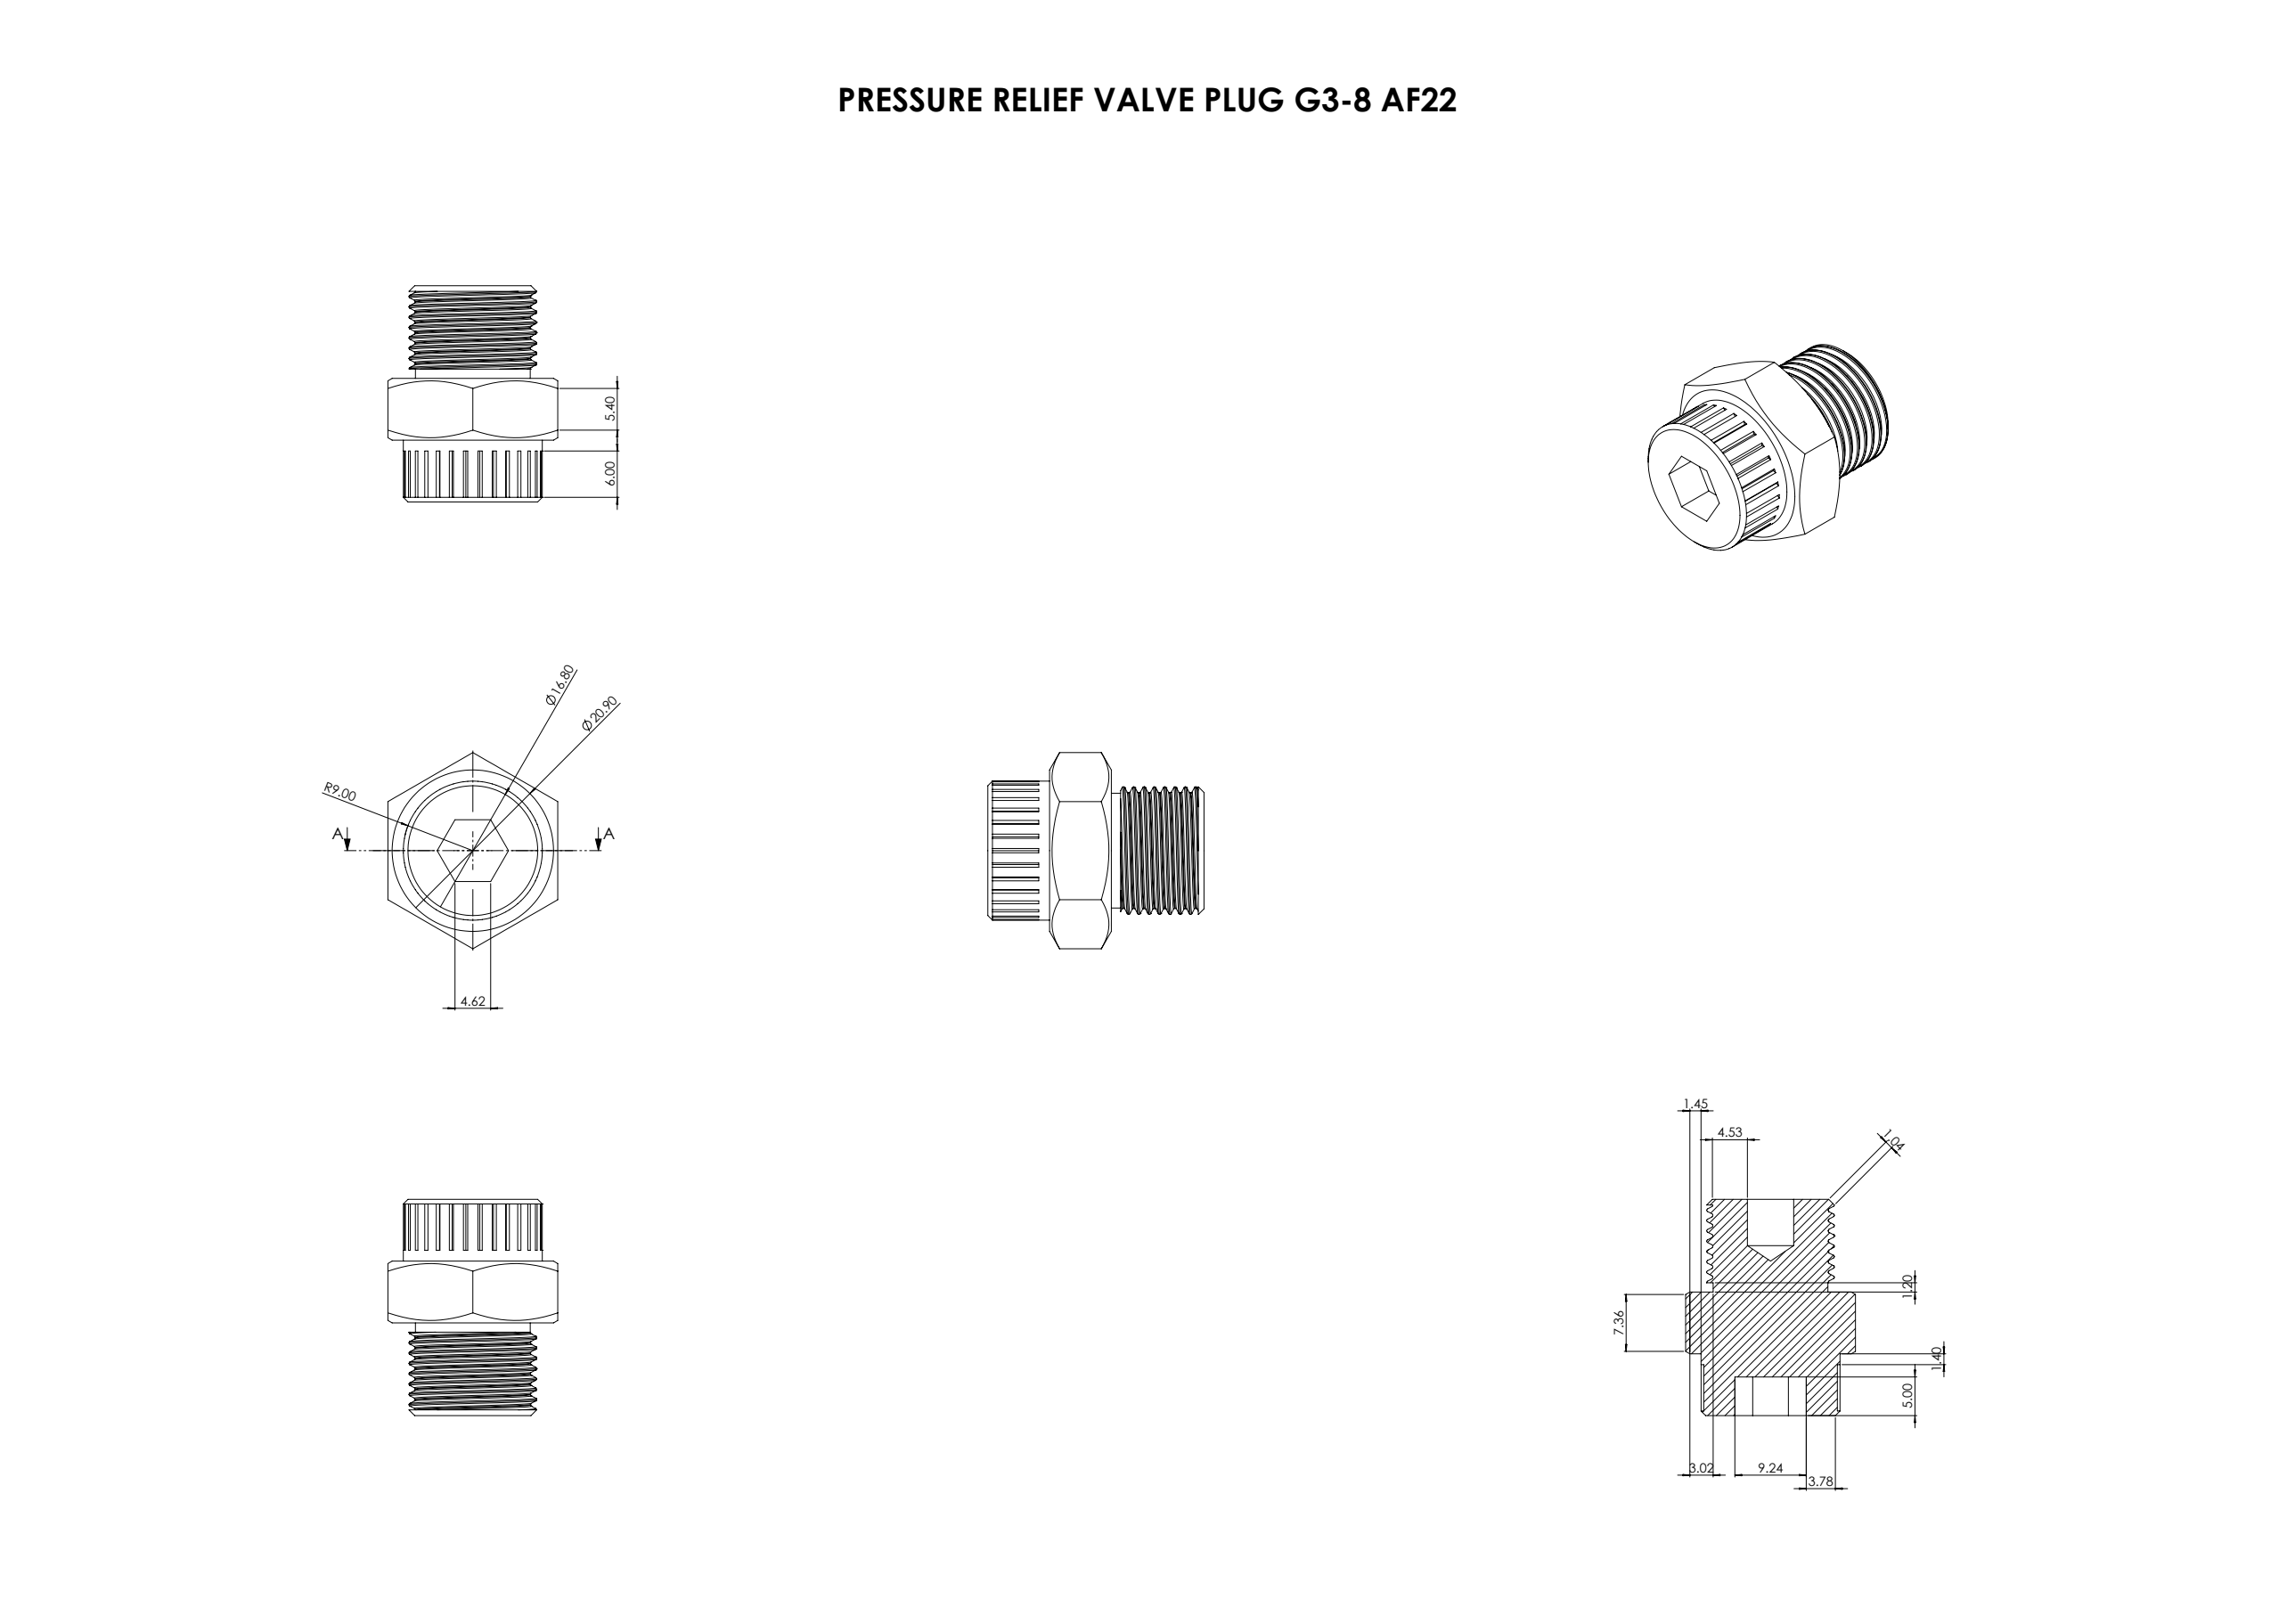
ISO-10303-21;
HEADER;
/* Generated by software containing ST-Developer
 * from STEP Tools, Inc. (www.steptools.com) 
 */

FILE_DESCRIPTION(
/* description */ (''),
/* implementation_level */ '2;1');

FILE_NAME(
/* name */ '18_Pressure_Relief_Valve_Plug_G3-8_AF22.step',
/* time_stamp */ '2026-10-23T00:52:27+05:00',
/* author */ (''),
/* organization */ (''),
/* preprocessor_version */ 'ST-DEVELOPER v20.2',
/* originating_system */ 'Autodesk Translation Framework v15.15.0.0',
/* authorisation */ '');

FILE_SCHEMA (('AUTOMOTIVE_DESIGN { 1 0 10303 214 3 1 1 }'));
ENDSEC;

DATA;
#10=MECHANICAL_DESIGN_GEOMETRIC_PRESENTATION_REPRESENTATION('',(#1554),#59204);
#318=B_SPLINE_SURFACE_WITH_KNOTS('',3,3,((#32590,#32591,#32592,#32593,#32594,
#32595,#32596,#32597,#32598,#32599,#32600,#32601,#32602,#32603,#32604,#32605,
#32606,#32607,#32608,#32609,#32610,#32611,#32612,#32613,#32614,#32615,#32616,
#32617,#32618,#32619,#32620,#32621,#32622,#32623,#32624,#32625,#32626,#32627,
#32628,#32629,#32630,#32631,#32632,#32633,#32634,#32635,#32636,#32637,#32638,
#32639,#32640,#32641,#32642,#32643,#32644,#32645,#32646,#32647,#32648,#32649,
#32650,#32651,#32652,#32653,#32654,#32655,#32656,#32657,#32658,#32659,#32660,
#32661,#32662,#32663,#32664,#32665,#32666,#32667,#32668,#32669,#32670,#32671,
#32672,#32673,#32674,#32675,#32676,#32677,#32678,#32679,#32680,#32681,#32682,
#32683,#32684,#32685,#32686,#32687,#32688,#32689,#32690),(#32691,#32692,
#32693,#32694,#32695,#32696,#32697,#32698,#32699,#32700,#32701,#32702,#32703,
#32704,#32705,#32706,#32707,#32708,#32709,#32710,#32711,#32712,#32713,#32714,
#32715,#32716,#32717,#32718,#32719,#32720,#32721,#32722,#32723,#32724,#32725,
#32726,#32727,#32728,#32729,#32730,#32731,#32732,#32733,#32734,#32735,#32736,
#32737,#32738,#32739,#32740,#32741,#32742,#32743,#32744,#32745,#32746,#32747,
#32748,#32749,#32750,#32751,#32752,#32753,#32754,#32755,#32756,#32757,#32758,
#32759,#32760,#32761,#32762,#32763,#32764,#32765,#32766,#32767,#32768,#32769,
#32770,#32771,#32772,#32773,#32774,#32775,#32776,#32777,#32778,#32779,#32780,
#32781,#32782,#32783,#32784,#32785,#32786,#32787,#32788,#32789,#32790,#32791),
(#32792,#32793,#32794,#32795,#32796,#32797,#32798,#32799,#32800,#32801,
#32802,#32803,#32804,#32805,#32806,#32807,#32808,#32809,#32810,#32811,#32812,
#32813,#32814,#32815,#32816,#32817,#32818,#32819,#32820,#32821,#32822,#32823,
#32824,#32825,#32826,#32827,#32828,#32829,#32830,#32831,#32832,#32833,#32834,
#32835,#32836,#32837,#32838,#32839,#32840,#32841,#32842,#32843,#32844,#32845,
#32846,#32847,#32848,#32849,#32850,#32851,#32852,#32853,#32854,#32855,#32856,
#32857,#32858,#32859,#32860,#32861,#32862,#32863,#32864,#32865,#32866,#32867,
#32868,#32869,#32870,#32871,#32872,#32873,#32874,#32875,#32876,#32877,#32878,
#32879,#32880,#32881,#32882,#32883,#32884,#32885,#32886,#32887,#32888,#32889,
#32890,#32891,#32892),(#32893,#32894,#32895,#32896,#32897,#32898,#32899,
#32900,#32901,#32902,#32903,#32904,#32905,#32906,#32907,#32908,#32909,#32910,
#32911,#32912,#32913,#32914,#32915,#32916,#32917,#32918,#32919,#32920,#32921,
#32922,#32923,#32924,#32925,#32926,#32927,#32928,#32929,#32930,#32931,#32932,
#32933,#32934,#32935,#32936,#32937,#32938,#32939,#32940,#32941,#32942,#32943,
#32944,#32945,#32946,#32947,#32948,#32949,#32950,#32951,#32952,#32953,#32954,
#32955,#32956,#32957,#32958,#32959,#32960,#32961,#32962,#32963,#32964,#32965,
#32966,#32967,#32968,#32969,#32970,#32971,#32972,#32973,#32974,#32975,#32976,
#32977,#32978,#32979,#32980,#32981,#32982,#32983,#32984,#32985,#32986,#32987,
#32988,#32989,#32990,#32991,#32992,#32993),(#32994,#32995,#32996,#32997,
#32998,#32999,#33000,#33001,#33002,#33003,#33004,#33005,#33006,#33007,#33008,
#33009,#33010,#33011,#33012,#33013,#33014,#33015,#33016,#33017,#33018,#33019,
#33020,#33021,#33022,#33023,#33024,#33025,#33026,#33027,#33028,#33029,#33030,
#33031,#33032,#33033,#33034,#33035,#33036,#33037,#33038,#33039,#33040,#33041,
#33042,#33043,#33044,#33045,#33046,#33047,#33048,#33049,#33050,#33051,#33052,
#33053,#33054,#33055,#33056,#33057,#33058,#33059,#33060,#33061,#33062,#33063,
#33064,#33065,#33066,#33067,#33068,#33069,#33070,#33071,#33072,#33073,#33074,
#33075,#33076,#33077,#33078,#33079,#33080,#33081,#33082,#33083,#33084,#33085,
#33086,#33087,#33088,#33089,#33090,#33091,#33092,#33093,#33094)),
 .UNSPECIFIED.,.F.,.F.,.F.,(4,1,4),(4,1,1,1,1,1,1,1,1,1,1,1,1,1,1,1,1,1,
1,1,1,1,1,1,1,1,1,1,1,1,1,1,1,1,1,1,1,1,1,1,1,1,1,1,1,1,1,1,1,1,1,1,1,1,
1,1,1,1,1,1,1,1,1,1,1,1,1,1,1,1,1,1,1,1,1,1,1,1,1,1,1,1,1,1,1,1,1,1,1,1,
1,1,1,1,1,1,1,1,4),(0.,0.467498906784196,1.09083078249646),(6.28318530717956,
6.77358368901884,7.26398207085813,7.75438045269741,8.24477883453669,8.73517721637598,
9.22557559821526,9.71597398005454,10.2063723618938,10.6967707437331,11.1871691255724,
11.6775675074117,12.167965889251,12.6583642710902,13.1487626529295,13.6391610347688,
14.1295594166081,14.6199577984474,15.1103561802867,15.6007545621259,16.0911529439652,
16.5815513258045,17.0719497076438,17.5623480894831,18.0527464713224,18.5431448531616,
19.0335432350009,19.5239416168402,20.0143399986795,20.5047383805188,20.9951367623581,
21.4855351441973,21.9759335260366,22.4663319078759,22.9567302897152,23.4471286715545,
23.9375270533938,24.427925435233,24.9183238170723,25.4087221989116,25.8991205807509,
26.3895189625902,26.8799173444295,27.3703157262687,27.860714108108,28.3511124899473,
28.8415108717866,29.3319092536259,29.8223076354652,30.3127060173044,30.8031043991437,
31.293502780983,31.7839011628223,32.2742995446616,32.7646979265009,33.2550963083402,
33.7454946901794,34.2358930720187,34.726291453858,35.2166898356973,35.7070882175366,
36.1974865993759,36.6878849812151,37.1782833630544,37.6686817448937,38.159080126733,
38.6494785085723,39.1398768904116,39.6302752722508,40.1206736540901,40.6110720359294,
41.1014704177687,41.591868799608,42.0822671814473,42.5726655632865,43.0630639451258,
43.5534623269651,44.0438607088044,44.5342590906437,45.024657472483,45.5150558543222,
46.0054542361615,46.4958526180008,46.9862509998401,47.4766493816794,47.9670477635187,
48.4574461453579,48.9478445271972,49.4382429090365,49.9286412908758,50.4190396727151,
50.9094380545544,51.3998364363936,51.8902348182329,52.3806332000722,52.8710315819115,
53.3614299637508,53.8518283455901,54.3422267274293),.UNSPECIFIED.);
#319=B_SPLINE_SURFACE_WITH_KNOTS('',3,3,((#33507,#33508,#33509,#33510,#33511,
#33512,#33513,#33514,#33515,#33516,#33517,#33518,#33519,#33520,#33521,#33522,
#33523,#33524,#33525,#33526,#33527,#33528,#33529,#33530,#33531,#33532,#33533,
#33534,#33535,#33536,#33537,#33538,#33539,#33540,#33541,#33542,#33543,#33544,
#33545,#33546,#33547,#33548,#33549,#33550,#33551,#33552,#33553,#33554,#33555,
#33556,#33557,#33558,#33559,#33560,#33561,#33562,#33563,#33564,#33565,#33566,
#33567,#33568,#33569,#33570,#33571,#33572,#33573,#33574,#33575,#33576,#33577,
#33578,#33579,#33580,#33581,#33582,#33583,#33584,#33585,#33586,#33587,#33588,
#33589,#33590,#33591,#33592,#33593,#33594,#33595,#33596,#33597,#33598,#33599,
#33600,#33601,#33602,#33603,#33604,#33605,#33606,#33607),(#33608,#33609,
#33610,#33611,#33612,#33613,#33614,#33615,#33616,#33617,#33618,#33619,#33620,
#33621,#33622,#33623,#33624,#33625,#33626,#33627,#33628,#33629,#33630,#33631,
#33632,#33633,#33634,#33635,#33636,#33637,#33638,#33639,#33640,#33641,#33642,
#33643,#33644,#33645,#33646,#33647,#33648,#33649,#33650,#33651,#33652,#33653,
#33654,#33655,#33656,#33657,#33658,#33659,#33660,#33661,#33662,#33663,#33664,
#33665,#33666,#33667,#33668,#33669,#33670,#33671,#33672,#33673,#33674,#33675,
#33676,#33677,#33678,#33679,#33680,#33681,#33682,#33683,#33684,#33685,#33686,
#33687,#33688,#33689,#33690,#33691,#33692,#33693,#33694,#33695,#33696,#33697,
#33698,#33699,#33700,#33701,#33702,#33703,#33704,#33705,#33706,#33707,#33708),
(#33709,#33710,#33711,#33712,#33713,#33714,#33715,#33716,#33717,#33718,
#33719,#33720,#33721,#33722,#33723,#33724,#33725,#33726,#33727,#33728,#33729,
#33730,#33731,#33732,#33733,#33734,#33735,#33736,#33737,#33738,#33739,#33740,
#33741,#33742,#33743,#33744,#33745,#33746,#33747,#33748,#33749,#33750,#33751,
#33752,#33753,#33754,#33755,#33756,#33757,#33758,#33759,#33760,#33761,#33762,
#33763,#33764,#33765,#33766,#33767,#33768,#33769,#33770,#33771,#33772,#33773,
#33774,#33775,#33776,#33777,#33778,#33779,#33780,#33781,#33782,#33783,#33784,
#33785,#33786,#33787,#33788,#33789,#33790,#33791,#33792,#33793,#33794,#33795,
#33796,#33797,#33798,#33799,#33800,#33801,#33802,#33803,#33804,#33805,#33806,
#33807,#33808,#33809),(#33810,#33811,#33812,#33813,#33814,#33815,#33816,
#33817,#33818,#33819,#33820,#33821,#33822,#33823,#33824,#33825,#33826,#33827,
#33828,#33829,#33830,#33831,#33832,#33833,#33834,#33835,#33836,#33837,#33838,
#33839,#33840,#33841,#33842,#33843,#33844,#33845,#33846,#33847,#33848,#33849,
#33850,#33851,#33852,#33853,#33854,#33855,#33856,#33857,#33858,#33859,#33860,
#33861,#33862,#33863,#33864,#33865,#33866,#33867,#33868,#33869,#33870,#33871,
#33872,#33873,#33874,#33875,#33876,#33877,#33878,#33879,#33880,#33881,#33882,
#33883,#33884,#33885,#33886,#33887,#33888,#33889,#33890,#33891,#33892,#33893,
#33894,#33895,#33896,#33897,#33898,#33899,#33900,#33901,#33902,#33903,#33904,
#33905,#33906,#33907,#33908,#33909,#33910)),.UNSPECIFIED.,.F.,.F.,.F.,(4,
4),(4,1,1,1,1,1,1,1,1,1,1,1,1,1,1,1,1,1,1,1,1,1,1,1,1,1,1,1,1,1,1,1,1,1,
1,1,1,1,1,1,1,1,1,1,1,1,1,1,1,1,1,1,1,1,1,1,1,1,1,1,1,1,1,1,1,1,1,1,1,1,
1,1,1,1,1,1,1,1,1,1,1,1,1,1,1,1,1,1,1,1,1,1,1,1,1,1,1,1,4),(0.,0.0671853436149873),
(7.04827039213813,7.54574010072062,8.04320980930311,8.5406795178856,9.03814922646809,
9.53561893505058,10.0330886436331,10.5305583522156,11.0280280607981,11.5254977693805,
12.022967477963,12.5204371865455,13.017906895128,13.5153766037105,14.012846312293,
14.5103160208755,15.007785729458,15.5052554380405,16.002725146623,16.5001948552054,
16.9976645637879,17.4951342723704,17.9926039809529,18.4900736895354,18.9875433981179,
19.4850131067004,19.9824828152829,20.4799525238654,20.9774222324479,21.4748919410303,
21.9723616496128,22.4698313581953,22.9673010667778,23.4647707753603,23.9622404839428,
24.4597101925253,24.9571799011078,25.4546496096903,25.9521193182728,26.4495890268552,
26.9470587354377,27.4445284440202,27.9419981526027,28.4394678611852,28.9369375697677,
29.4344072783502,29.9318769869327,30.4293466955152,30.9268164040977,31.4242861126801,
31.9217558212626,32.4192255298451,32.9166952384276,33.4141649470101,33.9116346555926,
34.4091043641751,34.9065740727576,35.4040437813401,35.9015134899225,36.398983198505,
36.8964529070875,37.39392261567,37.8913923242525,38.388862032835,38.8863317414175,
39.38380145,39.8812711585825,40.378740867165,40.8762105757474,41.3736802843299,
41.8711499929124,42.3686197014949,42.8660894100774,43.3635591186599,43.8610288272424,
44.3584985358249,44.8559682444074,45.3534379529899,45.8509076615723,46.3483773701548,
46.8458470787373,47.3433167873198,47.8407864959023,48.3382562044848,48.8357259130673,
49.3331956216498,49.8306653302323,50.3281350388148,50.8256047473972,51.3230744559797,
51.8205441645622,52.3180138731447,52.8154835817272,53.3129532903097,53.8104229988922,
54.3078927074747,54.8053624160572,55.3028321246397,55.8003018332221),
 .UNSPECIFIED.);
#320=B_SPLINE_SURFACE_WITH_KNOTS('',3,3,((#34113,#34114,#34115,#34116,#34117,
#34118,#34119,#34120,#34121,#34122,#34123,#34124,#34125,#34126,#34127,#34128,
#34129,#34130,#34131,#34132,#34133,#34134,#34135,#34136,#34137,#34138,#34139,
#34140,#34141,#34142,#34143,#34144,#34145,#34146,#34147,#34148,#34149,#34150,
#34151,#34152,#34153,#34154,#34155,#34156,#34157,#34158,#34159,#34160,#34161,
#34162,#34163,#34164,#34165,#34166,#34167,#34168,#34169,#34170,#34171,#34172,
#34173,#34174,#34175,#34176,#34177,#34178,#34179,#34180,#34181,#34182,#34183,
#34184,#34185,#34186,#34187,#34188,#34189,#34190,#34191,#34192,#34193,#34194,
#34195,#34196,#34197,#34198,#34199,#34200,#34201,#34202,#34203,#34204,#34205,
#34206,#34207,#34208,#34209,#34210,#34211,#34212,#34213),(#34214,#34215,
#34216,#34217,#34218,#34219,#34220,#34221,#34222,#34223,#34224,#34225,#34226,
#34227,#34228,#34229,#34230,#34231,#34232,#34233,#34234,#34235,#34236,#34237,
#34238,#34239,#34240,#34241,#34242,#34243,#34244,#34245,#34246,#34247,#34248,
#34249,#34250,#34251,#34252,#34253,#34254,#34255,#34256,#34257,#34258,#34259,
#34260,#34261,#34262,#34263,#34264,#34265,#34266,#34267,#34268,#34269,#34270,
#34271,#34272,#34273,#34274,#34275,#34276,#34277,#34278,#34279,#34280,#34281,
#34282,#34283,#34284,#34285,#34286,#34287,#34288,#34289,#34290,#34291,#34292,
#34293,#34294,#34295,#34296,#34297,#34298,#34299,#34300,#34301,#34302,#34303,
#34304,#34305,#34306,#34307,#34308,#34309,#34310,#34311,#34312,#34313,#34314),
(#34315,#34316,#34317,#34318,#34319,#34320,#34321,#34322,#34323,#34324,
#34325,#34326,#34327,#34328,#34329,#34330,#34331,#34332,#34333,#34334,#34335,
#34336,#34337,#34338,#34339,#34340,#34341,#34342,#34343,#34344,#34345,#34346,
#34347,#34348,#34349,#34350,#34351,#34352,#34353,#34354,#34355,#34356,#34357,
#34358,#34359,#34360,#34361,#34362,#34363,#34364,#34365,#34366,#34367,#34368,
#34369,#34370,#34371,#34372,#34373,#34374,#34375,#34376,#34377,#34378,#34379,
#34380,#34381,#34382,#34383,#34384,#34385,#34386,#34387,#34388,#34389,#34390,
#34391,#34392,#34393,#34394,#34395,#34396,#34397,#34398,#34399,#34400,#34401,
#34402,#34403,#34404,#34405,#34406,#34407,#34408,#34409,#34410,#34411,#34412,
#34413,#34414,#34415),(#34416,#34417,#34418,#34419,#34420,#34421,#34422,
#34423,#34424,#34425,#34426,#34427,#34428,#34429,#34430,#34431,#34432,#34433,
#34434,#34435,#34436,#34437,#34438,#34439,#34440,#34441,#34442,#34443,#34444,
#34445,#34446,#34447,#34448,#34449,#34450,#34451,#34452,#34453,#34454,#34455,
#34456,#34457,#34458,#34459,#34460,#34461,#34462,#34463,#34464,#34465,#34466,
#34467,#34468,#34469,#34470,#34471,#34472,#34473,#34474,#34475,#34476,#34477,
#34478,#34479,#34480,#34481,#34482,#34483,#34484,#34485,#34486,#34487,#34488,
#34489,#34490,#34491,#34492,#34493,#34494,#34495,#34496,#34497,#34498,#34499,
#34500,#34501,#34502,#34503,#34504,#34505,#34506,#34507,#34508,#34509,#34510,
#34511,#34512,#34513,#34514,#34515,#34516),(#34517,#34518,#34519,#34520,
#34521,#34522,#34523,#34524,#34525,#34526,#34527,#34528,#34529,#34530,#34531,
#34532,#34533,#34534,#34535,#34536,#34537,#34538,#34539,#34540,#34541,#34542,
#34543,#34544,#34545,#34546,#34547,#34548,#34549,#34550,#34551,#34552,#34553,
#34554,#34555,#34556,#34557,#34558,#34559,#34560,#34561,#34562,#34563,#34564,
#34565,#34566,#34567,#34568,#34569,#34570,#34571,#34572,#34573,#34574,#34575,
#34576,#34577,#34578,#34579,#34580,#34581,#34582,#34583,#34584,#34585,#34586,
#34587,#34588,#34589,#34590,#34591,#34592,#34593,#34594,#34595,#34596,#34597,
#34598,#34599,#34600,#34601,#34602,#34603,#34604,#34605,#34606,#34607,#34608,
#34609,#34610,#34611,#34612,#34613,#34614,#34615,#34616,#34617)),
 .UNSPECIFIED.,.F.,.F.,.F.,(4,1,4),(4,1,1,1,1,1,1,1,1,1,1,1,1,1,1,1,1,1,
1,1,1,1,1,1,1,1,1,1,1,1,1,1,1,1,1,1,1,1,1,1,1,1,1,1,1,1,1,1,1,1,1,1,1,1,
1,1,1,1,1,1,1,1,1,1,1,1,1,1,1,1,1,1,1,1,1,1,1,1,1,1,1,1,1,1,1,1,1,1,1,1,
1,1,1,1,1,1,1,1,4),(0.,0.467498906784196,1.09083078249646),(8.50634549793094,
8.99674387977022,9.48714226160951,9.97754064344879,10.4679390252881,10.9583374071274,
11.4487357889666,11.9391341708059,12.4295325526452,12.9199309344845,13.4103293163238,
13.9007276981631,14.3911260800023,14.8815244618416,15.3719228436809,15.8623212255202,
16.3527196073595,16.8431179891988,17.333516371038,17.8239147528773,18.3143131347166,
18.8047115165559,19.2951098983952,19.7855082802345,20.2759066620737,20.766305043913,
21.2567034257523,21.7471018075916,22.2375001894309,22.7278985712702,23.2182969531094,
23.7086953349487,24.199093716788,24.6894920986273,25.1798904804666,25.6702888623059,
26.1606872441451,26.6510856259844,27.1414840078237,27.631882389663,28.1222807715023,
28.6126791533416,29.1030775351808,29.5934759170201,30.0838742988594,30.5742726806987,
31.064671062538,31.5550694443773,32.0454678262165,32.5358662080558,33.0262645898951,
33.5166629717344,34.0070613535737,34.497459735413,34.9878581172523,35.4782564990915,
35.9686548809308,36.4590532627701,36.9494516446094,37.4398500264487,37.930248408288,
38.4206467901272,38.9110451719665,39.4014435538058,39.8918419356451,40.3822403174844,
40.8726386993237,41.3630370811629,41.8534354630022,42.3438338448415,42.8342322266808,
43.3246306085201,43.8150289903594,44.3054273721986,44.7958257540379,45.2862241358772,
45.7766225177165,46.2670208995558,46.7574192813951,47.2478176632343,47.7382160450736,
48.2286144269129,48.7190128087522,49.2094111905915,49.6998095724308,50.19020795427,
50.6806063361093,51.1710047179486,51.6614030997879,52.1518014816272,52.6421998634665,
53.1325982453057,53.622996627145,54.1133950089843,54.6037933908236,55.0941917726629,
55.5845901545022,56.0749885363414,56.5653869181807),.UNSPECIFIED.);
#321=B_SPLINE_SURFACE_WITH_KNOTS('',3,3,((#34710,#34711,#34712,#34713,#34714,
#34715,#34716,#34717,#34718,#34719,#34720,#34721,#34722,#34723,#34724,#34725,
#34726,#34727,#34728,#34729,#34730,#34731,#34732,#34733,#34734,#34735,#34736,
#34737,#34738,#34739,#34740,#34741,#34742,#34743,#34744,#34745,#34746,#34747,
#34748,#34749,#34750,#34751,#34752,#34753,#34754,#34755,#34756,#34757,#34758,
#34759,#34760,#34761,#34762,#34763,#34764,#34765,#34766,#34767,#34768,#34769,
#34770,#34771,#34772,#34773,#34774,#34775,#34776,#34777,#34778,#34779,#34780,
#34781,#34782,#34783,#34784,#34785,#34786,#34787,#34788,#34789,#34790,#34791,
#34792,#34793,#34794,#34795,#34796,#34797,#34798,#34799,#34800,#34801,#34802,
#34803,#34804,#34805,#34806,#34807,#34808,#34809,#34810),(#34811,#34812,
#34813,#34814,#34815,#34816,#34817,#34818,#34819,#34820,#34821,#34822,#34823,
#34824,#34825,#34826,#34827,#34828,#34829,#34830,#34831,#34832,#34833,#34834,
#34835,#34836,#34837,#34838,#34839,#34840,#34841,#34842,#34843,#34844,#34845,
#34846,#34847,#34848,#34849,#34850,#34851,#34852,#34853,#34854,#34855,#34856,
#34857,#34858,#34859,#34860,#34861,#34862,#34863,#34864,#34865,#34866,#34867,
#34868,#34869,#34870,#34871,#34872,#34873,#34874,#34875,#34876,#34877,#34878,
#34879,#34880,#34881,#34882,#34883,#34884,#34885,#34886,#34887,#34888,#34889,
#34890,#34891,#34892,#34893,#34894,#34895,#34896,#34897,#34898,#34899,#34900,
#34901,#34902,#34903,#34904,#34905,#34906,#34907,#34908,#34909,#34910,#34911),
(#34912,#34913,#34914,#34915,#34916,#34917,#34918,#34919,#34920,#34921,
#34922,#34923,#34924,#34925,#34926,#34927,#34928,#34929,#34930,#34931,#34932,
#34933,#34934,#34935,#34936,#34937,#34938,#34939,#34940,#34941,#34942,#34943,
#34944,#34945,#34946,#34947,#34948,#34949,#34950,#34951,#34952,#34953,#34954,
#34955,#34956,#34957,#34958,#34959,#34960,#34961,#34962,#34963,#34964,#34965,
#34966,#34967,#34968,#34969,#34970,#34971,#34972,#34973,#34974,#34975,#34976,
#34977,#34978,#34979,#34980,#34981,#34982,#34983,#34984,#34985,#34986,#34987,
#34988,#34989,#34990,#34991,#34992,#34993,#34994,#34995,#34996,#34997,#34998,
#34999,#35000,#35001,#35002,#35003,#35004,#35005,#35006,#35007,#35008,#35009,
#35010,#35011,#35012),(#35013,#35014,#35015,#35016,#35017,#35018,#35019,
#35020,#35021,#35022,#35023,#35024,#35025,#35026,#35027,#35028,#35029,#35030,
#35031,#35032,#35033,#35034,#35035,#35036,#35037,#35038,#35039,#35040,#35041,
#35042,#35043,#35044,#35045,#35046,#35047,#35048,#35049,#35050,#35051,#35052,
#35053,#35054,#35055,#35056,#35057,#35058,#35059,#35060,#35061,#35062,#35063,
#35064,#35065,#35066,#35067,#35068,#35069,#35070,#35071,#35072,#35073,#35074,
#35075,#35076,#35077,#35078,#35079,#35080,#35081,#35082,#35083,#35084,#35085,
#35086,#35087,#35088,#35089,#35090,#35091,#35092,#35093,#35094,#35095,#35096,
#35097,#35098,#35099,#35100,#35101,#35102,#35103,#35104,#35105,#35106,#35107,
#35108,#35109,#35110,#35111,#35112,#35113),(#35114,#35115,#35116,#35117,
#35118,#35119,#35120,#35121,#35122,#35123,#35124,#35125,#35126,#35127,#35128,
#35129,#35130,#35131,#35132,#35133,#35134,#35135,#35136,#35137,#35138,#35139,
#35140,#35141,#35142,#35143,#35144,#35145,#35146,#35147,#35148,#35149,#35150,
#35151,#35152,#35153,#35154,#35155,#35156,#35157,#35158,#35159,#35160,#35161,
#35162,#35163,#35164,#35165,#35166,#35167,#35168,#35169,#35170,#35171,#35172,
#35173,#35174,#35175,#35176,#35177,#35178,#35179,#35180,#35181,#35182,#35183,
#35184,#35185,#35186,#35187,#35188,#35189,#35190,#35191,#35192,#35193,#35194,
#35195,#35196,#35197,#35198,#35199,#35200,#35201,#35202,#35203,#35204,#35205,
#35206,#35207,#35208,#35209,#35210,#35211,#35212,#35213,#35214)),
 .UNSPECIFIED.,.F.,.F.,.F.,(4,1,4),(4,1,1,1,1,1,1,1,1,1,1,1,1,1,1,1,1,1,
1,1,1,1,1,1,1,1,1,1,1,1,1,1,1,1,1,1,1,1,1,1,1,1,1,1,1,1,1,1,1,1,1,1,1,1,
1,1,1,1,1,1,1,1,1,1,1,1,1,1,1,1,1,1,1,1,1,1,1,1,1,1,1,1,1,1,1,1,1,1,1,1,
1,1,1,1,1,1,1,1,4),(-1.09083078249646,-0.623331875712262,0.),(9.57812533864918,
10.0685237204885,10.5589221023278,11.049320484167,11.5397188660063,12.0301172478456,
12.5205156296849,13.0109140115242,13.5013123933635,13.9917107752027,14.482109157042,
14.9725075388813,15.4629059207206,15.9533043025599,16.4437026843992,16.9341010662384,
17.4244994480777,17.914897829917,18.4052962117563,18.8956945935956,19.3860929754349,
19.8764913572741,20.3668897391134,20.8572881209527,21.347686502792,21.8380848846313,
22.3284832664706,22.8188816483098,23.3092800301491,23.7996784119884,24.2900767938277,
24.780475175667,25.2708735575063,25.7612719393455,26.2516703211848,26.7420687030241,
27.2324670848634,27.7228654667027,28.213263848542,28.7036622303812,29.1940606122205,
29.6844589940598,30.1748573758991,30.6652557577384,31.1556541395777,31.6460525214169,
32.1364509032562,32.6268492850955,33.1172476669348,33.6076460487741,34.0980444306134,
34.5884428124526,35.0788411942919,35.5692395761312,36.0596379579705,36.5500363398098,
37.0404347216491,37.5308331034883,38.0212314853276,38.5116298671669,39.0020282490062,
39.4924266308455,39.9828250126848,40.473223394524,40.9636217763633,41.4540201582026,
41.9444185400419,42.4348169218812,42.9252153037205,43.4156136855597,43.906012067399,
44.3964104492383,44.8868088310776,45.3772072129169,45.8676055947562,46.3580039765954,
46.8484023584347,47.338800740274,47.8291991221133,48.3195975039526,48.8099958857919,
49.3003942676311,49.7907926494704,50.2811910313097,50.771589413149,51.2619877949883,
51.7523861768276,52.2427845586669,52.7331829405061,53.2235813223454,53.7139797041847,
54.204378086024,54.6947764678633,55.1851748497025,55.6755732315418,56.1659716133811,
56.6563699952204,57.1467683770597,57.637166758899),.UNSPECIFIED.);
#322=B_SPLINE_SURFACE_WITH_KNOTS('',3,3,((#35322,#35323,#35324,#35325,#35326,
#35327,#35328,#35329,#35330,#35331,#35332,#35333,#35334,#35335,#35336,#35337,
#35338,#35339,#35340,#35341,#35342,#35343,#35344,#35345,#35346,#35347,#35348,
#35349,#35350,#35351,#35352,#35353,#35354,#35355,#35356,#35357,#35358,#35359,
#35360,#35361,#35362,#35363,#35364,#35365,#35366,#35367,#35368,#35369,#35370,
#35371,#35372,#35373,#35374,#35375,#35376,#35377,#35378,#35379,#35380,#35381,
#35382,#35383,#35384,#35385,#35386,#35387,#35388,#35389,#35390,#35391,#35392,
#35393,#35394,#35395,#35396,#35397,#35398,#35399,#35400,#35401,#35402,#35403,
#35404,#35405,#35406,#35407,#35408,#35409,#35410,#35411,#35412,#35413,#35414,
#35415,#35416,#35417,#35418,#35419,#35420,#35421,#35422),(#35423,#35424,
#35425,#35426,#35427,#35428,#35429,#35430,#35431,#35432,#35433,#35434,#35435,
#35436,#35437,#35438,#35439,#35440,#35441,#35442,#35443,#35444,#35445,#35446,
#35447,#35448,#35449,#35450,#35451,#35452,#35453,#35454,#35455,#35456,#35457,
#35458,#35459,#35460,#35461,#35462,#35463,#35464,#35465,#35466,#35467,#35468,
#35469,#35470,#35471,#35472,#35473,#35474,#35475,#35476,#35477,#35478,#35479,
#35480,#35481,#35482,#35483,#35484,#35485,#35486,#35487,#35488,#35489,#35490,
#35491,#35492,#35493,#35494,#35495,#35496,#35497,#35498,#35499,#35500,#35501,
#35502,#35503,#35504,#35505,#35506,#35507,#35508,#35509,#35510,#35511,#35512,
#35513,#35514,#35515,#35516,#35517,#35518,#35519,#35520,#35521,#35522,#35523),
(#35524,#35525,#35526,#35527,#35528,#35529,#35530,#35531,#35532,#35533,
#35534,#35535,#35536,#35537,#35538,#35539,#35540,#35541,#35542,#35543,#35544,
#35545,#35546,#35547,#35548,#35549,#35550,#35551,#35552,#35553,#35554,#35555,
#35556,#35557,#35558,#35559,#35560,#35561,#35562,#35563,#35564,#35565,#35566,
#35567,#35568,#35569,#35570,#35571,#35572,#35573,#35574,#35575,#35576,#35577,
#35578,#35579,#35580,#35581,#35582,#35583,#35584,#35585,#35586,#35587,#35588,
#35589,#35590,#35591,#35592,#35593,#35594,#35595,#35596,#35597,#35598,#35599,
#35600,#35601,#35602,#35603,#35604,#35605,#35606,#35607,#35608,#35609,#35610,
#35611,#35612,#35613,#35614,#35615,#35616,#35617,#35618,#35619,#35620,#35621,
#35622,#35623,#35624),(#35625,#35626,#35627,#35628,#35629,#35630,#35631,
#35632,#35633,#35634,#35635,#35636,#35637,#35638,#35639,#35640,#35641,#35642,
#35643,#35644,#35645,#35646,#35647,#35648,#35649,#35650,#35651,#35652,#35653,
#35654,#35655,#35656,#35657,#35658,#35659,#35660,#35661,#35662,#35663,#35664,
#35665,#35666,#35667,#35668,#35669,#35670,#35671,#35672,#35673,#35674,#35675,
#35676,#35677,#35678,#35679,#35680,#35681,#35682,#35683,#35684,#35685,#35686,
#35687,#35688,#35689,#35690,#35691,#35692,#35693,#35694,#35695,#35696,#35697,
#35698,#35699,#35700,#35701,#35702,#35703,#35704,#35705,#35706,#35707,#35708,
#35709,#35710,#35711,#35712,#35713,#35714,#35715,#35716,#35717,#35718,#35719,
#35720,#35721,#35722,#35723,#35724,#35725)),.UNSPECIFIED.,.F.,.F.,.F.,(4,
4),(4,1,1,1,1,1,1,1,1,1,1,1,1,1,1,1,1,1,1,1,1,1,1,1,1,1,1,1,1,1,1,1,1,1,
1,1,1,1,1,1,1,1,1,1,1,1,1,1,1,1,1,1,1,1,1,1,1,1,1,1,1,1,1,1,1,1,1,1,1,1,
1,1,1,1,1,1,1,1,1,1,1,1,1,1,1,1,1,1,1,1,1,1,1,1,1,1,1,1,4),(0.,0.0671853436149873),
(10.3432104236078,10.8406801321902,11.3381498407727,11.8356195493552,12.3330892579377,
12.8305589665202,13.3280286751027,13.8254983836852,14.3229680922677,14.8204378008502,
15.3179075094327,15.8153772180151,16.3128469265976,16.8103166351801,17.3077863437626,
17.8052560523451,18.3027257609276,18.8001954695101,19.2976651780926,19.7951348866751,
20.2926045952576,20.79007430384,21.2875440124225,21.785013721005,22.2824834295875,
22.77995313817,23.2774228467525,23.774892555335,24.2723622639175,24.7698319725,
25.2673016810825,25.7647713896649,26.2622410982474,26.7597108068299,27.2571805154124,
27.7546502239949,28.2521199325774,28.7495896411599,29.2470593497424,29.7445290583249,
30.2419987669074,30.7394684754899,31.2369381840723,31.7344078926548,32.2318776012373,
32.7293473098198,33.2268170184023,33.7242867269848,34.2217564355673,34.7192261441498,
35.2166958527323,35.7141655613148,36.2116352698972,36.7091049784797,37.2065746870622,
37.7040443956447,38.2015141042272,38.6989838128097,39.1964535213922,39.6939232299747,
40.1913929385572,40.6888626471397,41.1863323557221,41.6838020643046,42.1812717728871,
42.6787414814696,43.1762111900521,43.6736808986346,44.1711506072171,44.6686203157996,
45.1660900243821,45.6635597329645,46.161029441547,46.6584991501295,47.155968858712,
47.6534385672945,48.150908275877,48.6483779844595,49.145847693042,49.6433174016245,
50.140787110207,50.6382568187894,51.1357265273719,51.6331962359544,52.1306659445369,
52.6281356531194,53.1256053617019,53.6230750702844,54.1205447788669,54.6180144874494,
55.1154841960319,55.6129539046143,56.1104236131968,56.6078933217793,57.1053630303618,
57.6028327389443,58.1003024475268,58.5977721561093,59.0952418646918),
 .UNSPECIFIED.);
#323=B_SPLINE_SURFACE_WITH_KNOTS('',3,3,((#35878,#35879,#35880,#35881,#35882,
#35883,#35884,#35885,#35886,#35887,#35888,#35889,#35890,#35891,#35892,#35893,
#35894,#35895,#35896,#35897,#35898,#35899,#35900,#35901,#35902,#35903,#35904,
#35905,#35906,#35907,#35908,#35909,#35910,#35911,#35912,#35913,#35914,#35915,
#35916,#35917,#35918,#35919,#35920,#35921,#35922,#35923,#35924,#35925,#35926,
#35927,#35928,#35929,#35930,#35931,#35932,#35933,#35934,#35935,#35936,#35937,
#35938,#35939,#35940,#35941,#35942,#35943,#35944,#35945,#35946,#35947,#35948,
#35949,#35950,#35951,#35952,#35953,#35954,#35955,#35956,#35957,#35958,#35959,
#35960,#35961,#35962,#35963,#35964,#35965,#35966,#35967,#35968,#35969,#35970,
#35971,#35972,#35973,#35974,#35975,#35976,#35977,#35978),(#35979,#35980,
#35981,#35982,#35983,#35984,#35985,#35986,#35987,#35988,#35989,#35990,#35991,
#35992,#35993,#35994,#35995,#35996,#35997,#35998,#35999,#36000,#36001,#36002,
#36003,#36004,#36005,#36006,#36007,#36008,#36009,#36010,#36011,#36012,#36013,
#36014,#36015,#36016,#36017,#36018,#36019,#36020,#36021,#36022,#36023,#36024,
#36025,#36026,#36027,#36028,#36029,#36030,#36031,#36032,#36033,#36034,#36035,
#36036,#36037,#36038,#36039,#36040,#36041,#36042,#36043,#36044,#36045,#36046,
#36047,#36048,#36049,#36050,#36051,#36052,#36053,#36054,#36055,#36056,#36057,
#36058,#36059,#36060,#36061,#36062,#36063,#36064,#36065,#36066,#36067,#36068,
#36069,#36070,#36071,#36072,#36073,#36074,#36075,#36076,#36077,#36078,#36079),
(#36080,#36081,#36082,#36083,#36084,#36085,#36086,#36087,#36088,#36089,
#36090,#36091,#36092,#36093,#36094,#36095,#36096,#36097,#36098,#36099,#36100,
#36101,#36102,#36103,#36104,#36105,#36106,#36107,#36108,#36109,#36110,#36111,
#36112,#36113,#36114,#36115,#36116,#36117,#36118,#36119,#36120,#36121,#36122,
#36123,#36124,#36125,#36126,#36127,#36128,#36129,#36130,#36131,#36132,#36133,
#36134,#36135,#36136,#36137,#36138,#36139,#36140,#36141,#36142,#36143,#36144,
#36145,#36146,#36147,#36148,#36149,#36150,#36151,#36152,#36153,#36154,#36155,
#36156,#36157,#36158,#36159,#36160,#36161,#36162,#36163,#36164,#36165,#36166,
#36167,#36168,#36169,#36170,#36171,#36172,#36173,#36174,#36175,#36176,#36177,
#36178,#36179,#36180),(#36181,#36182,#36183,#36184,#36185,#36186,#36187,
#36188,#36189,#36190,#36191,#36192,#36193,#36194,#36195,#36196,#36197,#36198,
#36199,#36200,#36201,#36202,#36203,#36204,#36205,#36206,#36207,#36208,#36209,
#36210,#36211,#36212,#36213,#36214,#36215,#36216,#36217,#36218,#36219,#36220,
#36221,#36222,#36223,#36224,#36225,#36226,#36227,#36228,#36229,#36230,#36231,
#36232,#36233,#36234,#36235,#36236,#36237,#36238,#36239,#36240,#36241,#36242,
#36243,#36244,#36245,#36246,#36247,#36248,#36249,#36250,#36251,#36252,#36253,
#36254,#36255,#36256,#36257,#36258,#36259,#36260,#36261,#36262,#36263,#36264,
#36265,#36266,#36267,#36268,#36269,#36270,#36271,#36272,#36273,#36274,#36275,
#36276,#36277,#36278,#36279,#36280,#36281),(#36282,#36283,#36284,#36285,
#36286,#36287,#36288,#36289,#36290,#36291,#36292,#36293,#36294,#36295,#36296,
#36297,#36298,#36299,#36300,#36301,#36302,#36303,#36304,#36305,#36306,#36307,
#36308,#36309,#36310,#36311,#36312,#36313,#36314,#36315,#36316,#36317,#36318,
#36319,#36320,#36321,#36322,#36323,#36324,#36325,#36326,#36327,#36328,#36329,
#36330,#36331,#36332,#36333,#36334,#36335,#36336,#36337,#36338,#36339,#36340,
#36341,#36342,#36343,#36344,#36345,#36346,#36347,#36348,#36349,#36350,#36351,
#36352,#36353,#36354,#36355,#36356,#36357,#36358,#36359,#36360,#36361,#36362,
#36363,#36364,#36365,#36366,#36367,#36368,#36369,#36370,#36371,#36372,#36373,
#36374,#36375,#36376,#36377,#36378,#36379,#36380,#36381,#36382)),
 .UNSPECIFIED.,.F.,.F.,.F.,(4,1,4),(4,1,1,1,1,1,1,1,1,1,1,1,1,1,1,1,1,1,
1,1,1,1,1,1,1,1,1,1,1,1,1,1,1,1,1,1,1,1,1,1,1,1,1,1,1,1,1,1,1,1,1,1,1,1,
1,1,1,1,1,1,1,1,1,1,1,1,1,1,1,1,1,1,1,1,1,1,1,1,1,1,1,1,1,1,1,1,1,1,1,1,
1,1,1,1,1,1,1,1,4),(-1.09083078249646,-0.623331875712262,0.),(11.8012855294006,
12.2916839112399,12.7820822930791,13.2724806749184,13.7628790567577,14.253277438597,
14.7436758204363,15.2340742022756,15.7244725841148,16.2148709659541,16.7052693477934,
17.1956677296327,17.686066111472,18.1764644933113,18.6668628751505,19.1572612569898,
19.6476596388291,20.1380580206684,20.6284564025077,21.118854784347,21.6092531661862,
22.0996515480255,22.5900499298648,23.0804483117041,23.5708466935434,24.0612450753827,
24.5516434572219,25.0420418390612,25.5324402209005,26.0228386027398,26.5132369845791,
27.0036353664184,27.4940337482576,27.9844321300969,28.4748305119362,28.9652288937755,
29.4556272756148,29.9460256574541,30.4364240392933,30.9268224211326,31.4172208029719,
31.9076191848112,32.3980175666505,32.8884159484898,33.378814330329,33.8692127121683,
34.3596110940076,34.8500094758469,35.3404078576862,35.8308062395255,36.3212046213647,
36.811603003204,37.3020013850433,37.7923997668826,38.2827981487219,38.7731965305612,
39.2635949124004,39.7539932942397,40.244391676079,40.7347900579183,41.2251884397576,
41.7155868215969,42.2059852034361,42.6963835852754,43.1867819671147,43.677180348954,
44.1675787307933,44.6579771126326,45.1483754944718,45.6387738763111,46.1291722581504,
46.6195706399897,47.109969021829,47.6003674036683,48.0907657855076,48.5811641673468,
49.0715625491861,49.5619609310254,50.0523593128647,50.542757694704,51.0331560765432,
51.5235544583825,52.0139528402218,52.5043512220611,52.9947496039004,53.4851479857397,
53.975546367579,54.4659447494182,54.9563431312575,55.4467415130968,55.9371398949361,
56.4275382767754,56.9179366586147,57.4083350404539,57.8987334222932,58.3891318041325,
58.8795301859718,59.3699285678111,59.8603269496504),.UNSPECIFIED.);
#581=B_SPLINE_CURVE_WITH_KNOTS('',3,(#32302,#32303,#32304,#32305,#32306,
#32307,#32308,#32309,#32310,#32311,#32312),.UNSPECIFIED.,.F.,.F.,(4,1,1,
1,1,1,1,1,4),(53.4070751110265,53.7139797041847,54.204378086024,54.6947764678633,
55.1851748497025,55.6755732315418,56.1659716133811,56.6563699952204,56.8720816739404),
 .UNSPECIFIED.);
#582=B_SPLINE_CURVE_WITH_KNOTS('',3,(#32315,#32316,#32317,#32318,#32319,
#32320,#32321,#32322,#32323,#32324),.UNSPECIFIED.,.F.,.F.,(4,1,1,1,1,1,
1,4),(53.4070751110265,53.622996627145,54.1133950089843,54.6037933908236,
55.0941917726629,55.5845901545022,56.0749885363414,56.5653869181807),
 .UNSPECIFIED.);
#583=B_SPLINE_CURVE_WITH_KNOTS('',3,(#32329,#32330,#32331,#32332,#32333,
#32334,#32335,#32336,#32337,#32338,#32339,#32340,#32341,#32342,#32343,#32344,
#32345),.UNSPECIFIED.,.F.,.F.,(4,1,1,1,1,1,1,1,1,1,1,1,1,1,4),(47.1238898038469,
47.338800740274,47.8291991221133,48.3195975039526,48.8099958857919,49.3003942676311,
49.7907926494704,50.2811910313097,50.771589413149,51.2619877949883,51.7523861768276,
52.2427845586669,52.7331829405061,53.2235813223454,53.4070751110265),
 .UNSPECIFIED.);
#584=B_SPLINE_CURVE_WITH_KNOTS('',3,(#32346,#32347,#32348,#32349,#32350,
#32351,#32352,#32353,#32354,#32355,#32356,#32357,#32358,#32359,#32360,#32361,
#32362),.UNSPECIFIED.,.F.,.F.,(4,1,1,1,1,1,1,1,1,1,1,1,1,1,4),(47.1238898038469,
47.2478176632343,47.7382160450736,48.2286144269129,48.7190128087522,49.2094111905915,
49.6998095724308,50.19020795427,50.6806063361093,51.1710047179486,51.6614030997879,
52.1518014816272,52.6421998634665,53.1325982453057,53.4070751110265),
 .UNSPECIFIED.);
#585=B_SPLINE_CURVE_WITH_KNOTS('',3,(#32367,#32368,#32369,#32370,#32371,
#32372,#32373,#32374,#32375,#32376,#32377,#32378,#32379,#32380,#32381,#32382,
#32383),.UNSPECIFIED.,.F.,.F.,(4,1,1,1,1,1,1,1,1,1,1,1,1,1,4),(40.8407044966673,
40.9636217763633,41.4540201582026,41.9444185400419,42.4348169218812,42.9252153037205,
43.4156136855597,43.906012067399,44.3964104492383,44.8868088310776,45.3772072129169,
45.8676055947562,46.3580039765954,46.8484023584347,47.1238898038469),
 .UNSPECIFIED.);
#586=B_SPLINE_CURVE_WITH_KNOTS('',3,(#32384,#32385,#32386,#32387,#32388,
#32389,#32390,#32391,#32392,#32393,#32394,#32395,#32396,#32397,#32398,#32399,
#32400),.UNSPECIFIED.,.F.,.F.,(4,1,1,1,1,1,1,1,1,1,1,1,1,1,4),(40.8407044966673,
40.8726386993237,41.3630370811629,41.8534354630022,42.3438338448415,42.8342322266808,
43.3246306085201,43.8150289903594,44.3054273721986,44.7958257540379,45.2862241358772,
45.7766225177165,46.2670208995558,46.7574192813951,47.1238898038469),
 .UNSPECIFIED.);
#587=B_SPLINE_CURVE_WITH_KNOTS('',3,(#32405,#32406,#32407,#32408,#32409,
#32410,#32411,#32412,#32413,#32414,#32415,#32416,#32417,#32418,#32419,#32420,
#32421),.UNSPECIFIED.,.F.,.F.,(4,1,1,1,1,1,1,1,1,1,1,1,1,1,4),(34.5575191894877,
34.5884428124526,35.0788411942919,35.5692395761312,36.0596379579705,36.5500363398098,
37.0404347216491,37.5308331034883,38.0212314853276,38.5116298671669,39.0020282490062,
39.4924266308455,39.9828250126848,40.473223394524,40.8407044966673),
 .UNSPECIFIED.);
#588=B_SPLINE_CURVE_WITH_KNOTS('',3,(#32422,#32423,#32424,#32425,#32426,
#32427,#32428,#32429,#32430,#32431,#32432,#32433,#32434,#32435,#32436,#32437),
 .UNSPECIFIED.,.F.,.F.,(4,1,1,1,1,1,1,1,1,1,1,1,1,4),(34.5575191894877,
34.9878581172523,35.4782564990915,35.9686548809308,36.4590532627701,36.9494516446094,
37.4398500264487,37.930248408288,38.4206467901272,38.9110451719665,39.4014435538058,
39.8918419356451,40.3822403174844,40.8407044966673),.UNSPECIFIED.);
#589=B_SPLINE_CURVE_WITH_KNOTS('',3,(#32442,#32443,#32444,#32445,#32446,
#32447,#32448,#32449,#32450,#32451,#32452,#32453,#32454,#32455,#32456,#32457),
 .UNSPECIFIED.,.F.,.F.,(4,1,1,1,1,1,1,1,1,1,1,1,1,4),(28.2743338823081,
28.7036622303812,29.1940606122205,29.6844589940598,30.1748573758991,30.6652557577384,
31.1556541395777,31.6460525214169,32.1364509032562,32.6268492850955,33.1172476669348,
33.6076460487741,34.0980444306134,34.5575191894877),.UNSPECIFIED.);
#590=B_SPLINE_CURVE_WITH_KNOTS('',3,(#32458,#32459,#32460,#32461,#32462,
#32463,#32464,#32465,#32466,#32467,#32468,#32469,#32470,#32471,#32472,#32473,
#32474),.UNSPECIFIED.,.F.,.F.,(4,1,1,1,1,1,1,1,1,1,1,1,1,1,4),(28.2743338823081,
28.6126791533416,29.1030775351808,29.5934759170201,30.0838742988594,30.5742726806987,
31.064671062538,31.5550694443773,32.0454678262165,32.5358662080558,33.0262645898951,
33.5166629717344,34.0070613535737,34.497459735413,34.5575191894877),
 .UNSPECIFIED.);
#591=B_SPLINE_CURVE_WITH_KNOTS('',3,(#32479,#32480,#32481,#32482,#32483,
#32484,#32485,#32486,#32487,#32488,#32489,#32490,#32491,#32492,#32493,#32494,
#32495),.UNSPECIFIED.,.F.,.F.,(4,1,1,1,1,1,1,1,1,1,1,1,1,1,4),(21.9911485751285,
22.3284832664706,22.8188816483098,23.3092800301491,23.7996784119884,24.2900767938277,
24.780475175667,25.2708735575063,25.7612719393455,26.2516703211848,26.7420687030241,
27.2324670848634,27.7228654667027,28.213263848542,28.2743338823081),
 .UNSPECIFIED.);
#592=B_SPLINE_CURVE_WITH_KNOTS('',3,(#32496,#32497,#32498,#32499,#32500,
#32501,#32502,#32503,#32504,#32505,#32506,#32507,#32508,#32509,#32510,#32511,
#32512),.UNSPECIFIED.,.F.,.F.,(4,1,1,1,1,1,1,1,1,1,1,1,1,1,4),(21.9911485751285,
22.2375001894309,22.7278985712702,23.2182969531094,23.7086953349487,24.199093716788,
24.6894920986273,25.1798904804666,25.6702888623059,26.1606872441451,26.6510856259844,
27.1414840078237,27.631882389663,28.1222807715023,28.2743338823081),
 .UNSPECIFIED.);
#593=B_SPLINE_CURVE_WITH_KNOTS('',3,(#32517,#32518,#32519,#32520,#32521,
#32522,#32523,#32524,#32525,#32526,#32527,#32528,#32529,#32530,#32531,#32532,
#32533),.UNSPECIFIED.,.F.,.F.,(4,1,1,1,1,1,1,1,1,1,1,1,1,1,4),(15.7079632679489,
15.9533043025599,16.4437026843992,16.9341010662384,17.4244994480777,17.914897829917,
18.4052962117563,18.8956945935956,19.3860929754349,19.8764913572741,20.3668897391134,
20.8572881209527,21.347686502792,21.8380848846313,21.9911485751285),
 .UNSPECIFIED.);
#594=B_SPLINE_CURVE_WITH_KNOTS('',3,(#32534,#32535,#32536,#32537,#32538,
#32539,#32540,#32541,#32542,#32543,#32544,#32545,#32546,#32547,#32548,#32549,
#32550),.UNSPECIFIED.,.F.,.F.,(4,1,1,1,1,1,1,1,1,1,1,1,1,1,4),(15.7079632679489,
15.8623212255202,16.3527196073595,16.8431179891988,17.333516371038,17.8239147528773,
18.3143131347166,18.8047115165559,19.2951098983952,19.7855082802345,20.2759066620737,
20.766305043913,21.2567034257523,21.7471018075916,21.9911485751285),
 .UNSPECIFIED.);
#595=B_SPLINE_CURVE_WITH_KNOTS('',3,(#32557,#32558,#32559,#32560,#32561,
#32562,#32563,#32564,#32565,#32566,#32567,#32568,#32569,#32570,#32571,#32572),
 .UNSPECIFIED.,.F.,.F.,(4,1,1,1,1,1,1,1,1,1,1,1,1,4),(9.57812533864918,
10.0685237204885,10.5589221023278,11.049320484167,11.5397188660063,12.0301172478456,
12.5205156296849,13.0109140115242,13.5013123933635,13.9917107752027,14.482109157042,
14.9725075388813,15.4629059207206,15.7079632679489),.UNSPECIFIED.);
#596=B_SPLINE_CURVE_WITH_KNOTS('',3,(#32573,#32574,#32575,#32576,#32577,
#32578,#32579,#32580,#32581,#32582,#32583,#32584,#32585,#32586,#32587,#32588,
#32589),.UNSPECIFIED.,.F.,.F.,(4,1,1,1,1,1,1,1,1,1,1,1,1,1,4),(9.42477796076936,
9.48714226160951,9.97754064344879,10.4679390252881,10.9583374071274,11.4487357889666,
11.9391341708059,12.4295325526452,12.9199309344845,13.4103293163238,13.9007276981631,
14.3911260800023,14.8815244618416,15.3719228436809,15.7079632679489),
 .UNSPECIFIED.);
#597=B_SPLINE_CURVE_WITH_KNOTS('',3,(#33097,#33098,#33099,#33100,#33101,
#33102,#33103,#33104),.UNSPECIFIED.,.F.,.F.,(4,2,2,4),(0.,0.303392014531492,
0.493985861454512,0.655896371978029),.UNSPECIFIED.);
#598=B_SPLINE_CURVE_WITH_KNOTS('',3,(#33106,#33107,#33108,#33109,#33110,
#33111,#33112,#33113,#33114,#33115,#33116,#33117,#33118,#33119,#33120,#33121,
#33122,#33123,#33124,#33125,#33126,#33127,#33128,#33129,#33130,#33131,#33132,
#33133,#33134,#33135,#33136,#33137,#33138,#33139,#33140,#33141,#33142,#33143,
#33144,#33145,#33146,#33147,#33148,#33149,#33150,#33151,#33152,#33153,#33154,
#33155,#33156,#33157,#33158,#33159,#33160,#33161,#33162,#33163,#33164,#33165,
#33166,#33167,#33168,#33169,#33170,#33171,#33172,#33173,#33174,#33175,#33176,
#33177,#33178,#33179,#33180,#33181,#33182,#33183,#33184,#33185,#33186,#33187,
#33188,#33189,#33190,#33191,#33192,#33193,#33194,#33195,#33196,#33197,#33198,
#33199,#33200,#33201,#33202,#33203,#33204,#33205,#33206,#33207,#33208,#33209,
#33210,#33211,#33212,#33213,#33214,#33215,#33216,#33217,#33218,#33219,#33220,
#33221,#33222,#33223,#33224,#33225,#33226,#33227,#33228,#33229,#33230,#33231,
#33232,#33233,#33234,#33235,#33236,#33237,#33238,#33239,#33240,#33241,#33242,
#33243,#33244,#33245,#33246,#33247,#33248,#33249,#33250,#33251,#33252,#33253,
#33254,#33255,#33256,#33257,#33258,#33259,#33260,#33261,#33262,#33263,#33264,
#33265,#33266,#33267,#33268,#33269,#33270,#33271,#33272,#33273,#33274,#33275,
#33276,#33277,#33278,#33279,#33280,#33281,#33282,#33283,#33284,#33285,#33286,
#33287,#33288,#33289,#33290,#33291,#33292,#33293,#33294,#33295,#33296,#33297,
#33298,#33299,#33300,#33301,#33302,#33303,#33304,#33305,#33306,#33307,#33308,
#33309,#33310,#33311,#33312,#33313,#33314,#33315,#33316,#33317,#33318,#33319,
#33320,#33321,#33322,#33323,#33324,#33325,#33326,#33327,#33328,#33329,#33330,
#33331,#33332,#33333,#33334,#33335,#33336,#33337,#33338,#33339,#33340,#33341,
#33342,#33343,#33344,#33345,#33346,#33347,#33348,#33349,#33350,#33351,#33352,
#33353,#33354,#33355,#33356,#33357,#33358,#33359,#33360,#33361,#33362,#33363,
#33364,#33365,#33366,#33367,#33368,#33369,#33370,#33371,#33372,#33373,#33374,
#33375,#33376,#33377,#33378,#33379,#33380,#33381,#33382,#33383,#33384,#33385,
#33386,#33387,#33388,#33389,#33390,#33391,#33392,#33393,#33394,#33395,#33396,
#33397),.UNSPECIFIED.,.F.,.F.,(4,3,3,3,3,3,3,3,3,3,3,3,3,3,3,3,3,3,3,3,
3,3,3,3,3,3,3,3,3,3,3,3,3,3,3,3,3,3,3,3,3,3,3,3,3,3,3,3,3,3,3,3,3,3,3,3,
3,3,3,3,3,3,3,3,3,3,3,3,3,3,3,3,3,3,3,3,3,3,3,3,3,3,3,3,3,3,3,3,3,3,3,3,
3,3,3,3,3,4),(0.,0.490398381839284,0.980796763678568,1.47119514551785,1.96159352735713,
2.45199190919642,2.9423902910357,3.43278867287498,3.92318705471427,4.41358543655355,
4.90398381839284,5.39438220023212,5.8847805820714,6.37517896391069,6.86557734574997,
7.35597572758925,7.84637410942854,8.33677249126782,8.8271708731071,9.31756925494639,
9.80796763678567,10.298366018625,10.7887644004642,11.2791627823035,11.7695611641428,
12.2599595459821,12.7503579278214,13.2407563096607,13.7311546914999,14.2215530733392,
14.7119514551785,15.2023498370178,15.6927482188571,16.1831466006964,16.6735449825356,
17.1639433643749,17.6543417462142,18.1447401280535,18.6351385098928,19.1255368917321,
19.6159352735713,20.1063336554106,20.5967320372499,21.0871304190892,21.5775288009285,
22.0679271827678,22.558325564607,23.0487239464463,23.5391223282856,24.0295207101249,
24.5199190919642,25.0103174738035,25.5007158556427,25.991114237482,26.4815126193213,
26.9719110011606,27.4623093829999,27.9527077648392,28.4431061466784,28.9335045285177,
29.423902910357,29.9143012921963,30.4046996740356,30.8950980558749,31.3854964377141,
31.8758948195534,32.3662932013927,32.856691583232,33.3470899650713,33.8374883469106,
34.3278867287498,34.8182851105891,35.3086834924284,35.7990818742677,36.289480256107,
36.7798786379463,37.2702770197855,37.7606754016248,38.2510737834641,38.7414721653034,
39.2318705471427,39.722268928982,40.2126673108212,40.7030656926605,41.1934640744998,
41.6838624563391,42.1742608381784,42.6646592200177,43.1550576018569,43.6454559836962,
44.1358543655355,44.6262527473748,45.1166511292141,45.6070495110534,46.0974478928927,
46.5878462747319,47.0782446565712,47.2939563352912),.UNSPECIFIED.);
#599=B_SPLINE_CURVE_WITH_KNOTS('',3,(#33399,#33400,#33401,#33402,#33403,
#33404,#33405,#33406),.UNSPECIFIED.,.F.,.F.,(4,2,2,4),(-0.65589582858317,
-0.493988108841952,-0.303390394118172,0.),.UNSPECIFIED.);
#600=B_SPLINE_CURVE_WITH_KNOTS('',3,(#33407,#33408,#33409,#33410,#33411,
#33412,#33413,#33414,#33415,#33416,#33417,#33418,#33419,#33420,#33421,#33422,
#33423,#33424,#33425,#33426,#33427,#33428,#33429,#33430,#33431,#33432,#33433,
#33434,#33435,#33436,#33437,#33438,#33439,#33440,#33441,#33442,#33443,#33444,
#33445,#33446,#33447,#33448,#33449,#33450,#33451,#33452,#33453,#33454,#33455,
#33456,#33457,#33458,#33459,#33460,#33461,#33462,#33463,#33464,#33465,#33466,
#33467,#33468,#33469,#33470,#33471,#33472,#33473,#33474,#33475,#33476,#33477,
#33478,#33479,#33480,#33481,#33482,#33483,#33484,#33485,#33486,#33487,#33488,
#33489,#33490,#33491,#33492,#33493,#33494,#33495,#33496,#33497,#33498,#33499,
#33500,#33501,#33502,#33503,#33504,#33505,#33506),.UNSPECIFIED.,.F.,.F.,
(4,1,1,1,1,1,1,1,1,1,1,1,1,1,1,1,1,1,1,1,1,1,1,1,1,1,1,1,1,1,1,1,1,1,1,
1,1,1,1,1,1,1,1,1,1,1,1,1,1,1,1,1,1,1,1,1,1,1,1,1,1,1,1,1,1,1,1,1,1,1,1,
1,1,1,1,1,1,1,1,1,1,1,1,1,1,1,1,1,1,1,1,1,1,1,1,1,1,4),(7.04827039213814,
7.26398207085813,7.75438045269741,8.24477883453669,8.73517721637598,9.22557559821526,
9.71597398005454,10.2063723618938,10.6967707437331,11.1871691255724,11.6775675074117,
12.167965889251,12.6583642710902,13.1487626529295,13.6391610347688,14.1295594166081,
14.6199577984474,15.1103561802867,15.6007545621259,16.0911529439652,16.5815513258045,
17.0719497076438,17.5623480894831,18.0527464713224,18.5431448531616,19.0335432350009,
19.5239416168402,20.0143399986795,20.5047383805188,20.9951367623581,21.4855351441973,
21.9759335260366,22.4663319078759,22.9567302897152,23.4471286715545,23.9375270533938,
24.427925435233,24.9183238170723,25.4087221989116,25.8991205807509,26.3895189625902,
26.8799173444295,27.3703157262687,27.860714108108,28.3511124899473,28.8415108717866,
29.3319092536259,29.8223076354652,30.3127060173044,30.8031043991437,31.293502780983,
31.7839011628223,32.2742995446616,32.7646979265009,33.2550963083402,33.7454946901794,
34.2358930720187,34.726291453858,35.2166898356973,35.7070882175366,36.1974865993759,
36.6878849812151,37.1782833630544,37.6686817448937,38.159080126733,38.6494785085723,
39.1398768904116,39.6302752722508,40.1206736540901,40.6110720359294,41.1014704177687,
41.591868799608,42.0822671814473,42.5726655632865,43.0630639451258,43.5534623269651,
44.0438607088044,44.5342590906437,45.024657472483,45.5150558543222,46.0054542361615,
46.4958526180008,46.9862509998401,47.4766493816794,47.9670477635187,48.4574461453579,
48.9478445271972,49.4382429090365,49.9286412908758,50.4190396727151,50.9094380545544,
51.3998364363936,51.8902348182329,52.3806332000722,52.8710315819115,53.3614299637508,
53.8518283455901,54.3422267274293),.UNSPECIFIED.);
#601=B_SPLINE_CURVE_WITH_KNOTS('',3,(#33912,#33913,#33914,#33915,#33916,
#33917,#33918,#33919,#33920,#33921,#33922,#33923,#33924,#33925,#33926,#33927,
#33928,#33929,#33930,#33931,#33932,#33933,#33934,#33935,#33936,#33937,#33938,
#33939,#33940,#33941,#33942,#33943,#33944,#33945,#33946,#33947,#33948,#33949,
#33950,#33951,#33952,#33953,#33954,#33955,#33956,#33957,#33958,#33959,#33960,
#33961,#33962,#33963),.UNSPECIFIED.,.F.,.F.,(4,3,3,3,3,3,3,3,3,3,3,3,3,
3,3,3,3,4),(0.,0.113340575159357,0.226679014314907,0.308971226978626,0.33157413936908,
0.375660801919025,0.487626538864722,0.577647057858466,0.619647639286856,
0.64272677861779,0.752674952041405,0.769690750751205,0.865631662359576,
0.890410497383802,0.914699066264647,1.0235933763044,1.1305555281797,1.15345439718469),
 .UNSPECIFIED.);
#602=B_SPLINE_CURVE_WITH_KNOTS('',3,(#33965,#33966,#33967,#33968,#33969,
#33970,#33971,#33972,#33973,#33974,#33975,#33976,#33977,#33978,#33979,#33980,
#33981,#33982,#33983,#33984,#33985,#33986,#33987,#33988,#33989,#33990,#33991,
#33992,#33993,#33994,#33995,#33996,#33997,#33998,#33999,#34000,#34001,#34002,
#34003,#34004,#34005,#34006,#34007,#34008,#34009,#34010,#34011,#34012,#34013),
 .UNSPECIFIED.,.F.,.F.,(4,3,3,3,3,3,3,3,3,3,3,3,3,3,3,3,4),(-1.15345439718468,
-1.04561219422333,-0.936713145930038,-0.898860433224647,-0.874966557602631,
-0.796527420497185,-0.698191229719559,-0.637686241518532,-0.608878950476881,
-0.496956393340814,-0.403182657386682,-0.351450861947777,-0.316015134691263,
-0.293361871620024,-0.18057397642641,-0.0674064753207201,0.),
 .UNSPECIFIED.);
#603=B_SPLINE_CURVE_WITH_KNOTS('',3,(#34014,#34015,#34016,#34017,#34018,
#34019,#34020,#34021,#34022,#34023,#34024,#34025,#34026,#34027,#34028,#34029,
#34030,#34031,#34032,#34033,#34034,#34035,#34036,#34037,#34038,#34039,#34040,
#34041,#34042,#34043,#34044,#34045,#34046,#34047,#34048,#34049,#34050,#34051,
#34052,#34053,#34054,#34055,#34056,#34057,#34058,#34059,#34060,#34061,#34062,
#34063,#34064,#34065,#34066,#34067,#34068,#34069,#34070,#34071,#34072,#34073,
#34074,#34075,#34076,#34077,#34078,#34079,#34080,#34081,#34082,#34083,#34084,
#34085,#34086,#34087,#34088,#34089,#34090,#34091,#34092,#34093,#34094,#34095,
#34096,#34097,#34098,#34099,#34100,#34101,#34102,#34103,#34104,#34105,#34106,
#34107,#34108,#34109,#34110,#34111,#34112),.UNSPECIFIED.,.F.,.F.,(4,1,1,
1,1,1,1,1,1,1,1,1,1,1,1,1,1,1,1,1,1,1,1,1,1,1,1,1,1,1,1,1,1,1,1,1,1,1,1,
1,1,1,1,1,1,1,1,1,1,1,1,1,1,1,1,1,1,1,1,1,1,1,1,1,1,1,1,1,1,1,1,1,1,1,1,
1,1,1,1,1,1,1,1,1,1,1,1,1,1,1,1,1,1,1,1,1,4),(8.50634549793094,8.5406795178856,
9.03814922646809,9.53561893505058,10.0330886436331,10.5305583522156,11.0280280607981,
11.5254977693805,12.022967477963,12.5204371865455,13.017906895128,13.5153766037105,
14.012846312293,14.5103160208755,15.007785729458,15.5052554380405,16.002725146623,
16.5001948552054,16.9976645637879,17.4951342723704,17.9926039809529,18.4900736895354,
18.9875433981179,19.4850131067004,19.9824828152829,20.4799525238654,20.9774222324479,
21.4748919410303,21.9723616496128,22.4698313581953,22.9673010667778,23.4647707753603,
23.9622404839428,24.4597101925253,24.9571799011078,25.4546496096903,25.9521193182728,
26.4495890268552,26.9470587354377,27.4445284440202,27.9419981526027,28.4394678611852,
28.9369375697677,29.4344072783502,29.9318769869327,30.4293466955152,30.9268164040977,
31.4242861126801,31.9217558212626,32.4192255298451,32.9166952384276,33.4141649470101,
33.9116346555926,34.4091043641751,34.9065740727576,35.4040437813401,35.9015134899225,
36.398983198505,36.8964529070875,37.39392261567,37.8913923242525,38.388862032835,
38.8863317414175,39.38380145,39.8812711585825,40.378740867165,40.8762105757474,
41.3736802843299,41.8711499929124,42.3686197014949,42.8660894100774,43.3635591186599,
43.8610288272424,44.3584985358249,44.8559682444074,45.3534379529899,45.8509076615723,
46.3483773701548,46.8458470787373,47.3433167873198,47.8407864959023,48.3382562044848,
48.8357259130673,49.3331956216498,49.8306653302323,50.3281350388148,50.8256047473972,
51.3230744559797,51.8205441645622,52.3180138731447,52.8154835817272,53.3129532903097,
53.8104229988922,54.3078927074747,54.8053624160572,55.3028321246397,55.8003018332221),
 .UNSPECIFIED.);
#604=B_SPLINE_CURVE_WITH_KNOTS('',3,(#34618,#34619,#34620,#34621,#34622,
#34623,#34624,#34625),.UNSPECIFIED.,.F.,.F.,(4,2,2,4),(0.,0.169060128143195,
0.259665069689286,0.357335207358759),.UNSPECIFIED.);
#605=B_SPLINE_CURVE_WITH_KNOTS('',3,(#34627,#34628,#34629,#34630,#34631,
#34632,#34633,#34634),.UNSPECIFIED.,.F.,.F.,(4,2,2,4),(-0.357325312875839,
-0.2596648130129,-0.169069150031592,0.),.UNSPECIFIED.);
#606=B_SPLINE_CURVE_WITH_KNOTS('',3,(#34635,#34636,#34637,#34638),
 .UNSPECIFIED.,.F.,.F.,(4,4),(9.27143058288951,9.42477796076936),
 .UNSPECIFIED.);
#607=B_SPLINE_CURVE_WITH_KNOTS('',3,(#34644,#34645,#34646,#34647,#34648,
#34649,#34650,#34651),.UNSPECIFIED.,.F.,.F.,(4,2,2,4),(-0.415677006509016,
-0.300108570891024,-0.193253093542031,0.),.UNSPECIFIED.);
#608=B_SPLINE_CURVE_WITH_KNOTS('',3,(#34653,#34654,#34655,#34656,#34657,
#34658,#34659,#34660,#34661,#34662,#34663,#34664,#34665,#34666,#34667,#34668,
#34669,#34670,#34671,#34672,#34673,#34674,#34675,#34676,#34677,#34678,#34679,
#34680,#34681,#34682,#34683,#34684,#34685,#34686,#34687,#34688,#34689,#34690,
#34691,#34692,#34693,#34694,#34695,#34696,#34697,#34698,#34699,#34700,#34701),
 .UNSPECIFIED.,.F.,.F.,(4,3,3,3,3,3,3,3,3,3,3,3,3,3,3,3,4),(-1.15166532125566,
-1.03829677946555,-0.925260930580166,-0.889798588874509,-0.857950257399306,
-0.776795567921363,-0.678445564828452,-0.620287810074686,-0.586753712344115,
-0.476556476809781,-0.383395555549721,-0.332702788626051,-0.305063279660781,
-0.282851348861602,-0.174044273864526,-0.0667784584747076,0.),
 .UNSPECIFIED.);
#609=B_SPLINE_CURVE_WITH_KNOTS('',3,(#34702,#34703,#34704,#34705,#34706,
#34707),.UNSPECIFIED.,.F.,.F.,(4,2,4),(-0.659276662925395,-0.291453031942622,
0.),.UNSPECIFIED.);
#610=B_SPLINE_CURVE_WITH_KNOTS('',3,(#35216,#35217,#35218,#35219,#35220,
#35221),.UNSPECIFIED.,.F.,.F.,(4,2,4),(0.,0.291454760594741,0.659275699695529),
 .UNSPECIFIED.);
#611=B_SPLINE_CURVE_WITH_KNOTS('',3,(#35222,#35223,#35224,#35225,#35226,
#35227,#35228,#35229,#35230,#35231,#35232,#35233,#35234,#35235,#35236,#35237,
#35238,#35239,#35240,#35241,#35242,#35243,#35244,#35245,#35246,#35247,#35248,
#35249,#35250,#35251,#35252,#35253,#35254,#35255,#35256,#35257,#35258,#35259,
#35260,#35261,#35262,#35263,#35264,#35265,#35266,#35267,#35268,#35269,#35270,
#35271,#35272,#35273,#35274,#35275,#35276,#35277,#35278,#35279,#35280,#35281,
#35282,#35283,#35284,#35285,#35286,#35287,#35288,#35289,#35290,#35291,#35292,
#35293,#35294,#35295,#35296,#35297,#35298,#35299,#35300,#35301,#35302,#35303,
#35304,#35305,#35306,#35307,#35308,#35309,#35310,#35311,#35312,#35313,#35314,
#35315,#35316,#35317,#35318,#35319,#35320,#35321),.UNSPECIFIED.,.F.,.F.,
(4,1,1,1,1,1,1,1,1,1,1,1,1,1,1,1,1,1,1,1,1,1,1,1,1,1,1,1,1,1,1,1,1,1,1,
1,1,1,1,1,1,1,1,1,1,1,1,1,1,1,1,1,1,1,1,1,1,1,1,1,1,1,1,1,1,1,1,1,1,1,1,
1,1,1,1,1,1,1,1,1,1,1,1,1,1,1,1,1,1,1,1,1,1,1,1,1,1,4),(10.3432104236078,
10.5589221023278,11.049320484167,11.5397188660063,12.0301172478456,12.5205156296849,
13.0109140115242,13.5013123933635,13.9917107752027,14.482109157042,14.9725075388813,
15.4629059207206,15.9533043025599,16.4437026843992,16.9341010662384,17.4244994480777,
17.914897829917,18.4052962117563,18.8956945935956,19.3860929754349,19.8764913572741,
20.3668897391134,20.8572881209527,21.347686502792,21.8380848846313,22.3284832664706,
22.8188816483098,23.3092800301491,23.7996784119884,24.2900767938277,24.780475175667,
25.2708735575063,25.7612719393455,26.2516703211848,26.7420687030241,27.2324670848634,
27.7228654667027,28.213263848542,28.7036622303812,29.1940606122205,29.6844589940598,
30.1748573758991,30.6652557577384,31.1556541395777,31.6460525214169,32.1364509032562,
32.6268492850955,33.1172476669348,33.6076460487741,34.0980444306134,34.5884428124526,
35.0788411942919,35.5692395761312,36.0596379579705,36.5500363398098,37.0404347216491,
37.5308331034883,38.0212314853276,38.5116298671669,39.0020282490062,39.4924266308455,
39.9828250126848,40.473223394524,40.9636217763633,41.4540201582026,41.9444185400419,
42.4348169218812,42.9252153037205,43.4156136855597,43.906012067399,44.3964104492383,
44.8868088310776,45.3772072129169,45.8676055947562,46.3580039765954,46.8484023584347,
47.338800740274,47.8291991221133,48.3195975039526,48.8099958857919,49.3003942676311,
49.7907926494704,50.2811910313097,50.771589413149,51.2619877949883,51.7523861768276,
52.2427845586669,52.7331829405061,53.2235813223454,53.7139797041847,54.204378086024,
54.6947764678633,55.1851748497025,55.6755732315418,56.1659716133811,56.6563699952204,
57.1467683770597,57.637166758899),.UNSPECIFIED.);
#612=B_SPLINE_CURVE_WITH_KNOTS('',3,(#35727,#35728,#35729,#35730,#35731,
#35732,#35733,#35734,#35735,#35736,#35737,#35738,#35739,#35740,#35741,#35742,
#35743,#35744,#35745,#35746,#35747,#35748,#35749,#35750,#35751,#35752,#35753,
#35754,#35755,#35756,#35757,#35758,#35759,#35760,#35761,#35762,#35763,#35764,
#35765,#35766,#35767,#35768,#35769,#35770,#35771,#35772,#35773,#35774,#35775,
#35776,#35777,#35778),.UNSPECIFIED.,.F.,.F.,(4,3,3,3,3,3,3,3,3,3,3,3,3,
3,3,3,3,4),(0.,0.107536136059931,0.216397453782157,0.296736912822655,0.319843387978689,
0.356604402276694,0.46652467054214,0.547074483570674,0.595815754020393,
0.619047604484214,0.731049962231847,0.749314772119407,0.849902409403466,
0.873496419878896,0.898389588300942,1.01139267280479,1.12432918309124,1.15166532125564),
 .UNSPECIFIED.);
#613=B_SPLINE_CURVE_WITH_KNOTS('',3,(#35779,#35780,#35781,#35782,#35783,
#35784,#35785,#35786,#35787,#35788,#35789,#35790,#35791,#35792,#35793,#35794,
#35795,#35796,#35797,#35798,#35799,#35800,#35801,#35802,#35803,#35804,#35805,
#35806,#35807,#35808,#35809,#35810,#35811,#35812,#35813,#35814,#35815,#35816,
#35817,#35818,#35819,#35820,#35821,#35822,#35823,#35824,#35825,#35826,#35827,
#35828,#35829,#35830,#35831,#35832,#35833,#35834,#35835,#35836,#35837,#35838,
#35839,#35840,#35841,#35842,#35843,#35844,#35845,#35846,#35847,#35848,#35849,
#35850,#35851,#35852,#35853,#35854,#35855,#35856,#35857,#35858,#35859,#35860,
#35861,#35862,#35863,#35864,#35865,#35866,#35867,#35868,#35869,#35870,#35871,
#35872,#35873,#35874,#35875,#35876,#35877),.UNSPECIFIED.,.F.,.F.,(4,1,1,
1,1,1,1,1,1,1,1,1,1,1,1,1,1,1,1,1,1,1,1,1,1,1,1,1,1,1,1,1,1,1,1,1,1,1,1,
1,1,1,1,1,1,1,1,1,1,1,1,1,1,1,1,1,1,1,1,1,1,1,1,1,1,1,1,1,1,1,1,1,1,1,1,
1,1,1,1,1,1,1,1,1,1,1,1,1,1,1,1,1,1,1,1,1,4),(11.8012855294006,11.8356195493552,
12.3330892579377,12.8305589665202,13.3280286751027,13.8254983836852,14.3229680922677,
14.8204378008502,15.3179075094327,15.8153772180151,16.3128469265976,16.8103166351801,
17.3077863437626,17.8052560523451,18.3027257609276,18.8001954695101,19.2976651780926,
19.7951348866751,20.2926045952576,20.79007430384,21.2875440124225,21.785013721005,
22.2824834295875,22.77995313817,23.2774228467525,23.774892555335,24.2723622639175,
24.7698319725,25.2673016810825,25.7647713896649,26.2622410982474,26.7597108068299,
27.2571805154124,27.7546502239949,28.2521199325774,28.7495896411599,29.2470593497424,
29.7445290583249,30.2419987669074,30.7394684754899,31.2369381840723,31.7344078926548,
32.2318776012373,32.7293473098198,33.2268170184023,33.7242867269848,34.2217564355673,
34.7192261441498,35.2166958527323,35.7141655613148,36.2116352698972,36.7091049784797,
37.2065746870622,37.7040443956447,38.2015141042272,38.6989838128097,39.1964535213922,
39.6939232299747,40.1913929385572,40.6888626471397,41.1863323557221,41.6838020643046,
42.1812717728871,42.6787414814696,43.1762111900521,43.6736808986346,44.1711506072171,
44.6686203157996,45.1660900243821,45.6635597329645,46.161029441547,46.6584991501295,
47.155968858712,47.6534385672945,48.150908275877,48.6483779844595,49.145847693042,
49.6433174016245,50.140787110207,50.6382568187894,51.1357265273719,51.6331962359544,
52.1306659445369,52.6281356531194,53.1256053617019,53.6230750702844,54.1205447788669,
54.6180144874494,55.1154841960319,55.6129539046143,56.1104236131968,56.6078933217793,
57.1053630303618,57.6028327389443,58.1003024475268,58.5977721561093,59.0952418646918),
 .UNSPECIFIED.);
#614=B_SPLINE_CURVE_WITH_KNOTS('',3,(#36383,#36384,#36385,#36386,#36387,
#36388,#36389,#36390),.UNSPECIFIED.,.F.,.F.,(4,2,2,4),(0.,0.193236966585146,
0.300098749787204,0.415673620384002),.UNSPECIFIED.);
#1454=(
BOUNDED_CURVE()
B_SPLINE_CURVE(2,(#37008,#37009,#37010),.UNSPECIFIED.,.F.,.F.)
B_SPLINE_CURVE_WITH_KNOTS((3,3),(0.0827095041446621,0.74095125061019),
 .UNSPECIFIED.)
CURVE()
GEOMETRIC_REPRESENTATION_ITEM()
RATIONAL_B_SPLINE_CURVE((1.02109552796081,1.1000775419169,1.1000775419169))
REPRESENTATION_ITEM('')
);
#1455=(
BOUNDED_CURVE()
B_SPLINE_CURVE(2,(#37012,#37013,#37014),.UNSPECIFIED.,.F.,.F.)
B_SPLINE_CURVE_WITH_KNOTS((3,3),(0.0827095041446618,1.39919299707572),
 .UNSPECIFIED.)
CURVE()
GEOMETRIC_REPRESENTATION_ITEM()
RATIONAL_B_SPLINE_CURVE((1.02109552796081,1.17905955587299,1.02109552796081))
REPRESENTATION_ITEM('')
);
#1456=(
BOUNDED_CURVE()
B_SPLINE_CURVE(2,(#37016,#37017,#37018),.UNSPECIFIED.,.F.,.F.)
B_SPLINE_CURVE_WITH_KNOTS((3,3),(0.082709504144662,1.39919299707572),
 .UNSPECIFIED.)
CURVE()
GEOMETRIC_REPRESENTATION_ITEM()
RATIONAL_B_SPLINE_CURVE((1.02109552796081,1.17905955587299,1.02109552796081))
REPRESENTATION_ITEM('')
);
#1457=(
BOUNDED_CURVE()
B_SPLINE_CURVE(2,(#37020,#37021,#37022),.UNSPECIFIED.,.F.,.F.)
B_SPLINE_CURVE_WITH_KNOTS((3,3),(0.0827095041446621,1.39919299707572),
 .UNSPECIFIED.)
CURVE()
GEOMETRIC_REPRESENTATION_ITEM()
RATIONAL_B_SPLINE_CURVE((1.02109552796081,1.17905955587299,1.02109552796081))
REPRESENTATION_ITEM('')
);
#1458=(
BOUNDED_CURVE()
B_SPLINE_CURVE(2,(#37024,#37025,#37026),.UNSPECIFIED.,.F.,.F.)
B_SPLINE_CURVE_WITH_KNOTS((3,3),(0.0827095041446625,1.39919299707572),
 .UNSPECIFIED.)
CURVE()
GEOMETRIC_REPRESENTATION_ITEM()
RATIONAL_B_SPLINE_CURVE((1.02109552796081,1.17905955587299,1.02109552796081))
REPRESENTATION_ITEM('')
);
#1459=(
BOUNDED_CURVE()
B_SPLINE_CURVE(2,(#37028,#37029,#37030),.UNSPECIFIED.,.F.,.F.)
B_SPLINE_CURVE_WITH_KNOTS((3,3),(0.0827095041446619,1.39919299707572),
 .UNSPECIFIED.)
CURVE()
GEOMETRIC_REPRESENTATION_ITEM()
RATIONAL_B_SPLINE_CURVE((1.02109552796081,1.17905955587299,1.02109552796081))
REPRESENTATION_ITEM('')
);
#1460=(
BOUNDED_CURVE()
B_SPLINE_CURVE(2,(#37031,#37032,#37033),.UNSPECIFIED.,.F.,.F.)
B_SPLINE_CURVE_WITH_KNOTS((3,3),(0.74095125061019,1.39919299707572),
 .UNSPECIFIED.)
CURVE()
GEOMETRIC_REPRESENTATION_ITEM()
RATIONAL_B_SPLINE_CURVE((1.1000775419169,1.1000775419169,1.02109552796081))
REPRESENTATION_ITEM('')
);
#1461=(
BOUNDED_CURVE()
B_SPLINE_CURVE(2,(#37038,#37039,#37040),.UNSPECIFIED.,.F.,.F.)
B_SPLINE_CURVE_WITH_KNOTS((3,3),(0.0827095041446625,1.39919299707572),
 .UNSPECIFIED.)
CURVE()
GEOMETRIC_REPRESENTATION_ITEM()
RATIONAL_B_SPLINE_CURVE((1.02109552796081,1.17905955587299,1.02109552796081))
REPRESENTATION_ITEM('')
);
#1462=(
BOUNDED_CURVE()
B_SPLINE_CURVE(2,(#37045,#37046,#37047),.UNSPECIFIED.,.F.,.F.)
B_SPLINE_CURVE_WITH_KNOTS((3,3),(0.0827095041446616,1.39919299707572),
 .UNSPECIFIED.)
CURVE()
GEOMETRIC_REPRESENTATION_ITEM()
RATIONAL_B_SPLINE_CURVE((1.02109552796081,1.17905955587299,1.02109552796081))
REPRESENTATION_ITEM('')
);
#1463=(
BOUNDED_CURVE()
B_SPLINE_CURVE(2,(#37051,#37052,#37053),.UNSPECIFIED.,.F.,.F.)
B_SPLINE_CURVE_WITH_KNOTS((3,3),(0.082709504144662,1.39919299707572),
 .UNSPECIFIED.)
CURVE()
GEOMETRIC_REPRESENTATION_ITEM()
RATIONAL_B_SPLINE_CURVE((1.02109552796081,1.17905955587299,1.02109552796081))
REPRESENTATION_ITEM('')
);
#1464=(
BOUNDED_CURVE()
B_SPLINE_CURVE(2,(#37056,#37057,#37058),.UNSPECIFIED.,.F.,.F.)
B_SPLINE_CURVE_WITH_KNOTS((3,3),(0.0827095041446617,1.39919299707572),
 .UNSPECIFIED.)
CURVE()
GEOMETRIC_REPRESENTATION_ITEM()
RATIONAL_B_SPLINE_CURVE((1.02109552796081,1.17905955587299,1.02109552796081))
REPRESENTATION_ITEM('')
);
#1465=(
BOUNDED_CURVE()
B_SPLINE_CURVE(2,(#37060,#37061,#37062),.UNSPECIFIED.,.F.,.F.)
B_SPLINE_CURVE_WITH_KNOTS((3,3),(0.74095125061019,1.39919299707572),
 .UNSPECIFIED.)
CURVE()
GEOMETRIC_REPRESENTATION_ITEM()
RATIONAL_B_SPLINE_CURVE((1.1000775419169,1.1000775419169,1.02109552796081))
REPRESENTATION_ITEM('')
);
#1466=(
BOUNDED_CURVE()
B_SPLINE_CURVE(2,(#37067,#37068,#37069),.UNSPECIFIED.,.F.,.F.)
B_SPLINE_CURVE_WITH_KNOTS((3,3),(0.0827095041446617,0.74095125061019),
 .UNSPECIFIED.)
CURVE()
GEOMETRIC_REPRESENTATION_ITEM()
RATIONAL_B_SPLINE_CURVE((1.02109552796081,1.1000775419169,1.1000775419169))
REPRESENTATION_ITEM('')
);
#1467=(
BOUNDED_CURVE()
B_SPLINE_CURVE(2,(#37070,#37071,#37072),.UNSPECIFIED.,.F.,.F.)
B_SPLINE_CURVE_WITH_KNOTS((3,3),(0.0827095041446618,1.39919299707572),
 .UNSPECIFIED.)
CURVE()
GEOMETRIC_REPRESENTATION_ITEM()
RATIONAL_B_SPLINE_CURVE((1.02109552796081,1.17905955587299,1.02109552796081))
REPRESENTATION_ITEM('')
);
#1514=SHAPE_REPRESENTATION_RELATIONSHIP('SRR','None',#59303,#1534);
#1534=ADVANCED_BREP_SHAPE_REPRESENTATION('',(#1581),#59190);
#1554=STYLED_ITEM('',(#59572),#1581);
#1581=MANIFOLD_SOLID_BREP('Relief valve plug',#22810);
#1629=FACE_BOUND('',#4244,.T.);
#1630=FACE_BOUND('',#4246,.T.);
#1631=FACE_BOUND('',#4252,.T.);
#1632=FACE_BOUND('',#4255,.T.);
#1633=FACE_BOUND('',#4260,.T.);
#1836=PLANE('',#23239);
#1837=PLANE('',#23244);
#1838=PLANE('',#23245);
#1839=PLANE('',#23246);
#1840=PLANE('',#23247);
#1841=PLANE('',#23248);
#1842=PLANE('',#23249);
#1843=PLANE('',#23250);
#1844=PLANE('',#23251);
#1845=PLANE('',#23252);
#1846=PLANE('',#23254);
#1847=PLANE('',#23255);
#1848=PLANE('',#23257);
#1849=PLANE('',#23258);
#1850=PLANE('',#23260);
#1851=PLANE('',#23261);
#1852=PLANE('',#23263);
#1853=PLANE('',#23264);
#1854=PLANE('',#23266);
#1855=PLANE('',#23267);
#1856=PLANE('',#23269);
#1857=PLANE('',#23270);
#1858=PLANE('',#23272);
#1859=PLANE('',#23273);
#1860=PLANE('',#23275);
#1861=PLANE('',#23276);
#1862=PLANE('',#23278);
#1863=PLANE('',#23279);
#1864=PLANE('',#23281);
#1865=PLANE('',#23282);
#1866=PLANE('',#23284);
#1867=PLANE('',#23285);
#1868=PLANE('',#23287);
#1869=PLANE('',#23288);
#1870=PLANE('',#23290);
#1871=PLANE('',#23291);
#1872=PLANE('',#23293);
#1873=PLANE('',#23295);
#1874=PLANE('',#23296);
#1875=PLANE('',#23297);
#1876=PLANE('',#23299);
#1877=PLANE('',#23300);
#1878=PLANE('',#23302);
#1879=PLANE('',#23303);
#1880=PLANE('',#23305);
#1881=PLANE('',#23306);
#1882=PLANE('',#23308);
#1883=PLANE('',#23309);
#1884=PLANE('',#23311);
#1885=PLANE('',#23312);
#1886=PLANE('',#23314);
#1887=PLANE('',#23315);
#1888=PLANE('',#23317);
#1889=PLANE('',#23318);
#1890=PLANE('',#23320);
#1891=PLANE('',#23321);
#1892=PLANE('',#23323);
#1893=PLANE('',#23324);
#1894=PLANE('',#23326);
#1895=PLANE('',#23327);
#1896=PLANE('',#23329);
#1897=PLANE('',#23330);
#1898=PLANE('',#23332);
#1899=PLANE('',#23333);
#1900=PLANE('',#23335);
#1901=PLANE('',#23336);
#1902=PLANE('',#23338);
#1903=PLANE('',#23339);
#1904=PLANE('',#23341);
#1905=PLANE('',#23342);
#1906=PLANE('',#23344);
#1907=PLANE('',#23345);
#1908=PLANE('',#23347);
#1909=PLANE('',#23348);
#1910=PLANE('',#23350);
#1911=PLANE('',#23351);
#1912=PLANE('',#23353);
#1913=PLANE('',#23354);
#1914=PLANE('',#23356);
#1915=PLANE('',#23357);
#1916=PLANE('',#23359);
#1917=PLANE('',#23360);
#1918=PLANE('',#23362);
#1919=PLANE('',#23363);
#1920=PLANE('',#23365);
#1921=PLANE('',#23366);
#1922=PLANE('',#23368);
#1923=PLANE('',#23369);
#1924=PLANE('',#23371);
#1925=PLANE('',#23372);
#1926=PLANE('',#23374);
#1927=PLANE('',#23375);
#1928=PLANE('',#23377);
#1929=PLANE('',#23378);
#1930=PLANE('',#23380);
#1931=PLANE('',#23381);
#1932=PLANE('',#23383);
#1933=PLANE('',#23384);
#1934=PLANE('',#23387);
#1935=PLANE('',#23388);
#1936=PLANE('',#23391);
#1937=PLANE('',#23392);
#1938=PLANE('',#23394);
#1939=PLANE('',#23395);
#1940=PLANE('',#23397);
#1941=PLANE('',#23398);
#1942=PLANE('',#23400);
#1943=PLANE('',#23401);
#1944=PLANE('',#23403);
#1945=PLANE('',#23404);
#1946=PLANE('',#23406);
#1947=PLANE('',#23407);
#1948=PLANE('',#23409);
#1949=PLANE('',#23410);
#1950=PLANE('',#23412);
#1951=PLANE('',#23413);
#1952=PLANE('',#23415);
#1953=PLANE('',#23416);
#1954=PLANE('',#23418);
#1955=PLANE('',#23419);
#1956=PLANE('',#23421);
#1957=PLANE('',#23422);
#1958=PLANE('',#23424);
#1959=PLANE('',#23425);
#1960=PLANE('',#23427);
#1961=PLANE('',#23428);
#1962=PLANE('',#23430);
#1963=PLANE('',#23431);
#1964=PLANE('',#23435);
#1965=PLANE('',#23436);
#1966=PLANE('',#23437);
#1967=PLANE('',#23440);
#1968=PLANE('',#23441);
#1969=PLANE('',#23443);
#1970=PLANE('',#23445);
#1971=PLANE('',#23446);
#1972=PLANE('',#23451);
#1973=PLANE('',#23454);
#1974=PLANE('',#23490);
#2434=CYLINDRICAL_SURFACE('',#23229,0.7475);
#2435=CYLINDRICAL_SURFACE('',#23231,0.7475);
#2436=CYLINDRICAL_SURFACE('',#23232,0.7475);
#2437=CYLINDRICAL_SURFACE('',#23233,0.7475);
#2438=CYLINDRICAL_SURFACE('',#23234,0.7475);
#2439=CYLINDRICAL_SURFACE('',#23235,0.7475);
#2440=CYLINDRICAL_SURFACE('',#23236,0.7475);
#2441=CYLINDRICAL_SURFACE('',#23237,0.7475);
#2442=CYLINDRICAL_SURFACE('',#23243,0.7475);
#2443=CYLINDRICAL_SURFACE('',#23447,0.3);
#2444=CYLINDRICAL_SURFACE('',#23456,0.7431);
#2445=CYLINDRICAL_SURFACE('',#23457,0.9);
#2759=FACE_OUTER_BOUND('',#4094,.T.);
#2760=FACE_OUTER_BOUND('',#4095,.T.);
#2761=FACE_OUTER_BOUND('',#4096,.T.);
#2762=FACE_OUTER_BOUND('',#4097,.T.);
#2763=FACE_OUTER_BOUND('',#4098,.T.);
#2764=FACE_OUTER_BOUND('',#4099,.T.);
#2765=FACE_OUTER_BOUND('',#4100,.T.);
#2766=FACE_OUTER_BOUND('',#4101,.T.);
#2767=FACE_OUTER_BOUND('',#4102,.T.);
#2768=FACE_OUTER_BOUND('',#4103,.T.);
#2769=FACE_OUTER_BOUND('',#4104,.T.);
#2770=FACE_OUTER_BOUND('',#4105,.T.);
#2771=FACE_OUTER_BOUND('',#4106,.T.);
#2772=FACE_OUTER_BOUND('',#4107,.T.);
#2773=FACE_OUTER_BOUND('',#4108,.T.);
#2774=FACE_OUTER_BOUND('',#4109,.T.);
#2775=FACE_OUTER_BOUND('',#4110,.T.);
#2776=FACE_OUTER_BOUND('',#4111,.T.);
#2777=FACE_OUTER_BOUND('',#4112,.T.);
#2778=FACE_OUTER_BOUND('',#4113,.T.);
#2779=FACE_OUTER_BOUND('',#4114,.T.);
#2780=FACE_OUTER_BOUND('',#4115,.T.);
#2781=FACE_OUTER_BOUND('',#4116,.T.);
#2782=FACE_OUTER_BOUND('',#4117,.T.);
#2783=FACE_OUTER_BOUND('',#4118,.T.);
#2784=FACE_OUTER_BOUND('',#4119,.T.);
#2785=FACE_OUTER_BOUND('',#4120,.T.);
#2786=FACE_OUTER_BOUND('',#4121,.T.);
#2787=FACE_OUTER_BOUND('',#4122,.T.);
#2788=FACE_OUTER_BOUND('',#4123,.T.);
#2789=FACE_OUTER_BOUND('',#4124,.T.);
#2790=FACE_OUTER_BOUND('',#4125,.T.);
#2791=FACE_OUTER_BOUND('',#4126,.T.);
#2792=FACE_OUTER_BOUND('',#4127,.T.);
#2793=FACE_OUTER_BOUND('',#4128,.T.);
#2794=FACE_OUTER_BOUND('',#4129,.T.);
#2795=FACE_OUTER_BOUND('',#4130,.T.);
#2796=FACE_OUTER_BOUND('',#4131,.T.);
#2797=FACE_OUTER_BOUND('',#4132,.T.);
#2798=FACE_OUTER_BOUND('',#4133,.T.);
#2799=FACE_OUTER_BOUND('',#4134,.T.);
#2800=FACE_OUTER_BOUND('',#4135,.T.);
#2801=FACE_OUTER_BOUND('',#4136,.T.);
#2802=FACE_OUTER_BOUND('',#4137,.T.);
#2803=FACE_OUTER_BOUND('',#4138,.T.);
#2804=FACE_OUTER_BOUND('',#4139,.T.);
#2805=FACE_OUTER_BOUND('',#4140,.T.);
#2806=FACE_OUTER_BOUND('',#4141,.T.);
#2807=FACE_OUTER_BOUND('',#4142,.T.);
#2808=FACE_OUTER_BOUND('',#4143,.T.);
#2809=FACE_OUTER_BOUND('',#4144,.T.);
#2810=FACE_OUTER_BOUND('',#4145,.T.);
#2811=FACE_OUTER_BOUND('',#4146,.T.);
#2812=FACE_OUTER_BOUND('',#4147,.T.);
#2813=FACE_OUTER_BOUND('',#4148,.T.);
#2814=FACE_OUTER_BOUND('',#4149,.T.);
#2815=FACE_OUTER_BOUND('',#4150,.T.);
#2816=FACE_OUTER_BOUND('',#4151,.T.);
#2817=FACE_OUTER_BOUND('',#4152,.T.);
#2818=FACE_OUTER_BOUND('',#4153,.T.);
#2819=FACE_OUTER_BOUND('',#4154,.T.);
#2820=FACE_OUTER_BOUND('',#4155,.T.);
#2821=FACE_OUTER_BOUND('',#4156,.T.);
#2822=FACE_OUTER_BOUND('',#4157,.T.);
#2823=FACE_OUTER_BOUND('',#4158,.T.);
#2824=FACE_OUTER_BOUND('',#4159,.T.);
#2825=FACE_OUTER_BOUND('',#4160,.T.);
#2826=FACE_OUTER_BOUND('',#4161,.T.);
#2827=FACE_OUTER_BOUND('',#4162,.T.);
#2828=FACE_OUTER_BOUND('',#4163,.T.);
#2829=FACE_OUTER_BOUND('',#4164,.T.);
#2830=FACE_OUTER_BOUND('',#4165,.T.);
#2831=FACE_OUTER_BOUND('',#4166,.T.);
#2832=FACE_OUTER_BOUND('',#4167,.T.);
#2833=FACE_OUTER_BOUND('',#4168,.T.);
#2834=FACE_OUTER_BOUND('',#4169,.T.);
#2835=FACE_OUTER_BOUND('',#4170,.T.);
#2836=FACE_OUTER_BOUND('',#4171,.T.);
#2837=FACE_OUTER_BOUND('',#4172,.T.);
#2838=FACE_OUTER_BOUND('',#4173,.T.);
#2839=FACE_OUTER_BOUND('',#4174,.T.);
#2840=FACE_OUTER_BOUND('',#4175,.T.);
#2841=FACE_OUTER_BOUND('',#4176,.T.);
#2842=FACE_OUTER_BOUND('',#4177,.T.);
#2843=FACE_OUTER_BOUND('',#4178,.T.);
#2844=FACE_OUTER_BOUND('',#4179,.T.);
#2845=FACE_OUTER_BOUND('',#4180,.T.);
#2846=FACE_OUTER_BOUND('',#4181,.T.);
#2847=FACE_OUTER_BOUND('',#4182,.T.);
#2848=FACE_OUTER_BOUND('',#4183,.T.);
#2849=FACE_OUTER_BOUND('',#4184,.T.);
#2850=FACE_OUTER_BOUND('',#4185,.T.);
#2851=FACE_OUTER_BOUND('',#4186,.T.);
#2852=FACE_OUTER_BOUND('',#4187,.T.);
#2853=FACE_OUTER_BOUND('',#4188,.T.);
#2854=FACE_OUTER_BOUND('',#4189,.T.);
#2855=FACE_OUTER_BOUND('',#4190,.T.);
#2856=FACE_OUTER_BOUND('',#4191,.T.);
#2857=FACE_OUTER_BOUND('',#4192,.T.);
#2858=FACE_OUTER_BOUND('',#4193,.T.);
#2859=FACE_OUTER_BOUND('',#4194,.T.);
#2860=FACE_OUTER_BOUND('',#4195,.T.);
#2861=FACE_OUTER_BOUND('',#4196,.T.);
#2862=FACE_OUTER_BOUND('',#4197,.T.);
#2863=FACE_OUTER_BOUND('',#4198,.T.);
#2864=FACE_OUTER_BOUND('',#4199,.T.);
#2865=FACE_OUTER_BOUND('',#4200,.T.);
#2866=FACE_OUTER_BOUND('',#4201,.T.);
#2867=FACE_OUTER_BOUND('',#4202,.T.);
#2868=FACE_OUTER_BOUND('',#4203,.T.);
#2869=FACE_OUTER_BOUND('',#4204,.T.);
#2870=FACE_OUTER_BOUND('',#4205,.T.);
#2871=FACE_OUTER_BOUND('',#4206,.T.);
#2872=FACE_OUTER_BOUND('',#4207,.T.);
#2873=FACE_OUTER_BOUND('',#4208,.T.);
#2874=FACE_OUTER_BOUND('',#4209,.T.);
#2875=FACE_OUTER_BOUND('',#4210,.T.);
#2876=FACE_OUTER_BOUND('',#4211,.T.);
#2877=FACE_OUTER_BOUND('',#4212,.T.);
#2878=FACE_OUTER_BOUND('',#4213,.T.);
#2879=FACE_OUTER_BOUND('',#4214,.T.);
#2880=FACE_OUTER_BOUND('',#4215,.T.);
#2881=FACE_OUTER_BOUND('',#4216,.T.);
#2882=FACE_OUTER_BOUND('',#4217,.T.);
#2883=FACE_OUTER_BOUND('',#4218,.T.);
#2884=FACE_OUTER_BOUND('',#4219,.T.);
#2885=FACE_OUTER_BOUND('',#4220,.T.);
#2886=FACE_OUTER_BOUND('',#4221,.T.);
#2887=FACE_OUTER_BOUND('',#4222,.T.);
#2888=FACE_OUTER_BOUND('',#4223,.T.);
#2889=FACE_OUTER_BOUND('',#4224,.T.);
#2890=FACE_OUTER_BOUND('',#4225,.T.);
#2891=FACE_OUTER_BOUND('',#4226,.T.);
#2892=FACE_OUTER_BOUND('',#4227,.T.);
#2893=FACE_OUTER_BOUND('',#4228,.T.);
#2894=FACE_OUTER_BOUND('',#4229,.T.);
#2895=FACE_OUTER_BOUND('',#4230,.T.);
#2896=FACE_OUTER_BOUND('',#4231,.T.);
#2897=FACE_OUTER_BOUND('',#4232,.T.);
#2898=FACE_OUTER_BOUND('',#4233,.T.);
#2899=FACE_OUTER_BOUND('',#4234,.T.);
#2900=FACE_OUTER_BOUND('',#4235,.T.);
#2901=FACE_OUTER_BOUND('',#4236,.T.);
#2902=FACE_OUTER_BOUND('',#4237,.T.);
#2903=FACE_OUTER_BOUND('',#4238,.T.);
#2904=FACE_OUTER_BOUND('',#4239,.T.);
#2905=FACE_OUTER_BOUND('',#4240,.T.);
#2906=FACE_OUTER_BOUND('',#4241,.T.);
#2907=FACE_OUTER_BOUND('',#4242,.T.);
#2908=FACE_OUTER_BOUND('',#4243,.T.);
#2909=FACE_OUTER_BOUND('',#4245,.T.);
#2910=FACE_OUTER_BOUND('',#4247,.T.);
#2911=FACE_OUTER_BOUND('',#4248,.T.);
#2912=FACE_OUTER_BOUND('',#4249,.T.);
#2913=FACE_OUTER_BOUND('',#4250,.T.);
#2914=FACE_OUTER_BOUND('',#4251,.T.);
#2915=FACE_OUTER_BOUND('',#4253,.T.);
#2916=FACE_OUTER_BOUND('',#4254,.T.);
#2917=FACE_OUTER_BOUND('',#4256,.T.);
#2918=FACE_OUTER_BOUND('',#4257,.T.);
#2919=FACE_OUTER_BOUND('',#4258,.T.);
#2920=FACE_OUTER_BOUND('',#4259,.T.);
#4094=EDGE_LOOP('',(#15038,#15039,#15040,#15041));
#4095=EDGE_LOOP('',(#15042,#15043,#15044,#15045));
#4096=EDGE_LOOP('',(#15046,#15047,#15048,#15049));
#4097=EDGE_LOOP('',(#15050,#15051,#15052,#15053));
#4098=EDGE_LOOP('',(#15054,#15055,#15056,#15057));
#4099=EDGE_LOOP('',(#15058,#15059,#15060,#15061));
#4100=EDGE_LOOP('',(#15062,#15063,#15064,#15065));
#4101=EDGE_LOOP('',(#15066,#15067,#15068,#15069,#15070));
#4102=EDGE_LOOP('',(#15071,#15072,#15073,#15074));
#4103=EDGE_LOOP('',(#15075,#15076,#15077,#15078));
#4104=EDGE_LOOP('',(#15079,#15080,#15081,#15082,#15083,#15084,#15085,#15086,
#15087,#15088,#15089,#15090));
#4105=EDGE_LOOP('',(#15091,#15092,#15093,#15094,#15095,#15096,#15097,#15098,
#15099,#15100));
#4106=EDGE_LOOP('',(#15101,#15102,#15103));
#4107=EDGE_LOOP('',(#15104,#15105,#15106,#15107,#15108,#15109,#15110,#15111,
#15112,#15113,#15114));
#4108=EDGE_LOOP('',(#15115,#15116,#15117,#15118));
#4109=EDGE_LOOP('',(#15119,#15120,#15121,#15122));
#4110=EDGE_LOOP('',(#15123,#15124,#15125,#15126));
#4111=EDGE_LOOP('',(#15127,#15128,#15129,#15130));
#4112=EDGE_LOOP('',(#15131,#15132,#15133,#15134));
#4113=EDGE_LOOP('',(#15135,#15136,#15137,#15138));
#4114=EDGE_LOOP('',(#15139,#15140,#15141,#15142));
#4115=EDGE_LOOP('',(#15143,#15144,#15145,#15146));
#4116=EDGE_LOOP('',(#15147,#15148,#15149,#15150,#15151,#15152));
#4117=EDGE_LOOP('',(#15153,#15154,#15155,#15156));
#4118=EDGE_LOOP('',(#15157,#15158,#15159));
#4119=EDGE_LOOP('',(#15160,#15161,#15162,#15163));
#4120=EDGE_LOOP('',(#15164,#15165,#15166));
#4121=EDGE_LOOP('',(#15167,#15168,#15169,#15170));
#4122=EDGE_LOOP('',(#15171,#15172,#15173));
#4123=EDGE_LOOP('',(#15174,#15175,#15176,#15177));
#4124=EDGE_LOOP('',(#15178,#15179,#15180));
#4125=EDGE_LOOP('',(#15181,#15182,#15183,#15184));
#4126=EDGE_LOOP('',(#15185,#15186,#15187));
#4127=EDGE_LOOP('',(#15188,#15189,#15190,#15191));
#4128=EDGE_LOOP('',(#15192,#15193,#15194));
#4129=EDGE_LOOP('',(#15195,#15196,#15197,#15198));
#4130=EDGE_LOOP('',(#15199,#15200,#15201));
#4131=EDGE_LOOP('',(#15202,#15203,#15204,#15205));
#4132=EDGE_LOOP('',(#15206,#15207,#15208));
#4133=EDGE_LOOP('',(#15209,#15210,#15211,#15212));
#4134=EDGE_LOOP('',(#15213,#15214,#15215));
#4135=EDGE_LOOP('',(#15216,#15217,#15218,#15219));
#4136=EDGE_LOOP('',(#15220,#15221,#15222));
#4137=EDGE_LOOP('',(#15223,#15224,#15225,#15226));
#4138=EDGE_LOOP('',(#15227,#15228,#15229));
#4139=EDGE_LOOP('',(#15230,#15231,#15232,#15233));
#4140=EDGE_LOOP('',(#15234,#15235,#15236));
#4141=EDGE_LOOP('',(#15237,#15238,#15239,#15240));
#4142=EDGE_LOOP('',(#15241,#15242,#15243));
#4143=EDGE_LOOP('',(#15244,#15245,#15246,#15247));
#4144=EDGE_LOOP('',(#15248,#15249,#15250));
#4145=EDGE_LOOP('',(#15251,#15252,#15253));
#4146=EDGE_LOOP('',(#15254,#15255,#15256,#15257));
#4147=EDGE_LOOP('',(#15258,#15259,#15260,#15261));
#4148=EDGE_LOOP('',(#15262,#15263,#15264));
#4149=EDGE_LOOP('',(#15265,#15266,#15267,#15268));
#4150=EDGE_LOOP('',(#15269,#15270,#15271));
#4151=EDGE_LOOP('',(#15272,#15273,#15274,#15275));
#4152=EDGE_LOOP('',(#15276,#15277,#15278));
#4153=EDGE_LOOP('',(#15279,#15280,#15281,#15282));
#4154=EDGE_LOOP('',(#15283,#15284,#15285));
#4155=EDGE_LOOP('',(#15286,#15287,#15288,#15289));
#4156=EDGE_LOOP('',(#15290,#15291,#15292));
#4157=EDGE_LOOP('',(#15293,#15294,#15295,#15296));
#4158=EDGE_LOOP('',(#15297,#15298,#15299));
#4159=EDGE_LOOP('',(#15300,#15301,#15302,#15303));
#4160=EDGE_LOOP('',(#15304,#15305,#15306));
#4161=EDGE_LOOP('',(#15307,#15308,#15309,#15310));
#4162=EDGE_LOOP('',(#15311,#15312,#15313));
#4163=EDGE_LOOP('',(#15314,#15315,#15316,#15317));
#4164=EDGE_LOOP('',(#15318,#15319,#15320));
#4165=EDGE_LOOP('',(#15321,#15322,#15323,#15324));
#4166=EDGE_LOOP('',(#15325,#15326,#15327));
#4167=EDGE_LOOP('',(#15328,#15329,#15330,#15331));
#4168=EDGE_LOOP('',(#15332,#15333,#15334));
#4169=EDGE_LOOP('',(#15335,#15336,#15337,#15338));
#4170=EDGE_LOOP('',(#15339,#15340,#15341));
#4171=EDGE_LOOP('',(#15342,#15343,#15344,#15345));
#4172=EDGE_LOOP('',(#15346,#15347,#15348));
#4173=EDGE_LOOP('',(#15349,#15350,#15351,#15352));
#4174=EDGE_LOOP('',(#15353,#15354,#15355));
#4175=EDGE_LOOP('',(#15356,#15357,#15358,#15359));
#4176=EDGE_LOOP('',(#15360,#15361,#15362));
#4177=EDGE_LOOP('',(#15363,#15364,#15365,#15366));
#4178=EDGE_LOOP('',(#15367,#15368,#15369));
#4179=EDGE_LOOP('',(#15370,#15371,#15372,#15373));
#4180=EDGE_LOOP('',(#15374,#15375,#15376));
#4181=EDGE_LOOP('',(#15377,#15378,#15379,#15380));
#4182=EDGE_LOOP('',(#15381,#15382,#15383));
#4183=EDGE_LOOP('',(#15384,#15385,#15386,#15387));
#4184=EDGE_LOOP('',(#15388,#15389,#15390));
#4185=EDGE_LOOP('',(#15391,#15392,#15393,#15394));
#4186=EDGE_LOOP('',(#15395,#15396,#15397));
#4187=EDGE_LOOP('',(#15398,#15399,#15400,#15401));
#4188=EDGE_LOOP('',(#15402,#15403,#15404));
#4189=EDGE_LOOP('',(#15405,#15406,#15407,#15408));
#4190=EDGE_LOOP('',(#15409,#15410,#15411));
#4191=EDGE_LOOP('',(#15412,#15413,#15414,#15415));
#4192=EDGE_LOOP('',(#15416,#15417,#15418));
#4193=EDGE_LOOP('',(#15419,#15420,#15421,#15422));
#4194=EDGE_LOOP('',(#15423,#15424,#15425));
#4195=EDGE_LOOP('',(#15426,#15427,#15428,#15429));
#4196=EDGE_LOOP('',(#15430,#15431,#15432));
#4197=EDGE_LOOP('',(#15433,#15434,#15435,#15436));
#4198=EDGE_LOOP('',(#15437,#15438,#15439));
#4199=EDGE_LOOP('',(#15440,#15441,#15442,#15443));
#4200=EDGE_LOOP('',(#15444,#15445,#15446));
#4201=EDGE_LOOP('',(#15447,#15448,#15449,#15450));
#4202=EDGE_LOOP('',(#15451,#15452,#15453));
#4203=EDGE_LOOP('',(#15454,#15455,#15456,#15457));
#4204=EDGE_LOOP('',(#15458,#15459,#15460));
#4205=EDGE_LOOP('',(#15461,#15462,#15463,#15464));
#4206=EDGE_LOOP('',(#15465,#15466,#15467,#15468));
#4207=EDGE_LOOP('',(#15469,#15470,#15471,#15472));
#4208=EDGE_LOOP('',(#15473,#15474,#15475,#15476));
#4209=EDGE_LOOP('',(#15477,#15478,#15479,#15480));
#4210=EDGE_LOOP('',(#15481,#15482,#15483));
#4211=EDGE_LOOP('',(#15484,#15485,#15486,#15487));
#4212=EDGE_LOOP('',(#15488,#15489,#15490));
#4213=EDGE_LOOP('',(#15491,#15492,#15493,#15494));
#4214=EDGE_LOOP('',(#15495,#15496,#15497));
#4215=EDGE_LOOP('',(#15498,#15499,#15500,#15501));
#4216=EDGE_LOOP('',(#15502,#15503,#15504));
#4217=EDGE_LOOP('',(#15505,#15506,#15507,#15508));
#4218=EDGE_LOOP('',(#15509,#15510,#15511));
#4219=EDGE_LOOP('',(#15512,#15513,#15514,#15515));
#4220=EDGE_LOOP('',(#15516,#15517,#15518));
#4221=EDGE_LOOP('',(#15519,#15520,#15521,#15522));
#4222=EDGE_LOOP('',(#15523,#15524,#15525));
#4223=EDGE_LOOP('',(#15526,#15527,#15528,#15529));
#4224=EDGE_LOOP('',(#15530,#15531,#15532));
#4225=EDGE_LOOP('',(#15533,#15534,#15535,#15536));
#4226=EDGE_LOOP('',(#15537,#15538,#15539));
#4227=EDGE_LOOP('',(#15540,#15541,#15542,#15543));
#4228=EDGE_LOOP('',(#15544,#15545,#15546));
#4229=EDGE_LOOP('',(#15547,#15548,#15549,#15550));
#4230=EDGE_LOOP('',(#15551,#15552,#15553));
#4231=EDGE_LOOP('',(#15554,#15555,#15556,#15557));
#4232=EDGE_LOOP('',(#15558,#15559,#15560));
#4233=EDGE_LOOP('',(#15561,#15562,#15563,#15564));
#4234=EDGE_LOOP('',(#15565,#15566,#15567));
#4235=EDGE_LOOP('',(#15568,#15569,#15570,#15571));
#4236=EDGE_LOOP('',(#15572,#15573,#15574));
#4237=EDGE_LOOP('',(#15575,#15576,#15577,#15578,#15579,#15580,#15581,#15582,
#15583,#15584));
#4238=EDGE_LOOP('',(#15585,#15586,#15587,#15588));
#4239=EDGE_LOOP('',(#15589,#15590,#15591,#15592));
#4240=EDGE_LOOP('',(#15593,#15594,#15595,#15596));
#4241=EDGE_LOOP('',(#15597,#15598,#15599,#15600,#15601,#15602,#15603,#15604,
#15605,#15606));
#4242=EDGE_LOOP('',(#15607,#15608,#15609,#15610));
#4243=EDGE_LOOP('',(#15611));
#4244=EDGE_LOOP('',(#15612));
#4245=EDGE_LOOP('',(#15613));
#4246=EDGE_LOOP('',(#15614));
#4247=EDGE_LOOP('',(#15615,#15616,#15617,#15618));
#4248=EDGE_LOOP('',(#15619,#15620,#15621,#15622,#15623,#15624));
#4249=EDGE_LOOP('',(#15625,#15626,#15627,#15628));
#4250=EDGE_LOOP('',(#15629,#15630,#15631));
#4251=EDGE_LOOP('',(#15632));
#4252=EDGE_LOOP('',(#15633));
#4253=EDGE_LOOP('',(#15634,#15635,#15636,#15637,#15638));
#4254=EDGE_LOOP('',(#15639,#15640,#15641,#15642,#15643,#15644,#15645));
#4255=EDGE_LOOP('',(#15646));
#4256=EDGE_LOOP('',(#15647,#15648,#15649,#15650));
#4257=EDGE_LOOP('',(#15651,#15652,#15653,#15654,#15655,#15656,#15657,#15658,
#15659,#15660,#15661,#15662,#15663,#15664,#15665,#15666,#15667,#15668,#15669,
#15670,#15671,#15672,#15673,#15674,#15675,#15676,#15677,#15678,#15679,#15680,
#15681,#15682,#15683,#15684,#15685,#15686,#15687,#15688,#15689,#15690,#15691,
#15692,#15693,#15694,#15695,#15696,#15697,#15698,#15699,#15700,#15701,#15702,
#15703,#15704,#15705,#15706,#15707,#15708,#15709,#15710,#15711,#15712,#15713,
#15714,#15715,#15716,#15717,#15718,#15719,#15720,#15721,#15722,#15723,#15724,
#15725,#15726,#15727,#15728,#15729,#15730,#15731,#15732,#15733,#15734,#15735,
#15736,#15737,#15738,#15739,#15740,#15741,#15742,#15743,#15744,#15745,#15746,
#15747,#15748,#15749,#15750,#15751,#15752,#15753,#15754,#15755,#15756,#15757,
#15758,#15759,#15760,#15761,#15762,#15763,#15764,#15765,#15766,#15767,#15768,
#15769,#15770,#15771,#15772,#15773,#15774));
#4258=EDGE_LOOP('',(#15775,#15776,#15777,#15778,#15779,#15780,#15781,#15782,
#15783,#15784,#15785,#15786,#15787,#15788,#15789,#15790,#15791,#15792,#15793,
#15794,#15795,#15796,#15797,#15798,#15799,#15800,#15801,#15802,#15803,#15804,
#15805,#15806,#15807,#15808,#15809,#15810,#15811,#15812,#15813,#15814,#15815,
#15816,#15817,#15818,#15819,#15820,#15821,#15822,#15823,#15824,#15825,#15826,
#15827,#15828,#15829,#15830,#15831,#15832,#15833,#15834,#15835,#15836,#15837,
#15838));
#4259=EDGE_LOOP('',(#15839));
#4260=EDGE_LOOP('',(#15840,#15841,#15842,#15843,#15844,#15845));
#5574=LINE('',#32300,#7007);
#5575=LINE('',#32328,#7008);
#5576=LINE('',#32366,#7009);
#5577=LINE('',#32404,#7010);
#5578=LINE('',#32441,#7011);
#5579=LINE('',#32478,#7012);
#5580=LINE('',#32516,#7013);
#5581=LINE('',#32554,#7014);
#5582=LINE('',#36394,#7015);
#5583=LINE('',#36396,#7016);
#5584=LINE('',#36398,#7017);
#5585=LINE('',#36399,#7018);
#5586=LINE('',#36402,#7019);
#5587=LINE('',#36404,#7020);
#5588=LINE('',#36405,#7021);
#5589=LINE('',#36408,#7022);
#5590=LINE('',#36410,#7023);
#5591=LINE('',#36411,#7024);
#5592=LINE('',#36414,#7025);
#5593=LINE('',#36416,#7026);
#5594=LINE('',#36417,#7027);
#5595=LINE('',#36420,#7028);
#5596=LINE('',#36422,#7029);
#5597=LINE('',#36423,#7030);
#5598=LINE('',#36425,#7031);
#5599=LINE('',#36426,#7032);
#5600=LINE('',#36431,#7033);
#5601=LINE('',#36433,#7034);
#5602=LINE('',#36435,#7035);
#5603=LINE('',#36436,#7036);
#5604=LINE('',#36440,#7037);
#5605=LINE('',#36443,#7038);
#5606=LINE('',#36444,#7039);
#5607=LINE('',#36450,#7040);
#5608=LINE('',#36452,#7041);
#5609=LINE('',#36454,#7042);
#5610=LINE('',#36455,#7043);
#5611=LINE('',#36459,#7044);
#5612=LINE('',#36462,#7045);
#5613=LINE('',#36463,#7046);
#5614=LINE('',#36469,#7047);
#5615=LINE('',#36471,#7048);
#5616=LINE('',#36473,#7049);
#5617=LINE('',#36474,#7050);
#5618=LINE('',#36478,#7051);
#5619=LINE('',#36481,#7052);
#5620=LINE('',#36482,#7053);
#5621=LINE('',#36488,#7054);
#5622=LINE('',#36490,#7055);
#5623=LINE('',#36492,#7056);
#5624=LINE('',#36493,#7057);
#5625=LINE('',#36497,#7058);
#5626=LINE('',#36500,#7059);
#5627=LINE('',#36501,#7060);
#5628=LINE('',#36507,#7061);
#5629=LINE('',#36509,#7062);
#5630=LINE('',#36511,#7063);
#5631=LINE('',#36512,#7064);
#5632=LINE('',#36516,#7065);
#5633=LINE('',#36519,#7066);
#5634=LINE('',#36520,#7067);
#5635=LINE('',#36526,#7068);
#5636=LINE('',#36528,#7069);
#5637=LINE('',#36530,#7070);
#5638=LINE('',#36531,#7071);
#5639=LINE('',#36535,#7072);
#5640=LINE('',#36538,#7073);
#5641=LINE('',#36539,#7074);
#5642=LINE('',#36545,#7075);
#5643=LINE('',#36547,#7076);
#5644=LINE('',#36549,#7077);
#5645=LINE('',#36550,#7078);
#5646=LINE('',#36554,#7079);
#5647=LINE('',#36557,#7080);
#5648=LINE('',#36558,#7081);
#5649=LINE('',#36566,#7082);
#5650=LINE('',#36567,#7083);
#5651=LINE('',#36570,#7084);
#5652=LINE('',#36572,#7085);
#5653=LINE('',#36573,#7086);
#5654=LINE('',#36576,#7087);
#5655=LINE('',#36577,#7088);
#5656=LINE('',#36583,#7089);
#5657=LINE('',#36585,#7090);
#5658=LINE('',#36587,#7091);
#5659=LINE('',#36588,#7092);
#5660=LINE('',#36592,#7093);
#5661=LINE('',#36595,#7094);
#5662=LINE('',#36596,#7095);
#5663=LINE('',#36602,#7096);
#5664=LINE('',#36604,#7097);
#5665=LINE('',#36606,#7098);
#5666=LINE('',#36607,#7099);
#5667=LINE('',#36611,#7100);
#5668=LINE('',#36614,#7101);
#5669=LINE('',#36615,#7102);
#5670=LINE('',#36621,#7103);
#5671=LINE('',#36623,#7104);
#5672=LINE('',#36625,#7105);
#5673=LINE('',#36626,#7106);
#5674=LINE('',#36630,#7107);
#5675=LINE('',#36633,#7108);
#5676=LINE('',#36634,#7109);
#5677=LINE('',#36640,#7110);
#5678=LINE('',#36642,#7111);
#5679=LINE('',#36644,#7112);
#5680=LINE('',#36645,#7113);
#5681=LINE('',#36649,#7114);
#5682=LINE('',#36652,#7115);
#5683=LINE('',#36653,#7116);
#5684=LINE('',#36659,#7117);
#5685=LINE('',#36661,#7118);
#5686=LINE('',#36663,#7119);
#5687=LINE('',#36664,#7120);
#5688=LINE('',#36668,#7121);
#5689=LINE('',#36671,#7122);
#5690=LINE('',#36672,#7123);
#5691=LINE('',#36678,#7124);
#5692=LINE('',#36680,#7125);
#5693=LINE('',#36682,#7126);
#5694=LINE('',#36683,#7127);
#5695=LINE('',#36687,#7128);
#5696=LINE('',#36690,#7129);
#5697=LINE('',#36691,#7130);
#5698=LINE('',#36697,#7131);
#5699=LINE('',#36699,#7132);
#5700=LINE('',#36701,#7133);
#5701=LINE('',#36702,#7134);
#5702=LINE('',#36706,#7135);
#5703=LINE('',#36709,#7136);
#5704=LINE('',#36710,#7137);
#5705=LINE('',#36716,#7138);
#5706=LINE('',#36718,#7139);
#5707=LINE('',#36720,#7140);
#5708=LINE('',#36721,#7141);
#5709=LINE('',#36725,#7142);
#5710=LINE('',#36728,#7143);
#5711=LINE('',#36729,#7144);
#5712=LINE('',#36735,#7145);
#5713=LINE('',#36737,#7146);
#5714=LINE('',#36739,#7147);
#5715=LINE('',#36740,#7148);
#5716=LINE('',#36744,#7149);
#5717=LINE('',#36747,#7150);
#5718=LINE('',#36748,#7151);
#5719=LINE('',#36754,#7152);
#5720=LINE('',#36756,#7153);
#5721=LINE('',#36758,#7154);
#5722=LINE('',#36759,#7155);
#5723=LINE('',#36763,#7156);
#5724=LINE('',#36766,#7157);
#5725=LINE('',#36767,#7158);
#5726=LINE('',#36773,#7159);
#5727=LINE('',#36775,#7160);
#5728=LINE('',#36777,#7161);
#5729=LINE('',#36778,#7162);
#5730=LINE('',#36782,#7163);
#5731=LINE('',#36785,#7164);
#5732=LINE('',#36786,#7165);
#5733=LINE('',#36792,#7166);
#5734=LINE('',#36794,#7167);
#5735=LINE('',#36796,#7168);
#5736=LINE('',#36797,#7169);
#5737=LINE('',#36801,#7170);
#5738=LINE('',#36804,#7171);
#5739=LINE('',#36805,#7172);
#5740=LINE('',#36811,#7173);
#5741=LINE('',#36813,#7174);
#5742=LINE('',#36815,#7175);
#5743=LINE('',#36816,#7176);
#5744=LINE('',#36820,#7177);
#5745=LINE('',#36823,#7178);
#5746=LINE('',#36824,#7179);
#5747=LINE('',#36830,#7180);
#5748=LINE('',#36832,#7181);
#5749=LINE('',#36834,#7182);
#5750=LINE('',#36835,#7183);
#5751=LINE('',#36839,#7184);
#5752=LINE('',#36842,#7185);
#5753=LINE('',#36843,#7186);
#5754=LINE('',#36849,#7187);
#5755=LINE('',#36851,#7188);
#5756=LINE('',#36853,#7189);
#5757=LINE('',#36854,#7190);
#5758=LINE('',#36859,#7191);
#5759=LINE('',#36863,#7192);
#5760=LINE('',#36864,#7193);
#5761=LINE('',#36872,#7194);
#5762=LINE('',#36874,#7195);
#5763=LINE('',#36876,#7196);
#5764=LINE('',#36877,#7197);
#5765=LINE('',#36881,#7198);
#5766=LINE('',#36884,#7199);
#5767=LINE('',#36885,#7200);
#5768=LINE('',#36891,#7201);
#5769=LINE('',#36893,#7202);
#5770=LINE('',#36895,#7203);
#5771=LINE('',#36896,#7204);
#5772=LINE('',#36900,#7205);
#5773=LINE('',#36903,#7206);
#5774=LINE('',#36904,#7207);
#5775=LINE('',#36910,#7208);
#5776=LINE('',#36912,#7209);
#5777=LINE('',#36914,#7210);
#5778=LINE('',#36915,#7211);
#5779=LINE('',#36919,#7212);
#5780=LINE('',#36922,#7213);
#5781=LINE('',#36923,#7214);
#5782=LINE('',#36929,#7215);
#5783=LINE('',#36931,#7216);
#5784=LINE('',#36933,#7217);
#5785=LINE('',#36934,#7218);
#5786=LINE('',#36938,#7219);
#5787=LINE('',#36941,#7220);
#5788=LINE('',#36942,#7221);
#5789=LINE('',#36948,#7222);
#5790=LINE('',#36950,#7223);
#5791=LINE('',#36952,#7224);
#5792=LINE('',#36953,#7225);
#5793=LINE('',#36957,#7226);
#5794=LINE('',#36960,#7227);
#5795=LINE('',#36961,#7228);
#5796=LINE('',#36967,#7229);
#5797=LINE('',#36969,#7230);
#5798=LINE('',#36971,#7231);
#5799=LINE('',#36972,#7232);
#5800=LINE('',#36976,#7233);
#5801=LINE('',#36979,#7234);
#5802=LINE('',#36980,#7235);
#5803=LINE('',#36986,#7236);
#5804=LINE('',#36988,#7237);
#5805=LINE('',#36990,#7238);
#5806=LINE('',#36991,#7239);
#5807=LINE('',#36995,#7240);
#5808=LINE('',#36998,#7241);
#5809=LINE('',#36999,#7242);
#5810=LINE('',#37006,#7243);
#5811=LINE('',#37036,#7244);
#5812=LINE('',#37041,#7245);
#5813=LINE('',#37044,#7246);
#5814=LINE('',#37050,#7247);
#5815=LINE('',#37064,#7248);
#5816=LINE('',#37074,#7249);
#5817=LINE('',#37082,#7250);
#5818=LINE('',#37088,#7251);
#5819=LINE('',#37092,#7252);
#5820=LINE('',#37097,#7253);
#5821=LINE('',#37102,#7254);
#5822=LINE('',#37117,#7255);
#5823=LINE('',#37138,#7256);
#7007=VECTOR('',#25570,0.7475);
#7008=VECTOR('',#25575,0.7475);
#7009=VECTOR('',#25578,0.7475);
#7010=VECTOR('',#25581,0.7475);
#7011=VECTOR('',#25584,0.7475);
#7012=VECTOR('',#25587,0.7475);
#7013=VECTOR('',#25590,0.7475);
#7014=VECTOR('',#25593,0.7475);
#7015=VECTOR('',#25608,1.);
#7016=VECTOR('',#25609,1.);
#7017=VECTOR('',#25610,1.);
#7018=VECTOR('',#25611,1.);
#7019=VECTOR('',#25614,1.);
#7020=VECTOR('',#25615,1.);
#7021=VECTOR('',#25616,1.);
#7022=VECTOR('',#25619,1.);
#7023=VECTOR('',#25620,1.);
#7024=VECTOR('',#25621,1.);
#7025=VECTOR('',#25624,1.);
#7026=VECTOR('',#25625,1.);
#7027=VECTOR('',#25626,1.);
#7028=VECTOR('',#25629,1.);
#7029=VECTOR('',#25630,1.);
#7030=VECTOR('',#25631,1.);
#7031=VECTOR('',#25634,1.);
#7032=VECTOR('',#25635,1.);
#7033=VECTOR('',#25640,1.);
#7034=VECTOR('',#25641,1.);
#7035=VECTOR('',#25642,1.);
#7036=VECTOR('',#25643,1.);
#7037=VECTOR('',#25648,1.);
#7038=VECTOR('',#25651,1.);
#7039=VECTOR('',#25652,1.);
#7040=VECTOR('',#25659,1.);
#7041=VECTOR('',#25660,1.);
#7042=VECTOR('',#25661,1.);
#7043=VECTOR('',#25662,1.);
#7044=VECTOR('',#25667,1.);
#7045=VECTOR('',#25670,1.);
#7046=VECTOR('',#25671,1.);
#7047=VECTOR('',#25678,1.);
#7048=VECTOR('',#25679,1.);
#7049=VECTOR('',#25680,1.);
#7050=VECTOR('',#25681,1.);
#7051=VECTOR('',#25686,1.);
#7052=VECTOR('',#25689,1.);
#7053=VECTOR('',#25690,1.);
#7054=VECTOR('',#25697,1.);
#7055=VECTOR('',#25698,1.);
#7056=VECTOR('',#25699,1.);
#7057=VECTOR('',#25700,1.);
#7058=VECTOR('',#25705,1.);
#7059=VECTOR('',#25708,1.);
#7060=VECTOR('',#25709,1.);
#7061=VECTOR('',#25716,1.);
#7062=VECTOR('',#25717,1.);
#7063=VECTOR('',#25718,1.);
#7064=VECTOR('',#25719,1.);
#7065=VECTOR('',#25724,1.);
#7066=VECTOR('',#25727,1.);
#7067=VECTOR('',#25728,1.);
#7068=VECTOR('',#25735,1.);
#7069=VECTOR('',#25736,1.);
#7070=VECTOR('',#25737,1.);
#7071=VECTOR('',#25738,1.);
#7072=VECTOR('',#25743,1.);
#7073=VECTOR('',#25746,1.);
#7074=VECTOR('',#25747,1.);
#7075=VECTOR('',#25754,1.);
#7076=VECTOR('',#25755,1.);
#7077=VECTOR('',#25756,1.);
#7078=VECTOR('',#25757,1.);
#7079=VECTOR('',#25762,1.);
#7080=VECTOR('',#25765,1.);
#7081=VECTOR('',#25766,1.);
#7082=VECTOR('',#25775,1.);
#7083=VECTOR('',#25776,1.);
#7084=VECTOR('',#25779,1.);
#7085=VECTOR('',#25780,1.);
#7086=VECTOR('',#25781,1.);
#7087=VECTOR('',#25784,1.);
#7088=VECTOR('',#25785,1.);
#7089=VECTOR('',#25792,1.);
#7090=VECTOR('',#25793,1.);
#7091=VECTOR('',#25794,1.);
#7092=VECTOR('',#25795,1.);
#7093=VECTOR('',#25800,1.);
#7094=VECTOR('',#25803,1.);
#7095=VECTOR('',#25804,1.);
#7096=VECTOR('',#25811,1.);
#7097=VECTOR('',#25812,1.);
#7098=VECTOR('',#25813,1.);
#7099=VECTOR('',#25814,1.);
#7100=VECTOR('',#25819,1.);
#7101=VECTOR('',#25822,1.);
#7102=VECTOR('',#25823,1.);
#7103=VECTOR('',#25830,1.);
#7104=VECTOR('',#25831,1.);
#7105=VECTOR('',#25832,1.);
#7106=VECTOR('',#25833,1.);
#7107=VECTOR('',#25838,1.);
#7108=VECTOR('',#25841,1.);
#7109=VECTOR('',#25842,1.);
#7110=VECTOR('',#25849,1.);
#7111=VECTOR('',#25850,1.);
#7112=VECTOR('',#25851,1.);
#7113=VECTOR('',#25852,1.);
#7114=VECTOR('',#25857,1.);
#7115=VECTOR('',#25860,1.);
#7116=VECTOR('',#25861,1.);
#7117=VECTOR('',#25868,1.);
#7118=VECTOR('',#25869,1.);
#7119=VECTOR('',#25870,1.);
#7120=VECTOR('',#25871,1.);
#7121=VECTOR('',#25876,1.);
#7122=VECTOR('',#25879,1.);
#7123=VECTOR('',#25880,1.);
#7124=VECTOR('',#25887,1.);
#7125=VECTOR('',#25888,1.);
#7126=VECTOR('',#25889,1.);
#7127=VECTOR('',#25890,1.);
#7128=VECTOR('',#25895,1.);
#7129=VECTOR('',#25898,1.);
#7130=VECTOR('',#25899,1.);
#7131=VECTOR('',#25906,1.);
#7132=VECTOR('',#25907,1.);
#7133=VECTOR('',#25908,1.);
#7134=VECTOR('',#25909,1.);
#7135=VECTOR('',#25914,1.);
#7136=VECTOR('',#25917,1.);
#7137=VECTOR('',#25918,1.);
#7138=VECTOR('',#25925,1.);
#7139=VECTOR('',#25926,1.);
#7140=VECTOR('',#25927,1.);
#7141=VECTOR('',#25928,1.);
#7142=VECTOR('',#25933,1.);
#7143=VECTOR('',#25936,1.);
#7144=VECTOR('',#25937,1.);
#7145=VECTOR('',#25944,1.);
#7146=VECTOR('',#25945,1.);
#7147=VECTOR('',#25946,1.);
#7148=VECTOR('',#25947,1.);
#7149=VECTOR('',#25952,1.);
#7150=VECTOR('',#25955,1.);
#7151=VECTOR('',#25956,1.);
#7152=VECTOR('',#25963,1.);
#7153=VECTOR('',#25964,1.);
#7154=VECTOR('',#25965,1.);
#7155=VECTOR('',#25966,1.);
#7156=VECTOR('',#25971,1.);
#7157=VECTOR('',#25974,1.);
#7158=VECTOR('',#25975,1.);
#7159=VECTOR('',#25982,1.);
#7160=VECTOR('',#25983,1.);
#7161=VECTOR('',#25984,1.);
#7162=VECTOR('',#25985,1.);
#7163=VECTOR('',#25990,1.);
#7164=VECTOR('',#25993,1.);
#7165=VECTOR('',#25994,1.);
#7166=VECTOR('',#26001,1.);
#7167=VECTOR('',#26002,1.);
#7168=VECTOR('',#26003,1.);
#7169=VECTOR('',#26004,1.);
#7170=VECTOR('',#26009,1.);
#7171=VECTOR('',#26012,1.);
#7172=VECTOR('',#26013,1.);
#7173=VECTOR('',#26020,1.);
#7174=VECTOR('',#26021,1.);
#7175=VECTOR('',#26022,1.);
#7176=VECTOR('',#26023,1.);
#7177=VECTOR('',#26028,1.);
#7178=VECTOR('',#26031,1.);
#7179=VECTOR('',#26032,1.);
#7180=VECTOR('',#26039,1.);
#7181=VECTOR('',#26040,1.);
#7182=VECTOR('',#26041,1.);
#7183=VECTOR('',#26042,1.);
#7184=VECTOR('',#26047,1.);
#7185=VECTOR('',#26050,1.);
#7186=VECTOR('',#26051,1.);
#7187=VECTOR('',#26058,1.);
#7188=VECTOR('',#26059,1.);
#7189=VECTOR('',#26060,1.);
#7190=VECTOR('',#26061,1.);
#7191=VECTOR('',#26066,1.);
#7192=VECTOR('',#26071,1.);
#7193=VECTOR('',#26072,1.);
#7194=VECTOR('',#26081,1.);
#7195=VECTOR('',#26082,1.);
#7196=VECTOR('',#26083,1.);
#7197=VECTOR('',#26084,1.);
#7198=VECTOR('',#26089,1.);
#7199=VECTOR('',#26092,1.);
#7200=VECTOR('',#26093,1.);
#7201=VECTOR('',#26100,1.);
#7202=VECTOR('',#26101,1.);
#7203=VECTOR('',#26102,1.);
#7204=VECTOR('',#26103,1.);
#7205=VECTOR('',#26108,1.);
#7206=VECTOR('',#26111,1.);
#7207=VECTOR('',#26112,1.);
#7208=VECTOR('',#26119,1.);
#7209=VECTOR('',#26120,1.);
#7210=VECTOR('',#26121,1.);
#7211=VECTOR('',#26122,1.);
#7212=VECTOR('',#26127,1.);
#7213=VECTOR('',#26130,1.);
#7214=VECTOR('',#26131,1.);
#7215=VECTOR('',#26138,1.);
#7216=VECTOR('',#26139,1.);
#7217=VECTOR('',#26140,1.);
#7218=VECTOR('',#26141,1.);
#7219=VECTOR('',#26146,1.);
#7220=VECTOR('',#26149,1.);
#7221=VECTOR('',#26150,1.);
#7222=VECTOR('',#26157,1.);
#7223=VECTOR('',#26158,1.);
#7224=VECTOR('',#26159,1.);
#7225=VECTOR('',#26160,1.);
#7226=VECTOR('',#26165,1.);
#7227=VECTOR('',#26168,1.);
#7228=VECTOR('',#26169,1.);
#7229=VECTOR('',#26176,1.);
#7230=VECTOR('',#26177,1.);
#7231=VECTOR('',#26178,1.);
#7232=VECTOR('',#26179,1.);
#7233=VECTOR('',#26184,1.);
#7234=VECTOR('',#26187,1.);
#7235=VECTOR('',#26188,1.);
#7236=VECTOR('',#26195,1.);
#7237=VECTOR('',#26196,1.);
#7238=VECTOR('',#26197,1.);
#7239=VECTOR('',#26198,1.);
#7240=VECTOR('',#26203,1.);
#7241=VECTOR('',#26206,1.);
#7242=VECTOR('',#26207,1.);
#7243=VECTOR('',#26216,1.18258529610859);
#7244=VECTOR('',#26219,1.);
#7245=VECTOR('',#26220,1.);
#7246=VECTOR('',#26223,1.);
#7247=VECTOR('',#26226,1.);
#7248=VECTOR('',#26229,1.18258529610859);
#7249=VECTOR('',#26234,1.);
#7250=VECTOR('',#26245,1.);
#7251=VECTOR('',#26252,0.3);
#7252=VECTOR('',#26257,0.3);
#7253=VECTOR('',#26264,0.7931);
#7254=VECTOR('',#26271,0.7431);
#7255=VECTOR('',#26300,0.9);
#7256=VECTOR('',#26339,0.87);
#8446=CIRCLE('',#23230,0.7475);
#8447=CIRCLE('',#23238,0.7475);
#8448=CIRCLE('',#23240,0.82685);
#8449=CIRCLE('',#23241,0.82685);
#8450=CIRCLE('',#23242,0.7475);
#8451=CIRCLE('',#23253,0.9);
#8452=CIRCLE('',#23256,0.9);
#8453=CIRCLE('',#23259,0.9);
#8454=CIRCLE('',#23262,0.9);
#8455=CIRCLE('',#23265,0.9);
#8456=CIRCLE('',#23268,0.9);
#8457=CIRCLE('',#23271,0.9);
#8458=CIRCLE('',#23274,0.9);
#8459=CIRCLE('',#23277,0.9);
#8460=CIRCLE('',#23280,0.9);
#8461=CIRCLE('',#23283,0.9);
#8462=CIRCLE('',#23286,0.9);
#8463=CIRCLE('',#23289,0.9);
#8464=CIRCLE('',#23292,0.9);
#8465=CIRCLE('',#23294,0.9);
#8466=CIRCLE('',#23298,0.9);
#8467=CIRCLE('',#23301,0.9);
#8468=CIRCLE('',#23304,0.9);
#8469=CIRCLE('',#23307,0.9);
#8470=CIRCLE('',#23310,0.9);
#8471=CIRCLE('',#23313,0.9);
#8472=CIRCLE('',#23316,0.9);
#8473=CIRCLE('',#23319,0.9);
#8474=CIRCLE('',#23322,0.9);
#8475=CIRCLE('',#23325,0.9);
#8476=CIRCLE('',#23328,0.9);
#8477=CIRCLE('',#23331,0.9);
#8478=CIRCLE('',#23334,0.9);
#8479=CIRCLE('',#23337,0.9);
#8480=CIRCLE('',#23340,0.9);
#8481=CIRCLE('',#23343,0.9);
#8482=CIRCLE('',#23346,0.9);
#8483=CIRCLE('',#23349,0.9);
#8484=CIRCLE('',#23352,0.9);
#8485=CIRCLE('',#23355,0.9);
#8486=CIRCLE('',#23358,0.9);
#8487=CIRCLE('',#23361,0.9);
#8488=CIRCLE('',#23364,0.9);
#8489=CIRCLE('',#23367,0.9);
#8490=CIRCLE('',#23370,0.9);
#8491=CIRCLE('',#23373,0.9);
#8492=CIRCLE('',#23376,0.9);
#8493=CIRCLE('',#23379,0.9);
#8494=CIRCLE('',#23382,0.9);
#8495=CIRCLE('',#23385,0.9);
#8496=CIRCLE('',#23386,0.9);
#8497=CIRCLE('',#23389,0.9);
#8498=CIRCLE('',#23390,0.9);
#8499=CIRCLE('',#23393,0.9);
#8500=CIRCLE('',#23396,0.9);
#8501=CIRCLE('',#23399,0.9);
#8502=CIRCLE('',#23402,0.9);
#8503=CIRCLE('',#23405,0.9);
#8504=CIRCLE('',#23408,0.9);
#8505=CIRCLE('',#23411,0.9);
#8506=CIRCLE('',#23414,0.9);
#8507=CIRCLE('',#23417,0.9);
#8508=CIRCLE('',#23420,0.9);
#8509=CIRCLE('',#23423,0.9);
#8510=CIRCLE('',#23426,0.9);
#8511=CIRCLE('',#23429,0.9);
#8512=CIRCLE('',#23432,0.9);
#8513=CIRCLE('',#23434,1.045);
#8514=CIRCLE('',#23439,1.045);
#8515=CIRCLE('',#23442,0.9);
#8516=CIRCLE('',#23444,0.7431);
#8517=CIRCLE('',#23448,0.3);
#8518=CIRCLE('',#23449,0.3);
#8519=CIRCLE('',#23452,0.7531);
#8520=CIRCLE('',#23455,0.7431);
#8521=CIRCLE('',#23458,0.9);
#8522=CIRCLE('',#23459,0.9);
#8523=CIRCLE('',#23460,0.9);
#8524=CIRCLE('',#23461,0.9);
#8525=CIRCLE('',#23462,0.9);
#8526=CIRCLE('',#23463,0.9);
#8527=CIRCLE('',#23464,0.9);
#8528=CIRCLE('',#23465,0.9);
#8529=CIRCLE('',#23466,0.9);
#8530=CIRCLE('',#23467,0.9);
#8531=CIRCLE('',#23468,0.9);
#8532=CIRCLE('',#23469,0.9);
#8533=CIRCLE('',#23470,0.9);
#8534=CIRCLE('',#23471,0.9);
#8535=CIRCLE('',#23472,0.9);
#8536=CIRCLE('',#23473,0.9);
#8537=CIRCLE('',#23474,0.9);
#8538=CIRCLE('',#23475,0.9);
#8539=CIRCLE('',#23476,0.9);
#8540=CIRCLE('',#23477,0.9);
#8541=CIRCLE('',#23478,0.9);
#8542=CIRCLE('',#23479,0.9);
#8543=CIRCLE('',#23480,0.9);
#8544=CIRCLE('',#23481,0.9);
#8545=CIRCLE('',#23482,0.9);
#8546=CIRCLE('',#23483,0.9);
#8547=CIRCLE('',#23484,0.9);
#8548=CIRCLE('',#23485,0.9);
#8549=CIRCLE('',#23486,0.9);
#8550=CIRCLE('',#23487,0.9);
#8551=CIRCLE('',#23489,0.84);
#9306=VERTEX_POINT('',#32298);
#9307=VERTEX_POINT('',#32299);
#9308=VERTEX_POINT('',#32301);
#9309=VERTEX_POINT('',#32313);
#9310=VERTEX_POINT('',#32326);
#9311=VERTEX_POINT('',#32327);
#9312=VERTEX_POINT('',#32364);
#9313=VERTEX_POINT('',#32365);
#9314=VERTEX_POINT('',#32402);
#9315=VERTEX_POINT('',#32403);
#9316=VERTEX_POINT('',#32439);
#9317=VERTEX_POINT('',#32440);
#9318=VERTEX_POINT('',#32476);
#9319=VERTEX_POINT('',#32477);
#9320=VERTEX_POINT('',#32514);
#9321=VERTEX_POINT('',#32515);
#9322=VERTEX_POINT('',#32552);
#9323=VERTEX_POINT('',#32553);
#9324=VERTEX_POINT('',#32555);
#9325=VERTEX_POINT('',#33095);
#9326=VERTEX_POINT('',#33096);
#9327=VERTEX_POINT('',#33105);
#9328=VERTEX_POINT('',#33398);
#9329=VERTEX_POINT('',#33911);
#9330=VERTEX_POINT('',#33964);
#9331=VERTEX_POINT('',#34626);
#9332=VERTEX_POINT('',#34640);
#9333=VERTEX_POINT('',#34643);
#9334=VERTEX_POINT('',#34652);
#9335=VERTEX_POINT('',#35215);
#9336=VERTEX_POINT('',#35726);
#9337=VERTEX_POINT('',#36392);
#9338=VERTEX_POINT('',#36393);
#9339=VERTEX_POINT('',#36395);
#9340=VERTEX_POINT('',#36397);
#9341=VERTEX_POINT('',#36401);
#9342=VERTEX_POINT('',#36403);
#9343=VERTEX_POINT('',#36407);
#9344=VERTEX_POINT('',#36409);
#9345=VERTEX_POINT('',#36413);
#9346=VERTEX_POINT('',#36415);
#9347=VERTEX_POINT('',#36419);
#9348=VERTEX_POINT('',#36421);
#9349=VERTEX_POINT('',#36429);
#9350=VERTEX_POINT('',#36430);
#9351=VERTEX_POINT('',#36432);
#9352=VERTEX_POINT('',#36434);
#9353=VERTEX_POINT('',#36438);
#9354=VERTEX_POINT('',#36442);
#9355=VERTEX_POINT('',#36448);
#9356=VERTEX_POINT('',#36449);
#9357=VERTEX_POINT('',#36451);
#9358=VERTEX_POINT('',#36453);
#9359=VERTEX_POINT('',#36457);
#9360=VERTEX_POINT('',#36461);
#9361=VERTEX_POINT('',#36467);
#9362=VERTEX_POINT('',#36468);
#9363=VERTEX_POINT('',#36470);
#9364=VERTEX_POINT('',#36472);
#9365=VERTEX_POINT('',#36476);
#9366=VERTEX_POINT('',#36480);
#9367=VERTEX_POINT('',#36486);
#9368=VERTEX_POINT('',#36487);
#9369=VERTEX_POINT('',#36489);
#9370=VERTEX_POINT('',#36491);
#9371=VERTEX_POINT('',#36495);
#9372=VERTEX_POINT('',#36499);
#9373=VERTEX_POINT('',#36505);
#9374=VERTEX_POINT('',#36506);
#9375=VERTEX_POINT('',#36508);
#9376=VERTEX_POINT('',#36510);
#9377=VERTEX_POINT('',#36514);
#9378=VERTEX_POINT('',#36518);
#9379=VERTEX_POINT('',#36524);
#9380=VERTEX_POINT('',#36525);
#9381=VERTEX_POINT('',#36527);
#9382=VERTEX_POINT('',#36529);
#9383=VERTEX_POINT('',#36533);
#9384=VERTEX_POINT('',#36537);
#9385=VERTEX_POINT('',#36543);
#9386=VERTEX_POINT('',#36544);
#9387=VERTEX_POINT('',#36546);
#9388=VERTEX_POINT('',#36548);
#9389=VERTEX_POINT('',#36552);
#9390=VERTEX_POINT('',#36556);
#9391=VERTEX_POINT('',#36562);
#9392=VERTEX_POINT('',#36563);
#9393=VERTEX_POINT('',#36565);
#9394=VERTEX_POINT('',#36569);
#9395=VERTEX_POINT('',#36571);
#9396=VERTEX_POINT('',#36575);
#9397=VERTEX_POINT('',#36581);
#9398=VERTEX_POINT('',#36582);
#9399=VERTEX_POINT('',#36584);
#9400=VERTEX_POINT('',#36586);
#9401=VERTEX_POINT('',#36590);
#9402=VERTEX_POINT('',#36594);
#9403=VERTEX_POINT('',#36600);
#9404=VERTEX_POINT('',#36601);
#9405=VERTEX_POINT('',#36603);
#9406=VERTEX_POINT('',#36605);
#9407=VERTEX_POINT('',#36609);
#9408=VERTEX_POINT('',#36613);
#9409=VERTEX_POINT('',#36619);
#9410=VERTEX_POINT('',#36620);
#9411=VERTEX_POINT('',#36622);
#9412=VERTEX_POINT('',#36624);
#9413=VERTEX_POINT('',#36628);
#9414=VERTEX_POINT('',#36632);
#9415=VERTEX_POINT('',#36638);
#9416=VERTEX_POINT('',#36639);
#9417=VERTEX_POINT('',#36641);
#9418=VERTEX_POINT('',#36643);
#9419=VERTEX_POINT('',#36647);
#9420=VERTEX_POINT('',#36651);
#9421=VERTEX_POINT('',#36657);
#9422=VERTEX_POINT('',#36658);
#9423=VERTEX_POINT('',#36660);
#9424=VERTEX_POINT('',#36662);
#9425=VERTEX_POINT('',#36666);
#9426=VERTEX_POINT('',#36670);
#9427=VERTEX_POINT('',#36676);
#9428=VERTEX_POINT('',#36677);
#9429=VERTEX_POINT('',#36679);
#9430=VERTEX_POINT('',#36681);
#9431=VERTEX_POINT('',#36685);
#9432=VERTEX_POINT('',#36689);
#9433=VERTEX_POINT('',#36695);
#9434=VERTEX_POINT('',#36696);
#9435=VERTEX_POINT('',#36698);
#9436=VERTEX_POINT('',#36700);
#9437=VERTEX_POINT('',#36704);
#9438=VERTEX_POINT('',#36708);
#9439=VERTEX_POINT('',#36714);
#9440=VERTEX_POINT('',#36715);
#9441=VERTEX_POINT('',#36717);
#9442=VERTEX_POINT('',#36719);
#9443=VERTEX_POINT('',#36723);
#9444=VERTEX_POINT('',#36727);
#9445=VERTEX_POINT('',#36733);
#9446=VERTEX_POINT('',#36734);
#9447=VERTEX_POINT('',#36736);
#9448=VERTEX_POINT('',#36738);
#9449=VERTEX_POINT('',#36742);
#9450=VERTEX_POINT('',#36746);
#9451=VERTEX_POINT('',#36752);
#9452=VERTEX_POINT('',#36753);
#9453=VERTEX_POINT('',#36755);
#9454=VERTEX_POINT('',#36757);
#9455=VERTEX_POINT('',#36761);
#9456=VERTEX_POINT('',#36765);
#9457=VERTEX_POINT('',#36771);
#9458=VERTEX_POINT('',#36772);
#9459=VERTEX_POINT('',#36774);
#9460=VERTEX_POINT('',#36776);
#9461=VERTEX_POINT('',#36780);
#9462=VERTEX_POINT('',#36784);
#9463=VERTEX_POINT('',#36790);
#9464=VERTEX_POINT('',#36791);
#9465=VERTEX_POINT('',#36793);
#9466=VERTEX_POINT('',#36795);
#9467=VERTEX_POINT('',#36799);
#9468=VERTEX_POINT('',#36803);
#9469=VERTEX_POINT('',#36809);
#9470=VERTEX_POINT('',#36810);
#9471=VERTEX_POINT('',#36812);
#9472=VERTEX_POINT('',#36814);
#9473=VERTEX_POINT('',#36818);
#9474=VERTEX_POINT('',#36822);
#9475=VERTEX_POINT('',#36828);
#9476=VERTEX_POINT('',#36829);
#9477=VERTEX_POINT('',#36831);
#9478=VERTEX_POINT('',#36833);
#9479=VERTEX_POINT('',#36837);
#9480=VERTEX_POINT('',#36841);
#9481=VERTEX_POINT('',#36847);
#9482=VERTEX_POINT('',#36848);
#9483=VERTEX_POINT('',#36850);
#9484=VERTEX_POINT('',#36852);
#9485=VERTEX_POINT('',#36856);
#9486=VERTEX_POINT('',#36858);
#9487=VERTEX_POINT('',#36862);
#9488=VERTEX_POINT('',#36866);
#9489=VERTEX_POINT('',#36870);
#9490=VERTEX_POINT('',#36871);
#9491=VERTEX_POINT('',#36873);
#9492=VERTEX_POINT('',#36875);
#9493=VERTEX_POINT('',#36879);
#9494=VERTEX_POINT('',#36883);
#9495=VERTEX_POINT('',#36889);
#9496=VERTEX_POINT('',#36890);
#9497=VERTEX_POINT('',#36892);
#9498=VERTEX_POINT('',#36894);
#9499=VERTEX_POINT('',#36898);
#9500=VERTEX_POINT('',#36902);
#9501=VERTEX_POINT('',#36908);
#9502=VERTEX_POINT('',#36909);
#9503=VERTEX_POINT('',#36911);
#9504=VERTEX_POINT('',#36913);
#9505=VERTEX_POINT('',#36917);
#9506=VERTEX_POINT('',#36921);
#9507=VERTEX_POINT('',#36927);
#9508=VERTEX_POINT('',#36928);
#9509=VERTEX_POINT('',#36930);
#9510=VERTEX_POINT('',#36932);
#9511=VERTEX_POINT('',#36936);
#9512=VERTEX_POINT('',#36940);
#9513=VERTEX_POINT('',#36946);
#9514=VERTEX_POINT('',#36947);
#9515=VERTEX_POINT('',#36949);
#9516=VERTEX_POINT('',#36951);
#9517=VERTEX_POINT('',#36955);
#9518=VERTEX_POINT('',#36959);
#9519=VERTEX_POINT('',#36965);
#9520=VERTEX_POINT('',#36966);
#9521=VERTEX_POINT('',#36968);
#9522=VERTEX_POINT('',#36970);
#9523=VERTEX_POINT('',#36974);
#9524=VERTEX_POINT('',#36978);
#9525=VERTEX_POINT('',#36984);
#9526=VERTEX_POINT('',#36985);
#9527=VERTEX_POINT('',#36987);
#9528=VERTEX_POINT('',#36989);
#9529=VERTEX_POINT('',#36993);
#9530=VERTEX_POINT('',#36997);
#9531=VERTEX_POINT('',#37003);
#9532=VERTEX_POINT('',#37005);
#9533=VERTEX_POINT('',#37007);
#9534=VERTEX_POINT('',#37011);
#9535=VERTEX_POINT('',#37015);
#9536=VERTEX_POINT('',#37019);
#9537=VERTEX_POINT('',#37023);
#9538=VERTEX_POINT('',#37027);
#9539=VERTEX_POINT('',#37035);
#9540=VERTEX_POINT('',#37037);
#9541=VERTEX_POINT('',#37043);
#9542=VERTEX_POINT('',#37049);
#9543=VERTEX_POINT('',#37055);
#9544=VERTEX_POINT('',#37059);
#9545=VERTEX_POINT('',#37063);
#9546=VERTEX_POINT('',#37066);
#9547=VERTEX_POINT('',#37076);
#9548=VERTEX_POINT('',#37079);
#9549=VERTEX_POINT('',#37085);
#9550=VERTEX_POINT('',#37087);
#9551=VERTEX_POINT('',#37091);
#9552=VERTEX_POINT('',#37094);
#9553=VERTEX_POINT('',#37099);
#9554=VERTEX_POINT('',#37136);
#11523=EDGE_CURVE('',#9306,#9307,#5574,.T.);
#11524=EDGE_CURVE('',#9306,#9308,#581,.T.);
#11525=EDGE_CURVE('',#9309,#9308,#8446,.T.);
#11526=EDGE_CURVE('',#9307,#9309,#582,.T.);
#11527=EDGE_CURVE('',#9310,#9311,#5575,.T.);
#11528=EDGE_CURVE('',#9310,#9306,#583,.T.);
#11529=EDGE_CURVE('',#9311,#9307,#584,.T.);
#11530=EDGE_CURVE('',#9312,#9313,#5576,.T.);
#11531=EDGE_CURVE('',#9312,#9310,#585,.T.);
#11532=EDGE_CURVE('',#9313,#9311,#586,.T.);
#11533=EDGE_CURVE('',#9314,#9315,#5577,.T.);
#11534=EDGE_CURVE('',#9314,#9312,#587,.T.);
#11535=EDGE_CURVE('',#9315,#9313,#588,.T.);
#11536=EDGE_CURVE('',#9316,#9317,#5578,.T.);
#11537=EDGE_CURVE('',#9316,#9314,#589,.T.);
#11538=EDGE_CURVE('',#9317,#9315,#590,.T.);
#11539=EDGE_CURVE('',#9318,#9319,#5579,.T.);
#11540=EDGE_CURVE('',#9318,#9316,#591,.T.);
#11541=EDGE_CURVE('',#9319,#9317,#592,.T.);
#11542=EDGE_CURVE('',#9320,#9321,#5580,.T.);
#11543=EDGE_CURVE('',#9320,#9318,#593,.T.);
#11544=EDGE_CURVE('',#9321,#9319,#594,.T.);
#11545=EDGE_CURVE('',#9322,#9323,#5581,.T.);
#11546=EDGE_CURVE('',#9324,#9322,#8447,.T.);
#11547=EDGE_CURVE('',#9324,#9320,#595,.T.);
#11548=EDGE_CURVE('',#9323,#9321,#596,.T.);
#11549=EDGE_CURVE('',#9325,#9326,#597,.T.);
#11550=EDGE_CURVE('',#9327,#9325,#598,.T.);
#11551=EDGE_CURVE('',#9328,#9327,#599,.T.);
#11552=EDGE_CURVE('',#9328,#9326,#600,.T.);
#11553=EDGE_CURVE('',#9326,#9329,#601,.T.);
#11554=EDGE_CURVE('',#9330,#9328,#602,.T.);
#11555=EDGE_CURVE('',#9330,#9329,#603,.T.);
#11556=EDGE_CURVE('',#9329,#9309,#604,.T.);
#11557=EDGE_CURVE('',#9331,#9330,#605,.T.);
#11558=EDGE_CURVE('',#9331,#9323,#606,.T.);
#11559=EDGE_CURVE('',#9327,#9332,#8448,.T.);
#11560=EDGE_CURVE('',#9332,#9327,#8449,.T.);
#11561=EDGE_CURVE('',#9327,#9333,#607,.T.);
#11562=EDGE_CURVE('',#9333,#9334,#608,.T.);
#11563=EDGE_CURVE('',#9334,#9324,#609,.T.);
#11564=EDGE_CURVE('',#9322,#9331,#8450,.T.);
#11565=EDGE_CURVE('',#9308,#9335,#610,.T.);
#11566=EDGE_CURVE('',#9334,#9335,#611,.T.);
#11567=EDGE_CURVE('',#9335,#9336,#612,.T.);
#11568=EDGE_CURVE('',#9333,#9336,#613,.T.);
#11569=EDGE_CURVE('',#9336,#9325,#614,.T.);
#11570=EDGE_CURVE('',#9337,#9338,#5582,.T.);
#11571=EDGE_CURVE('',#9337,#9339,#5583,.T.);
#11572=EDGE_CURVE('',#9339,#9340,#5584,.T.);
#11573=EDGE_CURVE('',#9338,#9340,#5585,.T.);
#11574=EDGE_CURVE('',#9341,#9337,#5586,.T.);
#11575=EDGE_CURVE('',#9341,#9342,#5587,.T.);
#11576=EDGE_CURVE('',#9342,#9339,#5588,.T.);
#11577=EDGE_CURVE('',#9343,#9341,#5589,.T.);
#11578=EDGE_CURVE('',#9343,#9344,#5590,.T.);
#11579=EDGE_CURVE('',#9344,#9342,#5591,.T.);
#11580=EDGE_CURVE('',#9345,#9343,#5592,.T.);
#11581=EDGE_CURVE('',#9345,#9346,#5593,.T.);
#11582=EDGE_CURVE('',#9346,#9344,#5594,.T.);
#11583=EDGE_CURVE('',#9347,#9345,#5595,.T.);
#11584=EDGE_CURVE('',#9347,#9348,#5596,.T.);
#11585=EDGE_CURVE('',#9348,#9346,#5597,.T.);
#11586=EDGE_CURVE('',#9338,#9347,#5598,.T.);
#11587=EDGE_CURVE('',#9340,#9348,#5599,.T.);
#11588=EDGE_CURVE('',#9349,#9350,#5600,.T.);
#11589=EDGE_CURVE('',#9349,#9351,#5601,.T.);
#11590=EDGE_CURVE('',#9352,#9351,#5602,.T.);
#11591=EDGE_CURVE('',#9350,#9352,#5603,.T.);
#11592=EDGE_CURVE('',#9350,#9353,#8451,.T.);
#11593=EDGE_CURVE('',#9352,#9353,#5604,.T.);
#11594=EDGE_CURVE('',#9353,#9354,#5605,.T.);
#11595=EDGE_CURVE('',#9351,#9354,#5606,.T.);
#11596=EDGE_CURVE('',#9354,#9349,#8452,.T.);
#11597=EDGE_CURVE('',#9355,#9356,#5607,.T.);
#11598=EDGE_CURVE('',#9355,#9357,#5608,.T.);
#11599=EDGE_CURVE('',#9358,#9357,#5609,.T.);
#11600=EDGE_CURVE('',#9356,#9358,#5610,.T.);
#11601=EDGE_CURVE('',#9356,#9359,#8453,.T.);
#11602=EDGE_CURVE('',#9358,#9359,#5611,.T.);
#11603=EDGE_CURVE('',#9359,#9360,#5612,.T.);
#11604=EDGE_CURVE('',#9357,#9360,#5613,.T.);
#11605=EDGE_CURVE('',#9360,#9355,#8454,.T.);
#11606=EDGE_CURVE('',#9361,#9362,#5614,.T.);
#11607=EDGE_CURVE('',#9361,#9363,#5615,.T.);
#11608=EDGE_CURVE('',#9364,#9363,#5616,.T.);
#11609=EDGE_CURVE('',#9362,#9364,#5617,.T.);
#11610=EDGE_CURVE('',#9362,#9365,#8455,.T.);
#11611=EDGE_CURVE('',#9364,#9365,#5618,.T.);
#11612=EDGE_CURVE('',#9365,#9366,#5619,.T.);
#11613=EDGE_CURVE('',#9363,#9366,#5620,.T.);
#11614=EDGE_CURVE('',#9366,#9361,#8456,.T.);
#11615=EDGE_CURVE('',#9367,#9368,#5621,.T.);
#11616=EDGE_CURVE('',#9367,#9369,#5622,.T.);
#11617=EDGE_CURVE('',#9370,#9369,#5623,.T.);
#11618=EDGE_CURVE('',#9368,#9370,#5624,.T.);
#11619=EDGE_CURVE('',#9368,#9371,#8457,.T.);
#11620=EDGE_CURVE('',#9370,#9371,#5625,.T.);
#11621=EDGE_CURVE('',#9371,#9372,#5626,.T.);
#11622=EDGE_CURVE('',#9369,#9372,#5627,.T.);
#11623=EDGE_CURVE('',#9372,#9367,#8458,.T.);
#11624=EDGE_CURVE('',#9373,#9374,#5628,.T.);
#11625=EDGE_CURVE('',#9373,#9375,#5629,.T.);
#11626=EDGE_CURVE('',#9376,#9375,#5630,.T.);
#11627=EDGE_CURVE('',#9374,#9376,#5631,.T.);
#11628=EDGE_CURVE('',#9374,#9377,#8459,.T.);
#11629=EDGE_CURVE('',#9376,#9377,#5632,.T.);
#11630=EDGE_CURVE('',#9377,#9378,#5633,.T.);
#11631=EDGE_CURVE('',#9375,#9378,#5634,.T.);
#11632=EDGE_CURVE('',#9378,#9373,#8460,.T.);
#11633=EDGE_CURVE('',#9379,#9380,#5635,.T.);
#11634=EDGE_CURVE('',#9379,#9381,#5636,.T.);
#11635=EDGE_CURVE('',#9382,#9381,#5637,.T.);
#11636=EDGE_CURVE('',#9380,#9382,#5638,.T.);
#11637=EDGE_CURVE('',#9380,#9383,#8461,.T.);
#11638=EDGE_CURVE('',#9382,#9383,#5639,.T.);
#11639=EDGE_CURVE('',#9383,#9384,#5640,.T.);
#11640=EDGE_CURVE('',#9381,#9384,#5641,.T.);
#11641=EDGE_CURVE('',#9384,#9379,#8462,.T.);
#11642=EDGE_CURVE('',#9385,#9386,#5642,.T.);
#11643=EDGE_CURVE('',#9385,#9387,#5643,.T.);
#11644=EDGE_CURVE('',#9388,#9387,#5644,.T.);
#11645=EDGE_CURVE('',#9386,#9388,#5645,.T.);
#11646=EDGE_CURVE('',#9386,#9389,#8463,.T.);
#11647=EDGE_CURVE('',#9388,#9389,#5646,.T.);
#11648=EDGE_CURVE('',#9389,#9390,#5647,.T.);
#11649=EDGE_CURVE('',#9387,#9390,#5648,.T.);
#11650=EDGE_CURVE('',#9390,#9385,#8464,.T.);
#11651=EDGE_CURVE('',#9391,#9392,#8465,.T.);
#11652=EDGE_CURVE('',#9391,#9393,#5649,.T.);
#11653=EDGE_CURVE('',#9393,#9392,#5650,.T.);
#11654=EDGE_CURVE('',#9394,#9391,#5651,.T.);
#11655=EDGE_CURVE('',#9394,#9395,#5652,.T.);
#11656=EDGE_CURVE('',#9393,#9395,#5653,.T.);
#11657=EDGE_CURVE('',#9392,#9396,#5654,.T.);
#11658=EDGE_CURVE('',#9395,#9396,#5655,.T.);
#11659=EDGE_CURVE('',#9396,#9394,#8466,.T.);
#11660=EDGE_CURVE('',#9397,#9398,#5656,.T.);
#11661=EDGE_CURVE('',#9397,#9399,#5657,.T.);
#11662=EDGE_CURVE('',#9400,#9399,#5658,.T.);
#11663=EDGE_CURVE('',#9398,#9400,#5659,.T.);
#11664=EDGE_CURVE('',#9398,#9401,#8467,.T.);
#11665=EDGE_CURVE('',#9400,#9401,#5660,.T.);
#11666=EDGE_CURVE('',#9401,#9402,#5661,.T.);
#11667=EDGE_CURVE('',#9399,#9402,#5662,.T.);
#11668=EDGE_CURVE('',#9402,#9397,#8468,.T.);
#11669=EDGE_CURVE('',#9403,#9404,#5663,.T.);
#11670=EDGE_CURVE('',#9403,#9405,#5664,.T.);
#11671=EDGE_CURVE('',#9406,#9405,#5665,.T.);
#11672=EDGE_CURVE('',#9404,#9406,#5666,.T.);
#11673=EDGE_CURVE('',#9404,#9407,#8469,.T.);
#11674=EDGE_CURVE('',#9406,#9407,#5667,.T.);
#11675=EDGE_CURVE('',#9407,#9408,#5668,.T.);
#11676=EDGE_CURVE('',#9405,#9408,#5669,.T.);
#11677=EDGE_CURVE('',#9408,#9403,#8470,.T.);
#11678=EDGE_CURVE('',#9409,#9410,#5670,.T.);
#11679=EDGE_CURVE('',#9409,#9411,#5671,.T.);
#11680=EDGE_CURVE('',#9412,#9411,#5672,.T.);
#11681=EDGE_CURVE('',#9410,#9412,#5673,.T.);
#11682=EDGE_CURVE('',#9410,#9413,#8471,.T.);
#11683=EDGE_CURVE('',#9412,#9413,#5674,.T.);
#11684=EDGE_CURVE('',#9413,#9414,#5675,.T.);
#11685=EDGE_CURVE('',#9411,#9414,#5676,.T.);
#11686=EDGE_CURVE('',#9414,#9409,#8472,.T.);
#11687=EDGE_CURVE('',#9415,#9416,#5677,.T.);
#11688=EDGE_CURVE('',#9415,#9417,#5678,.T.);
#11689=EDGE_CURVE('',#9418,#9417,#5679,.T.);
#11690=EDGE_CURVE('',#9416,#9418,#5680,.T.);
#11691=EDGE_CURVE('',#9416,#9419,#8473,.T.);
#11692=EDGE_CURVE('',#9418,#9419,#5681,.T.);
#11693=EDGE_CURVE('',#9419,#9420,#5682,.T.);
#11694=EDGE_CURVE('',#9417,#9420,#5683,.T.);
#11695=EDGE_CURVE('',#9420,#9415,#8474,.T.);
#11696=EDGE_CURVE('',#9421,#9422,#5684,.T.);
#11697=EDGE_CURVE('',#9421,#9423,#5685,.T.);
#11698=EDGE_CURVE('',#9424,#9423,#5686,.T.);
#11699=EDGE_CURVE('',#9422,#9424,#5687,.T.);
#11700=EDGE_CURVE('',#9422,#9425,#8475,.T.);
#11701=EDGE_CURVE('',#9424,#9425,#5688,.T.);
#11702=EDGE_CURVE('',#9425,#9426,#5689,.T.);
#11703=EDGE_CURVE('',#9423,#9426,#5690,.T.);
#11704=EDGE_CURVE('',#9426,#9421,#8476,.T.);
#11705=EDGE_CURVE('',#9427,#9428,#5691,.T.);
#11706=EDGE_CURVE('',#9427,#9429,#5692,.T.);
#11707=EDGE_CURVE('',#9430,#9429,#5693,.T.);
#11708=EDGE_CURVE('',#9428,#9430,#5694,.T.);
#11709=EDGE_CURVE('',#9428,#9431,#8477,.T.);
#11710=EDGE_CURVE('',#9430,#9431,#5695,.T.);
#11711=EDGE_CURVE('',#9431,#9432,#5696,.T.);
#11712=EDGE_CURVE('',#9429,#9432,#5697,.T.);
#11713=EDGE_CURVE('',#9432,#9427,#8478,.T.);
#11714=EDGE_CURVE('',#9433,#9434,#5698,.T.);
#11715=EDGE_CURVE('',#9433,#9435,#5699,.T.);
#11716=EDGE_CURVE('',#9436,#9435,#5700,.T.);
#11717=EDGE_CURVE('',#9434,#9436,#5701,.T.);
#11718=EDGE_CURVE('',#9434,#9437,#8479,.T.);
#11719=EDGE_CURVE('',#9436,#9437,#5702,.T.);
#11720=EDGE_CURVE('',#9437,#9438,#5703,.T.);
#11721=EDGE_CURVE('',#9435,#9438,#5704,.T.);
#11722=EDGE_CURVE('',#9438,#9433,#8480,.T.);
#11723=EDGE_CURVE('',#9439,#9440,#5705,.T.);
#11724=EDGE_CURVE('',#9439,#9441,#5706,.T.);
#11725=EDGE_CURVE('',#9442,#9441,#5707,.T.);
#11726=EDGE_CURVE('',#9440,#9442,#5708,.T.);
#11727=EDGE_CURVE('',#9440,#9443,#8481,.T.);
#11728=EDGE_CURVE('',#9442,#9443,#5709,.T.);
#11729=EDGE_CURVE('',#9443,#9444,#5710,.T.);
#11730=EDGE_CURVE('',#9441,#9444,#5711,.T.);
#11731=EDGE_CURVE('',#9444,#9439,#8482,.T.);
#11732=EDGE_CURVE('',#9445,#9446,#5712,.T.);
#11733=EDGE_CURVE('',#9445,#9447,#5713,.T.);
#11734=EDGE_CURVE('',#9448,#9447,#5714,.T.);
#11735=EDGE_CURVE('',#9446,#9448,#5715,.T.);
#11736=EDGE_CURVE('',#9446,#9449,#8483,.T.);
#11737=EDGE_CURVE('',#9448,#9449,#5716,.T.);
#11738=EDGE_CURVE('',#9449,#9450,#5717,.T.);
#11739=EDGE_CURVE('',#9447,#9450,#5718,.T.);
#11740=EDGE_CURVE('',#9450,#9445,#8484,.T.);
#11741=EDGE_CURVE('',#9451,#9452,#5719,.T.);
#11742=EDGE_CURVE('',#9451,#9453,#5720,.T.);
#11743=EDGE_CURVE('',#9454,#9453,#5721,.T.);
#11744=EDGE_CURVE('',#9452,#9454,#5722,.T.);
#11745=EDGE_CURVE('',#9452,#9455,#8485,.T.);
#11746=EDGE_CURVE('',#9454,#9455,#5723,.T.);
#11747=EDGE_CURVE('',#9455,#9456,#5724,.T.);
#11748=EDGE_CURVE('',#9453,#9456,#5725,.T.);
#11749=EDGE_CURVE('',#9456,#9451,#8486,.T.);
#11750=EDGE_CURVE('',#9457,#9458,#5726,.T.);
#11751=EDGE_CURVE('',#9457,#9459,#5727,.T.);
#11752=EDGE_CURVE('',#9460,#9459,#5728,.T.);
#11753=EDGE_CURVE('',#9458,#9460,#5729,.T.);
#11754=EDGE_CURVE('',#9458,#9461,#8487,.T.);
#11755=EDGE_CURVE('',#9460,#9461,#5730,.T.);
#11756=EDGE_CURVE('',#9461,#9462,#5731,.T.);
#11757=EDGE_CURVE('',#9459,#9462,#5732,.T.);
#11758=EDGE_CURVE('',#9462,#9457,#8488,.T.);
#11759=EDGE_CURVE('',#9463,#9464,#5733,.T.);
#11760=EDGE_CURVE('',#9463,#9465,#5734,.T.);
#11761=EDGE_CURVE('',#9466,#9465,#5735,.T.);
#11762=EDGE_CURVE('',#9464,#9466,#5736,.T.);
#11763=EDGE_CURVE('',#9464,#9467,#8489,.T.);
#11764=EDGE_CURVE('',#9466,#9467,#5737,.T.);
#11765=EDGE_CURVE('',#9467,#9468,#5738,.T.);
#11766=EDGE_CURVE('',#9465,#9468,#5739,.T.);
#11767=EDGE_CURVE('',#9468,#9463,#8490,.T.);
#11768=EDGE_CURVE('',#9469,#9470,#5740,.T.);
#11769=EDGE_CURVE('',#9469,#9471,#5741,.T.);
#11770=EDGE_CURVE('',#9472,#9471,#5742,.T.);
#11771=EDGE_CURVE('',#9470,#9472,#5743,.T.);
#11772=EDGE_CURVE('',#9470,#9473,#8491,.T.);
#11773=EDGE_CURVE('',#9472,#9473,#5744,.T.);
#11774=EDGE_CURVE('',#9473,#9474,#5745,.T.);
#11775=EDGE_CURVE('',#9471,#9474,#5746,.T.);
#11776=EDGE_CURVE('',#9474,#9469,#8492,.T.);
#11777=EDGE_CURVE('',#9475,#9476,#5747,.T.);
#11778=EDGE_CURVE('',#9475,#9477,#5748,.T.);
#11779=EDGE_CURVE('',#9478,#9477,#5749,.T.);
#11780=EDGE_CURVE('',#9476,#9478,#5750,.T.);
#11781=EDGE_CURVE('',#9476,#9479,#8493,.T.);
#11782=EDGE_CURVE('',#9478,#9479,#5751,.T.);
#11783=EDGE_CURVE('',#9479,#9480,#5752,.T.);
#11784=EDGE_CURVE('',#9477,#9480,#5753,.T.);
#11785=EDGE_CURVE('',#9480,#9475,#8494,.T.);
#11786=EDGE_CURVE('',#9481,#9482,#5754,.T.);
#11787=EDGE_CURVE('',#9481,#9483,#5755,.T.);
#11788=EDGE_CURVE('',#9484,#9483,#5756,.T.);
#11789=EDGE_CURVE('',#9482,#9484,#5757,.T.);
#11790=EDGE_CURVE('',#9482,#9485,#8495,.T.);
#11791=EDGE_CURVE('',#9484,#9486,#5758,.T.);
#11792=EDGE_CURVE('',#9485,#9486,#8496,.T.);
#11793=EDGE_CURVE('',#9486,#9487,#5759,.T.);
#11794=EDGE_CURVE('',#9483,#9487,#5760,.T.);
#11795=EDGE_CURVE('',#9487,#9488,#8497,.T.);
#11796=EDGE_CURVE('',#9488,#9481,#8498,.T.);
#11797=EDGE_CURVE('',#9489,#9490,#5761,.T.);
#11798=EDGE_CURVE('',#9489,#9491,#5762,.T.);
#11799=EDGE_CURVE('',#9492,#9491,#5763,.T.);
#11800=EDGE_CURVE('',#9490,#9492,#5764,.T.);
#11801=EDGE_CURVE('',#9490,#9493,#8499,.T.);
#11802=EDGE_CURVE('',#9492,#9493,#5765,.T.);
#11803=EDGE_CURVE('',#9493,#9494,#5766,.T.);
#11804=EDGE_CURVE('',#9491,#9494,#5767,.T.);
#11805=EDGE_CURVE('',#9494,#9489,#8500,.T.);
#11806=EDGE_CURVE('',#9495,#9496,#5768,.T.);
#11807=EDGE_CURVE('',#9495,#9497,#5769,.T.);
#11808=EDGE_CURVE('',#9498,#9497,#5770,.T.);
#11809=EDGE_CURVE('',#9496,#9498,#5771,.T.);
#11810=EDGE_CURVE('',#9496,#9499,#8501,.T.);
#11811=EDGE_CURVE('',#9498,#9499,#5772,.T.);
#11812=EDGE_CURVE('',#9499,#9500,#5773,.T.);
#11813=EDGE_CURVE('',#9497,#9500,#5774,.T.);
#11814=EDGE_CURVE('',#9500,#9495,#8502,.T.);
#11815=EDGE_CURVE('',#9501,#9502,#5775,.T.);
#11816=EDGE_CURVE('',#9501,#9503,#5776,.T.);
#11817=EDGE_CURVE('',#9504,#9503,#5777,.T.);
#11818=EDGE_CURVE('',#9502,#9504,#5778,.T.);
#11819=EDGE_CURVE('',#9502,#9505,#8503,.T.);
#11820=EDGE_CURVE('',#9504,#9505,#5779,.T.);
#11821=EDGE_CURVE('',#9505,#9506,#5780,.T.);
#11822=EDGE_CURVE('',#9503,#9506,#5781,.T.);
#11823=EDGE_CURVE('',#9506,#9501,#8504,.T.);
#11824=EDGE_CURVE('',#9507,#9508,#5782,.T.);
#11825=EDGE_CURVE('',#9507,#9509,#5783,.T.);
#11826=EDGE_CURVE('',#9510,#9509,#5784,.T.);
#11827=EDGE_CURVE('',#9508,#9510,#5785,.T.);
#11828=EDGE_CURVE('',#9508,#9511,#8505,.T.);
#11829=EDGE_CURVE('',#9510,#9511,#5786,.T.);
#11830=EDGE_CURVE('',#9511,#9512,#5787,.T.);
#11831=EDGE_CURVE('',#9509,#9512,#5788,.T.);
#11832=EDGE_CURVE('',#9512,#9507,#8506,.T.);
#11833=EDGE_CURVE('',#9513,#9514,#5789,.T.);
#11834=EDGE_CURVE('',#9513,#9515,#5790,.T.);
#11835=EDGE_CURVE('',#9516,#9515,#5791,.T.);
#11836=EDGE_CURVE('',#9514,#9516,#5792,.T.);
#11837=EDGE_CURVE('',#9514,#9517,#8507,.T.);
#11838=EDGE_CURVE('',#9516,#9517,#5793,.T.);
#11839=EDGE_CURVE('',#9517,#9518,#5794,.T.);
#11840=EDGE_CURVE('',#9515,#9518,#5795,.T.);
#11841=EDGE_CURVE('',#9518,#9513,#8508,.T.);
#11842=EDGE_CURVE('',#9519,#9520,#5796,.T.);
#11843=EDGE_CURVE('',#9519,#9521,#5797,.T.);
#11844=EDGE_CURVE('',#9522,#9521,#5798,.T.);
#11845=EDGE_CURVE('',#9520,#9522,#5799,.T.);
#11846=EDGE_CURVE('',#9520,#9523,#8509,.T.);
#11847=EDGE_CURVE('',#9522,#9523,#5800,.T.);
#11848=EDGE_CURVE('',#9523,#9524,#5801,.T.);
#11849=EDGE_CURVE('',#9521,#9524,#5802,.T.);
#11850=EDGE_CURVE('',#9524,#9519,#8510,.T.);
#11851=EDGE_CURVE('',#9525,#9526,#5803,.T.);
#11852=EDGE_CURVE('',#9525,#9527,#5804,.T.);
#11853=EDGE_CURVE('',#9528,#9527,#5805,.T.);
#11854=EDGE_CURVE('',#9526,#9528,#5806,.T.);
#11855=EDGE_CURVE('',#9526,#9529,#8511,.T.);
#11856=EDGE_CURVE('',#9528,#9529,#5807,.T.);
#11857=EDGE_CURVE('',#9529,#9530,#5808,.T.);
#11858=EDGE_CURVE('',#9527,#9530,#5809,.T.);
#11859=EDGE_CURVE('',#9530,#9525,#8512,.T.);
#11860=EDGE_CURVE('',#9531,#9531,#8513,.T.);
#11861=EDGE_CURVE('',#9531,#9532,#5810,.T.);
#11862=EDGE_CURVE('',#9533,#9532,#1454,.T.);
#11863=EDGE_CURVE('',#9534,#9533,#1455,.T.);
#11864=EDGE_CURVE('',#9535,#9534,#1456,.T.);
#11865=EDGE_CURVE('',#9536,#9535,#1457,.T.);
#11866=EDGE_CURVE('',#9537,#9536,#1458,.T.);
#11867=EDGE_CURVE('',#9538,#9537,#1459,.T.);
#11868=EDGE_CURVE('',#9532,#9538,#1460,.T.);
#11869=EDGE_CURVE('',#9536,#9539,#5811,.T.);
#11870=EDGE_CURVE('',#9539,#9540,#1461,.T.);
#11871=EDGE_CURVE('',#9537,#9540,#5812,.T.);
#11872=EDGE_CURVE('',#9535,#9541,#5813,.T.);
#11873=EDGE_CURVE('',#9541,#9539,#1462,.T.);
#11874=EDGE_CURVE('',#9534,#9542,#5814,.T.);
#11875=EDGE_CURVE('',#9542,#9541,#1463,.T.);
#11876=EDGE_CURVE('',#9543,#9542,#1464,.T.);
#11877=EDGE_CURVE('',#9544,#9543,#1465,.T.);
#11878=EDGE_CURVE('',#9544,#9545,#5815,.T.);
#11879=EDGE_CURVE('',#9545,#9545,#8514,.T.);
#11880=EDGE_CURVE('',#9546,#9544,#1466,.T.);
#11881=EDGE_CURVE('',#9540,#9546,#1467,.T.);
#11882=EDGE_CURVE('',#9533,#9543,#5816,.T.);
#11883=EDGE_CURVE('',#9547,#9547,#8515,.T.);
#11884=EDGE_CURVE('',#9548,#9548,#8516,.T.);
#11885=EDGE_CURVE('',#9538,#9546,#5817,.T.);
#11886=EDGE_CURVE('',#9549,#9549,#8517,.T.);
#11887=EDGE_CURVE('',#9549,#9550,#5818,.T.);
#11888=EDGE_CURVE('',#9550,#9550,#8518,.T.);
#11889=EDGE_CURVE('',#9550,#9551,#5819,.T.);
#11890=EDGE_CURVE('',#9552,#9552,#8519,.T.);
#11891=EDGE_CURVE('',#9332,#9552,#5820,.T.);
#11892=EDGE_CURVE('',#9553,#9553,#8520,.T.);
#11893=EDGE_CURVE('',#9548,#9553,#5821,.T.);
#11894=EDGE_CURVE('',#9523,#9350,#8521,.T.);
#11895=EDGE_CURVE('',#9359,#9520,#8522,.T.);
#11896=EDGE_CURVE('',#9517,#9356,#8523,.T.);
#11897=EDGE_CURVE('',#9365,#9514,#8524,.T.);
#11898=EDGE_CURVE('',#9511,#9362,#8525,.T.);
#11899=EDGE_CURVE('',#9371,#9508,#8526,.T.);
#11900=EDGE_CURVE('',#9505,#9368,#8527,.T.);
#11901=EDGE_CURVE('',#9377,#9502,#8528,.T.);
#11902=EDGE_CURVE('',#9499,#9374,#8529,.T.);
#11903=EDGE_CURVE('',#9383,#9496,#8530,.T.);
#11904=EDGE_CURVE('',#9493,#9380,#8531,.T.);
#11905=EDGE_CURVE('',#9389,#9490,#8532,.T.);
#11906=EDGE_CURVE('',#9486,#9386,#8533,.T.);
#11907=EDGE_CURVE('',#9488,#9547,#5822,.T.);
#11908=EDGE_CURVE('',#9479,#9482,#8534,.T.);
#11909=EDGE_CURVE('',#9401,#9476,#8535,.T.);
#11910=EDGE_CURVE('',#9473,#9398,#8536,.T.);
#11911=EDGE_CURVE('',#9407,#9470,#8537,.T.);
#11912=EDGE_CURVE('',#9467,#9404,#8538,.T.);
#11913=EDGE_CURVE('',#9413,#9464,#8539,.T.);
#11914=EDGE_CURVE('',#9461,#9410,#8540,.T.);
#11915=EDGE_CURVE('',#9419,#9458,#8541,.T.);
#11916=EDGE_CURVE('',#9455,#9416,#8542,.T.);
#11917=EDGE_CURVE('',#9425,#9452,#8543,.T.);
#11918=EDGE_CURVE('',#9449,#9422,#8544,.T.);
#11919=EDGE_CURVE('',#9431,#9446,#8545,.T.);
#11920=EDGE_CURVE('',#9443,#9428,#8546,.T.);
#11921=EDGE_CURVE('',#9437,#9440,#8547,.T.);
#11922=EDGE_CURVE('',#9392,#9434,#8548,.T.);
#11923=EDGE_CURVE('',#9529,#9391,#8549,.T.);
#11924=EDGE_CURVE('',#9353,#9526,#8550,.T.);
#11925=EDGE_CURVE('',#9554,#9554,#8551,.T.);
#11926=EDGE_CURVE('',#9554,#9485,#5823,.T.);
#15038=ORIENTED_EDGE('',*,*,#11523,.F.);
#15039=ORIENTED_EDGE('',*,*,#11524,.T.);
#15040=ORIENTED_EDGE('',*,*,#11525,.F.);
#15041=ORIENTED_EDGE('',*,*,#11526,.F.);
#15042=ORIENTED_EDGE('',*,*,#11527,.F.);
#15043=ORIENTED_EDGE('',*,*,#11528,.T.);
#15044=ORIENTED_EDGE('',*,*,#11523,.T.);
#15045=ORIENTED_EDGE('',*,*,#11529,.F.);
#15046=ORIENTED_EDGE('',*,*,#11530,.F.);
#15047=ORIENTED_EDGE('',*,*,#11531,.T.);
#15048=ORIENTED_EDGE('',*,*,#11527,.T.);
#15049=ORIENTED_EDGE('',*,*,#11532,.F.);
#15050=ORIENTED_EDGE('',*,*,#11533,.F.);
#15051=ORIENTED_EDGE('',*,*,#11534,.T.);
#15052=ORIENTED_EDGE('',*,*,#11530,.T.);
#15053=ORIENTED_EDGE('',*,*,#11535,.F.);
#15054=ORIENTED_EDGE('',*,*,#11536,.F.);
#15055=ORIENTED_EDGE('',*,*,#11537,.T.);
#15056=ORIENTED_EDGE('',*,*,#11533,.T.);
#15057=ORIENTED_EDGE('',*,*,#11538,.F.);
#15058=ORIENTED_EDGE('',*,*,#11539,.F.);
#15059=ORIENTED_EDGE('',*,*,#11540,.T.);
#15060=ORIENTED_EDGE('',*,*,#11536,.T.);
#15061=ORIENTED_EDGE('',*,*,#11541,.F.);
#15062=ORIENTED_EDGE('',*,*,#11542,.F.);
#15063=ORIENTED_EDGE('',*,*,#11543,.T.);
#15064=ORIENTED_EDGE('',*,*,#11539,.T.);
#15065=ORIENTED_EDGE('',*,*,#11544,.F.);
#15066=ORIENTED_EDGE('',*,*,#11545,.F.);
#15067=ORIENTED_EDGE('',*,*,#11546,.F.);
#15068=ORIENTED_EDGE('',*,*,#11547,.T.);
#15069=ORIENTED_EDGE('',*,*,#11542,.T.);
#15070=ORIENTED_EDGE('',*,*,#11548,.F.);
#15071=ORIENTED_EDGE('',*,*,#11549,.F.);
#15072=ORIENTED_EDGE('',*,*,#11550,.F.);
#15073=ORIENTED_EDGE('',*,*,#11551,.F.);
#15074=ORIENTED_EDGE('',*,*,#11552,.T.);
#15075=ORIENTED_EDGE('',*,*,#11553,.F.);
#15076=ORIENTED_EDGE('',*,*,#11552,.F.);
#15077=ORIENTED_EDGE('',*,*,#11554,.F.);
#15078=ORIENTED_EDGE('',*,*,#11555,.T.);
#15079=ORIENTED_EDGE('',*,*,#11556,.F.);
#15080=ORIENTED_EDGE('',*,*,#11555,.F.);
#15081=ORIENTED_EDGE('',*,*,#11557,.F.);
#15082=ORIENTED_EDGE('',*,*,#11558,.T.);
#15083=ORIENTED_EDGE('',*,*,#11548,.T.);
#15084=ORIENTED_EDGE('',*,*,#11544,.T.);
#15085=ORIENTED_EDGE('',*,*,#11541,.T.);
#15086=ORIENTED_EDGE('',*,*,#11538,.T.);
#15087=ORIENTED_EDGE('',*,*,#11535,.T.);
#15088=ORIENTED_EDGE('',*,*,#11532,.T.);
#15089=ORIENTED_EDGE('',*,*,#11529,.T.);
#15090=ORIENTED_EDGE('',*,*,#11526,.T.);
#15091=ORIENTED_EDGE('',*,*,#11559,.T.);
#15092=ORIENTED_EDGE('',*,*,#11560,.T.);
#15093=ORIENTED_EDGE('',*,*,#11561,.T.);
#15094=ORIENTED_EDGE('',*,*,#11562,.T.);
#15095=ORIENTED_EDGE('',*,*,#11563,.T.);
#15096=ORIENTED_EDGE('',*,*,#11546,.T.);
#15097=ORIENTED_EDGE('',*,*,#11564,.T.);
#15098=ORIENTED_EDGE('',*,*,#11557,.T.);
#15099=ORIENTED_EDGE('',*,*,#11554,.T.);
#15100=ORIENTED_EDGE('',*,*,#11551,.T.);
#15101=ORIENTED_EDGE('',*,*,#11545,.T.);
#15102=ORIENTED_EDGE('',*,*,#11558,.F.);
#15103=ORIENTED_EDGE('',*,*,#11564,.F.);
#15104=ORIENTED_EDGE('',*,*,#11565,.F.);
#15105=ORIENTED_EDGE('',*,*,#11524,.F.);
#15106=ORIENTED_EDGE('',*,*,#11528,.F.);
#15107=ORIENTED_EDGE('',*,*,#11531,.F.);
#15108=ORIENTED_EDGE('',*,*,#11534,.F.);
#15109=ORIENTED_EDGE('',*,*,#11537,.F.);
#15110=ORIENTED_EDGE('',*,*,#11540,.F.);
#15111=ORIENTED_EDGE('',*,*,#11543,.F.);
#15112=ORIENTED_EDGE('',*,*,#11547,.F.);
#15113=ORIENTED_EDGE('',*,*,#11563,.F.);
#15114=ORIENTED_EDGE('',*,*,#11566,.T.);
#15115=ORIENTED_EDGE('',*,*,#11567,.F.);
#15116=ORIENTED_EDGE('',*,*,#11566,.F.);
#15117=ORIENTED_EDGE('',*,*,#11562,.F.);
#15118=ORIENTED_EDGE('',*,*,#11568,.T.);
#15119=ORIENTED_EDGE('',*,*,#11569,.F.);
#15120=ORIENTED_EDGE('',*,*,#11568,.F.);
#15121=ORIENTED_EDGE('',*,*,#11561,.F.);
#15122=ORIENTED_EDGE('',*,*,#11550,.T.);
#15123=ORIENTED_EDGE('',*,*,#11570,.F.);
#15124=ORIENTED_EDGE('',*,*,#11571,.T.);
#15125=ORIENTED_EDGE('',*,*,#11572,.T.);
#15126=ORIENTED_EDGE('',*,*,#11573,.F.);
#15127=ORIENTED_EDGE('',*,*,#11574,.F.);
#15128=ORIENTED_EDGE('',*,*,#11575,.T.);
#15129=ORIENTED_EDGE('',*,*,#11576,.T.);
#15130=ORIENTED_EDGE('',*,*,#11571,.F.);
#15131=ORIENTED_EDGE('',*,*,#11577,.F.);
#15132=ORIENTED_EDGE('',*,*,#11578,.T.);
#15133=ORIENTED_EDGE('',*,*,#11579,.T.);
#15134=ORIENTED_EDGE('',*,*,#11575,.F.);
#15135=ORIENTED_EDGE('',*,*,#11580,.F.);
#15136=ORIENTED_EDGE('',*,*,#11581,.T.);
#15137=ORIENTED_EDGE('',*,*,#11582,.T.);
#15138=ORIENTED_EDGE('',*,*,#11578,.F.);
#15139=ORIENTED_EDGE('',*,*,#11583,.F.);
#15140=ORIENTED_EDGE('',*,*,#11584,.T.);
#15141=ORIENTED_EDGE('',*,*,#11585,.T.);
#15142=ORIENTED_EDGE('',*,*,#11581,.F.);
#15143=ORIENTED_EDGE('',*,*,#11586,.F.);
#15144=ORIENTED_EDGE('',*,*,#11573,.T.);
#15145=ORIENTED_EDGE('',*,*,#11587,.T.);
#15146=ORIENTED_EDGE('',*,*,#11584,.F.);
#15147=ORIENTED_EDGE('',*,*,#11587,.F.);
#15148=ORIENTED_EDGE('',*,*,#11572,.F.);
#15149=ORIENTED_EDGE('',*,*,#11576,.F.);
#15150=ORIENTED_EDGE('',*,*,#11579,.F.);
#15151=ORIENTED_EDGE('',*,*,#11582,.F.);
#15152=ORIENTED_EDGE('',*,*,#11585,.F.);
#15153=ORIENTED_EDGE('',*,*,#11588,.F.);
#15154=ORIENTED_EDGE('',*,*,#11589,.T.);
#15155=ORIENTED_EDGE('',*,*,#11590,.F.);
#15156=ORIENTED_EDGE('',*,*,#11591,.F.);
#15157=ORIENTED_EDGE('',*,*,#11592,.F.);
#15158=ORIENTED_EDGE('',*,*,#11591,.T.);
#15159=ORIENTED_EDGE('',*,*,#11593,.T.);
#15160=ORIENTED_EDGE('',*,*,#11594,.F.);
#15161=ORIENTED_EDGE('',*,*,#11593,.F.);
#15162=ORIENTED_EDGE('',*,*,#11590,.T.);
#15163=ORIENTED_EDGE('',*,*,#11595,.T.);
#15164=ORIENTED_EDGE('',*,*,#11596,.F.);
#15165=ORIENTED_EDGE('',*,*,#11595,.F.);
#15166=ORIENTED_EDGE('',*,*,#11589,.F.);
#15167=ORIENTED_EDGE('',*,*,#11597,.F.);
#15168=ORIENTED_EDGE('',*,*,#11598,.T.);
#15169=ORIENTED_EDGE('',*,*,#11599,.F.);
#15170=ORIENTED_EDGE('',*,*,#11600,.F.);
#15171=ORIENTED_EDGE('',*,*,#11601,.F.);
#15172=ORIENTED_EDGE('',*,*,#11600,.T.);
#15173=ORIENTED_EDGE('',*,*,#11602,.T.);
#15174=ORIENTED_EDGE('',*,*,#11603,.F.);
#15175=ORIENTED_EDGE('',*,*,#11602,.F.);
#15176=ORIENTED_EDGE('',*,*,#11599,.T.);
#15177=ORIENTED_EDGE('',*,*,#11604,.T.);
#15178=ORIENTED_EDGE('',*,*,#11605,.F.);
#15179=ORIENTED_EDGE('',*,*,#11604,.F.);
#15180=ORIENTED_EDGE('',*,*,#11598,.F.);
#15181=ORIENTED_EDGE('',*,*,#11606,.F.);
#15182=ORIENTED_EDGE('',*,*,#11607,.T.);
#15183=ORIENTED_EDGE('',*,*,#11608,.F.);
#15184=ORIENTED_EDGE('',*,*,#11609,.F.);
#15185=ORIENTED_EDGE('',*,*,#11610,.F.);
#15186=ORIENTED_EDGE('',*,*,#11609,.T.);
#15187=ORIENTED_EDGE('',*,*,#11611,.T.);
#15188=ORIENTED_EDGE('',*,*,#11612,.F.);
#15189=ORIENTED_EDGE('',*,*,#11611,.F.);
#15190=ORIENTED_EDGE('',*,*,#11608,.T.);
#15191=ORIENTED_EDGE('',*,*,#11613,.T.);
#15192=ORIENTED_EDGE('',*,*,#11614,.F.);
#15193=ORIENTED_EDGE('',*,*,#11613,.F.);
#15194=ORIENTED_EDGE('',*,*,#11607,.F.);
#15195=ORIENTED_EDGE('',*,*,#11615,.F.);
#15196=ORIENTED_EDGE('',*,*,#11616,.T.);
#15197=ORIENTED_EDGE('',*,*,#11617,.F.);
#15198=ORIENTED_EDGE('',*,*,#11618,.F.);
#15199=ORIENTED_EDGE('',*,*,#11619,.F.);
#15200=ORIENTED_EDGE('',*,*,#11618,.T.);
#15201=ORIENTED_EDGE('',*,*,#11620,.T.);
#15202=ORIENTED_EDGE('',*,*,#11621,.F.);
#15203=ORIENTED_EDGE('',*,*,#11620,.F.);
#15204=ORIENTED_EDGE('',*,*,#11617,.T.);
#15205=ORIENTED_EDGE('',*,*,#11622,.T.);
#15206=ORIENTED_EDGE('',*,*,#11623,.F.);
#15207=ORIENTED_EDGE('',*,*,#11622,.F.);
#15208=ORIENTED_EDGE('',*,*,#11616,.F.);
#15209=ORIENTED_EDGE('',*,*,#11624,.F.);
#15210=ORIENTED_EDGE('',*,*,#11625,.T.);
#15211=ORIENTED_EDGE('',*,*,#11626,.F.);
#15212=ORIENTED_EDGE('',*,*,#11627,.F.);
#15213=ORIENTED_EDGE('',*,*,#11628,.F.);
#15214=ORIENTED_EDGE('',*,*,#11627,.T.);
#15215=ORIENTED_EDGE('',*,*,#11629,.T.);
#15216=ORIENTED_EDGE('',*,*,#11630,.F.);
#15217=ORIENTED_EDGE('',*,*,#11629,.F.);
#15218=ORIENTED_EDGE('',*,*,#11626,.T.);
#15219=ORIENTED_EDGE('',*,*,#11631,.T.);
#15220=ORIENTED_EDGE('',*,*,#11632,.F.);
#15221=ORIENTED_EDGE('',*,*,#11631,.F.);
#15222=ORIENTED_EDGE('',*,*,#11625,.F.);
#15223=ORIENTED_EDGE('',*,*,#11633,.F.);
#15224=ORIENTED_EDGE('',*,*,#11634,.T.);
#15225=ORIENTED_EDGE('',*,*,#11635,.F.);
#15226=ORIENTED_EDGE('',*,*,#11636,.F.);
#15227=ORIENTED_EDGE('',*,*,#11637,.F.);
#15228=ORIENTED_EDGE('',*,*,#11636,.T.);
#15229=ORIENTED_EDGE('',*,*,#11638,.T.);
#15230=ORIENTED_EDGE('',*,*,#11639,.F.);
#15231=ORIENTED_EDGE('',*,*,#11638,.F.);
#15232=ORIENTED_EDGE('',*,*,#11635,.T.);
#15233=ORIENTED_EDGE('',*,*,#11640,.T.);
#15234=ORIENTED_EDGE('',*,*,#11641,.F.);
#15235=ORIENTED_EDGE('',*,*,#11640,.F.);
#15236=ORIENTED_EDGE('',*,*,#11634,.F.);
#15237=ORIENTED_EDGE('',*,*,#11642,.F.);
#15238=ORIENTED_EDGE('',*,*,#11643,.T.);
#15239=ORIENTED_EDGE('',*,*,#11644,.F.);
#15240=ORIENTED_EDGE('',*,*,#11645,.F.);
#15241=ORIENTED_EDGE('',*,*,#11646,.F.);
#15242=ORIENTED_EDGE('',*,*,#11645,.T.);
#15243=ORIENTED_EDGE('',*,*,#11647,.T.);
#15244=ORIENTED_EDGE('',*,*,#11648,.F.);
#15245=ORIENTED_EDGE('',*,*,#11647,.F.);
#15246=ORIENTED_EDGE('',*,*,#11644,.T.);
#15247=ORIENTED_EDGE('',*,*,#11649,.T.);
#15248=ORIENTED_EDGE('',*,*,#11650,.F.);
#15249=ORIENTED_EDGE('',*,*,#11649,.F.);
#15250=ORIENTED_EDGE('',*,*,#11643,.F.);
#15251=ORIENTED_EDGE('',*,*,#11651,.F.);
#15252=ORIENTED_EDGE('',*,*,#11652,.T.);
#15253=ORIENTED_EDGE('',*,*,#11653,.T.);
#15254=ORIENTED_EDGE('',*,*,#11654,.F.);
#15255=ORIENTED_EDGE('',*,*,#11655,.T.);
#15256=ORIENTED_EDGE('',*,*,#11656,.F.);
#15257=ORIENTED_EDGE('',*,*,#11652,.F.);
#15258=ORIENTED_EDGE('',*,*,#11657,.F.);
#15259=ORIENTED_EDGE('',*,*,#11653,.F.);
#15260=ORIENTED_EDGE('',*,*,#11656,.T.);
#15261=ORIENTED_EDGE('',*,*,#11658,.T.);
#15262=ORIENTED_EDGE('',*,*,#11659,.F.);
#15263=ORIENTED_EDGE('',*,*,#11658,.F.);
#15264=ORIENTED_EDGE('',*,*,#11655,.F.);
#15265=ORIENTED_EDGE('',*,*,#11660,.F.);
#15266=ORIENTED_EDGE('',*,*,#11661,.T.);
#15267=ORIENTED_EDGE('',*,*,#11662,.F.);
#15268=ORIENTED_EDGE('',*,*,#11663,.F.);
#15269=ORIENTED_EDGE('',*,*,#11664,.F.);
#15270=ORIENTED_EDGE('',*,*,#11663,.T.);
#15271=ORIENTED_EDGE('',*,*,#11665,.T.);
#15272=ORIENTED_EDGE('',*,*,#11666,.F.);
#15273=ORIENTED_EDGE('',*,*,#11665,.F.);
#15274=ORIENTED_EDGE('',*,*,#11662,.T.);
#15275=ORIENTED_EDGE('',*,*,#11667,.T.);
#15276=ORIENTED_EDGE('',*,*,#11668,.F.);
#15277=ORIENTED_EDGE('',*,*,#11667,.F.);
#15278=ORIENTED_EDGE('',*,*,#11661,.F.);
#15279=ORIENTED_EDGE('',*,*,#11669,.F.);
#15280=ORIENTED_EDGE('',*,*,#11670,.T.);
#15281=ORIENTED_EDGE('',*,*,#11671,.F.);
#15282=ORIENTED_EDGE('',*,*,#11672,.F.);
#15283=ORIENTED_EDGE('',*,*,#11673,.F.);
#15284=ORIENTED_EDGE('',*,*,#11672,.T.);
#15285=ORIENTED_EDGE('',*,*,#11674,.T.);
#15286=ORIENTED_EDGE('',*,*,#11675,.F.);
#15287=ORIENTED_EDGE('',*,*,#11674,.F.);
#15288=ORIENTED_EDGE('',*,*,#11671,.T.);
#15289=ORIENTED_EDGE('',*,*,#11676,.T.);
#15290=ORIENTED_EDGE('',*,*,#11677,.F.);
#15291=ORIENTED_EDGE('',*,*,#11676,.F.);
#15292=ORIENTED_EDGE('',*,*,#11670,.F.);
#15293=ORIENTED_EDGE('',*,*,#11678,.F.);
#15294=ORIENTED_EDGE('',*,*,#11679,.T.);
#15295=ORIENTED_EDGE('',*,*,#11680,.F.);
#15296=ORIENTED_EDGE('',*,*,#11681,.F.);
#15297=ORIENTED_EDGE('',*,*,#11682,.F.);
#15298=ORIENTED_EDGE('',*,*,#11681,.T.);
#15299=ORIENTED_EDGE('',*,*,#11683,.T.);
#15300=ORIENTED_EDGE('',*,*,#11684,.F.);
#15301=ORIENTED_EDGE('',*,*,#11683,.F.);
#15302=ORIENTED_EDGE('',*,*,#11680,.T.);
#15303=ORIENTED_EDGE('',*,*,#11685,.T.);
#15304=ORIENTED_EDGE('',*,*,#11686,.F.);
#15305=ORIENTED_EDGE('',*,*,#11685,.F.);
#15306=ORIENTED_EDGE('',*,*,#11679,.F.);
#15307=ORIENTED_EDGE('',*,*,#11687,.F.);
#15308=ORIENTED_EDGE('',*,*,#11688,.T.);
#15309=ORIENTED_EDGE('',*,*,#11689,.F.);
#15310=ORIENTED_EDGE('',*,*,#11690,.F.);
#15311=ORIENTED_EDGE('',*,*,#11691,.F.);
#15312=ORIENTED_EDGE('',*,*,#11690,.T.);
#15313=ORIENTED_EDGE('',*,*,#11692,.T.);
#15314=ORIENTED_EDGE('',*,*,#11693,.F.);
#15315=ORIENTED_EDGE('',*,*,#11692,.F.);
#15316=ORIENTED_EDGE('',*,*,#11689,.T.);
#15317=ORIENTED_EDGE('',*,*,#11694,.T.);
#15318=ORIENTED_EDGE('',*,*,#11695,.F.);
#15319=ORIENTED_EDGE('',*,*,#11694,.F.);
#15320=ORIENTED_EDGE('',*,*,#11688,.F.);
#15321=ORIENTED_EDGE('',*,*,#11696,.F.);
#15322=ORIENTED_EDGE('',*,*,#11697,.T.);
#15323=ORIENTED_EDGE('',*,*,#11698,.F.);
#15324=ORIENTED_EDGE('',*,*,#11699,.F.);
#15325=ORIENTED_EDGE('',*,*,#11700,.F.);
#15326=ORIENTED_EDGE('',*,*,#11699,.T.);
#15327=ORIENTED_EDGE('',*,*,#11701,.T.);
#15328=ORIENTED_EDGE('',*,*,#11702,.F.);
#15329=ORIENTED_EDGE('',*,*,#11701,.F.);
#15330=ORIENTED_EDGE('',*,*,#11698,.T.);
#15331=ORIENTED_EDGE('',*,*,#11703,.T.);
#15332=ORIENTED_EDGE('',*,*,#11704,.F.);
#15333=ORIENTED_EDGE('',*,*,#11703,.F.);
#15334=ORIENTED_EDGE('',*,*,#11697,.F.);
#15335=ORIENTED_EDGE('',*,*,#11705,.F.);
#15336=ORIENTED_EDGE('',*,*,#11706,.T.);
#15337=ORIENTED_EDGE('',*,*,#11707,.F.);
#15338=ORIENTED_EDGE('',*,*,#11708,.F.);
#15339=ORIENTED_EDGE('',*,*,#11709,.F.);
#15340=ORIENTED_EDGE('',*,*,#11708,.T.);
#15341=ORIENTED_EDGE('',*,*,#11710,.T.);
#15342=ORIENTED_EDGE('',*,*,#11711,.F.);
#15343=ORIENTED_EDGE('',*,*,#11710,.F.);
#15344=ORIENTED_EDGE('',*,*,#11707,.T.);
#15345=ORIENTED_EDGE('',*,*,#11712,.T.);
#15346=ORIENTED_EDGE('',*,*,#11713,.F.);
#15347=ORIENTED_EDGE('',*,*,#11712,.F.);
#15348=ORIENTED_EDGE('',*,*,#11706,.F.);
#15349=ORIENTED_EDGE('',*,*,#11714,.F.);
#15350=ORIENTED_EDGE('',*,*,#11715,.T.);
#15351=ORIENTED_EDGE('',*,*,#11716,.F.);
#15352=ORIENTED_EDGE('',*,*,#11717,.F.);
#15353=ORIENTED_EDGE('',*,*,#11718,.F.);
#15354=ORIENTED_EDGE('',*,*,#11717,.T.);
#15355=ORIENTED_EDGE('',*,*,#11719,.T.);
#15356=ORIENTED_EDGE('',*,*,#11720,.F.);
#15357=ORIENTED_EDGE('',*,*,#11719,.F.);
#15358=ORIENTED_EDGE('',*,*,#11716,.T.);
#15359=ORIENTED_EDGE('',*,*,#11721,.T.);
#15360=ORIENTED_EDGE('',*,*,#11722,.F.);
#15361=ORIENTED_EDGE('',*,*,#11721,.F.);
#15362=ORIENTED_EDGE('',*,*,#11715,.F.);
#15363=ORIENTED_EDGE('',*,*,#11723,.F.);
#15364=ORIENTED_EDGE('',*,*,#11724,.T.);
#15365=ORIENTED_EDGE('',*,*,#11725,.F.);
#15366=ORIENTED_EDGE('',*,*,#11726,.F.);
#15367=ORIENTED_EDGE('',*,*,#11727,.F.);
#15368=ORIENTED_EDGE('',*,*,#11726,.T.);
#15369=ORIENTED_EDGE('',*,*,#11728,.T.);
#15370=ORIENTED_EDGE('',*,*,#11729,.F.);
#15371=ORIENTED_EDGE('',*,*,#11728,.F.);
#15372=ORIENTED_EDGE('',*,*,#11725,.T.);
#15373=ORIENTED_EDGE('',*,*,#11730,.T.);
#15374=ORIENTED_EDGE('',*,*,#11731,.F.);
#15375=ORIENTED_EDGE('',*,*,#11730,.F.);
#15376=ORIENTED_EDGE('',*,*,#11724,.F.);
#15377=ORIENTED_EDGE('',*,*,#11732,.F.);
#15378=ORIENTED_EDGE('',*,*,#11733,.T.);
#15379=ORIENTED_EDGE('',*,*,#11734,.F.);
#15380=ORIENTED_EDGE('',*,*,#11735,.F.);
#15381=ORIENTED_EDGE('',*,*,#11736,.F.);
#15382=ORIENTED_EDGE('',*,*,#11735,.T.);
#15383=ORIENTED_EDGE('',*,*,#11737,.T.);
#15384=ORIENTED_EDGE('',*,*,#11738,.F.);
#15385=ORIENTED_EDGE('',*,*,#11737,.F.);
#15386=ORIENTED_EDGE('',*,*,#11734,.T.);
#15387=ORIENTED_EDGE('',*,*,#11739,.T.);
#15388=ORIENTED_EDGE('',*,*,#11740,.F.);
#15389=ORIENTED_EDGE('',*,*,#11739,.F.);
#15390=ORIENTED_EDGE('',*,*,#11733,.F.);
#15391=ORIENTED_EDGE('',*,*,#11741,.F.);
#15392=ORIENTED_EDGE('',*,*,#11742,.T.);
#15393=ORIENTED_EDGE('',*,*,#11743,.F.);
#15394=ORIENTED_EDGE('',*,*,#11744,.F.);
#15395=ORIENTED_EDGE('',*,*,#11745,.F.);
#15396=ORIENTED_EDGE('',*,*,#11744,.T.);
#15397=ORIENTED_EDGE('',*,*,#11746,.T.);
#15398=ORIENTED_EDGE('',*,*,#11747,.F.);
#15399=ORIENTED_EDGE('',*,*,#11746,.F.);
#15400=ORIENTED_EDGE('',*,*,#11743,.T.);
#15401=ORIENTED_EDGE('',*,*,#11748,.T.);
#15402=ORIENTED_EDGE('',*,*,#11749,.F.);
#15403=ORIENTED_EDGE('',*,*,#11748,.F.);
#15404=ORIENTED_EDGE('',*,*,#11742,.F.);
#15405=ORIENTED_EDGE('',*,*,#11750,.F.);
#15406=ORIENTED_EDGE('',*,*,#11751,.T.);
#15407=ORIENTED_EDGE('',*,*,#11752,.F.);
#15408=ORIENTED_EDGE('',*,*,#11753,.F.);
#15409=ORIENTED_EDGE('',*,*,#11754,.F.);
#15410=ORIENTED_EDGE('',*,*,#11753,.T.);
#15411=ORIENTED_EDGE('',*,*,#11755,.T.);
#15412=ORIENTED_EDGE('',*,*,#11756,.F.);
#15413=ORIENTED_EDGE('',*,*,#11755,.F.);
#15414=ORIENTED_EDGE('',*,*,#11752,.T.);
#15415=ORIENTED_EDGE('',*,*,#11757,.T.);
#15416=ORIENTED_EDGE('',*,*,#11758,.F.);
#15417=ORIENTED_EDGE('',*,*,#11757,.F.);
#15418=ORIENTED_EDGE('',*,*,#11751,.F.);
#15419=ORIENTED_EDGE('',*,*,#11759,.F.);
#15420=ORIENTED_EDGE('',*,*,#11760,.T.);
#15421=ORIENTED_EDGE('',*,*,#11761,.F.);
#15422=ORIENTED_EDGE('',*,*,#11762,.F.);
#15423=ORIENTED_EDGE('',*,*,#11763,.F.);
#15424=ORIENTED_EDGE('',*,*,#11762,.T.);
#15425=ORIENTED_EDGE('',*,*,#11764,.T.);
#15426=ORIENTED_EDGE('',*,*,#11765,.F.);
#15427=ORIENTED_EDGE('',*,*,#11764,.F.);
#15428=ORIENTED_EDGE('',*,*,#11761,.T.);
#15429=ORIENTED_EDGE('',*,*,#11766,.T.);
#15430=ORIENTED_EDGE('',*,*,#11767,.F.);
#15431=ORIENTED_EDGE('',*,*,#11766,.F.);
#15432=ORIENTED_EDGE('',*,*,#11760,.F.);
#15433=ORIENTED_EDGE('',*,*,#11768,.F.);
#15434=ORIENTED_EDGE('',*,*,#11769,.T.);
#15435=ORIENTED_EDGE('',*,*,#11770,.F.);
#15436=ORIENTED_EDGE('',*,*,#11771,.F.);
#15437=ORIENTED_EDGE('',*,*,#11772,.F.);
#15438=ORIENTED_EDGE('',*,*,#11771,.T.);
#15439=ORIENTED_EDGE('',*,*,#11773,.T.);
#15440=ORIENTED_EDGE('',*,*,#11774,.F.);
#15441=ORIENTED_EDGE('',*,*,#11773,.F.);
#15442=ORIENTED_EDGE('',*,*,#11770,.T.);
#15443=ORIENTED_EDGE('',*,*,#11775,.T.);
#15444=ORIENTED_EDGE('',*,*,#11776,.F.);
#15445=ORIENTED_EDGE('',*,*,#11775,.F.);
#15446=ORIENTED_EDGE('',*,*,#11769,.F.);
#15447=ORIENTED_EDGE('',*,*,#11777,.F.);
#15448=ORIENTED_EDGE('',*,*,#11778,.T.);
#15449=ORIENTED_EDGE('',*,*,#11779,.F.);
#15450=ORIENTED_EDGE('',*,*,#11780,.F.);
#15451=ORIENTED_EDGE('',*,*,#11781,.F.);
#15452=ORIENTED_EDGE('',*,*,#11780,.T.);
#15453=ORIENTED_EDGE('',*,*,#11782,.T.);
#15454=ORIENTED_EDGE('',*,*,#11783,.F.);
#15455=ORIENTED_EDGE('',*,*,#11782,.F.);
#15456=ORIENTED_EDGE('',*,*,#11779,.T.);
#15457=ORIENTED_EDGE('',*,*,#11784,.T.);
#15458=ORIENTED_EDGE('',*,*,#11785,.F.);
#15459=ORIENTED_EDGE('',*,*,#11784,.F.);
#15460=ORIENTED_EDGE('',*,*,#11778,.F.);
#15461=ORIENTED_EDGE('',*,*,#11786,.F.);
#15462=ORIENTED_EDGE('',*,*,#11787,.T.);
#15463=ORIENTED_EDGE('',*,*,#11788,.F.);
#15464=ORIENTED_EDGE('',*,*,#11789,.F.);
#15465=ORIENTED_EDGE('',*,*,#11790,.F.);
#15466=ORIENTED_EDGE('',*,*,#11789,.T.);
#15467=ORIENTED_EDGE('',*,*,#11791,.T.);
#15468=ORIENTED_EDGE('',*,*,#11792,.F.);
#15469=ORIENTED_EDGE('',*,*,#11793,.F.);
#15470=ORIENTED_EDGE('',*,*,#11791,.F.);
#15471=ORIENTED_EDGE('',*,*,#11788,.T.);
#15472=ORIENTED_EDGE('',*,*,#11794,.T.);
#15473=ORIENTED_EDGE('',*,*,#11795,.F.);
#15474=ORIENTED_EDGE('',*,*,#11794,.F.);
#15475=ORIENTED_EDGE('',*,*,#11787,.F.);
#15476=ORIENTED_EDGE('',*,*,#11796,.F.);
#15477=ORIENTED_EDGE('',*,*,#11797,.F.);
#15478=ORIENTED_EDGE('',*,*,#11798,.T.);
#15479=ORIENTED_EDGE('',*,*,#11799,.F.);
#15480=ORIENTED_EDGE('',*,*,#11800,.F.);
#15481=ORIENTED_EDGE('',*,*,#11801,.F.);
#15482=ORIENTED_EDGE('',*,*,#11800,.T.);
#15483=ORIENTED_EDGE('',*,*,#11802,.T.);
#15484=ORIENTED_EDGE('',*,*,#11803,.F.);
#15485=ORIENTED_EDGE('',*,*,#11802,.F.);
#15486=ORIENTED_EDGE('',*,*,#11799,.T.);
#15487=ORIENTED_EDGE('',*,*,#11804,.T.);
#15488=ORIENTED_EDGE('',*,*,#11805,.F.);
#15489=ORIENTED_EDGE('',*,*,#11804,.F.);
#15490=ORIENTED_EDGE('',*,*,#11798,.F.);
#15491=ORIENTED_EDGE('',*,*,#11806,.F.);
#15492=ORIENTED_EDGE('',*,*,#11807,.T.);
#15493=ORIENTED_EDGE('',*,*,#11808,.F.);
#15494=ORIENTED_EDGE('',*,*,#11809,.F.);
#15495=ORIENTED_EDGE('',*,*,#11810,.F.);
#15496=ORIENTED_EDGE('',*,*,#11809,.T.);
#15497=ORIENTED_EDGE('',*,*,#11811,.T.);
#15498=ORIENTED_EDGE('',*,*,#11812,.F.);
#15499=ORIENTED_EDGE('',*,*,#11811,.F.);
#15500=ORIENTED_EDGE('',*,*,#11808,.T.);
#15501=ORIENTED_EDGE('',*,*,#11813,.T.);
#15502=ORIENTED_EDGE('',*,*,#11814,.F.);
#15503=ORIENTED_EDGE('',*,*,#11813,.F.);
#15504=ORIENTED_EDGE('',*,*,#11807,.F.);
#15505=ORIENTED_EDGE('',*,*,#11815,.F.);
#15506=ORIENTED_EDGE('',*,*,#11816,.T.);
#15507=ORIENTED_EDGE('',*,*,#11817,.F.);
#15508=ORIENTED_EDGE('',*,*,#11818,.F.);
#15509=ORIENTED_EDGE('',*,*,#11819,.F.);
#15510=ORIENTED_EDGE('',*,*,#11818,.T.);
#15511=ORIENTED_EDGE('',*,*,#11820,.T.);
#15512=ORIENTED_EDGE('',*,*,#11821,.F.);
#15513=ORIENTED_EDGE('',*,*,#11820,.F.);
#15514=ORIENTED_EDGE('',*,*,#11817,.T.);
#15515=ORIENTED_EDGE('',*,*,#11822,.T.);
#15516=ORIENTED_EDGE('',*,*,#11823,.F.);
#15517=ORIENTED_EDGE('',*,*,#11822,.F.);
#15518=ORIENTED_EDGE('',*,*,#11816,.F.);
#15519=ORIENTED_EDGE('',*,*,#11824,.F.);
#15520=ORIENTED_EDGE('',*,*,#11825,.T.);
#15521=ORIENTED_EDGE('',*,*,#11826,.F.);
#15522=ORIENTED_EDGE('',*,*,#11827,.F.);
#15523=ORIENTED_EDGE('',*,*,#11828,.F.);
#15524=ORIENTED_EDGE('',*,*,#11827,.T.);
#15525=ORIENTED_EDGE('',*,*,#11829,.T.);
#15526=ORIENTED_EDGE('',*,*,#11830,.F.);
#15527=ORIENTED_EDGE('',*,*,#11829,.F.);
#15528=ORIENTED_EDGE('',*,*,#11826,.T.);
#15529=ORIENTED_EDGE('',*,*,#11831,.T.);
#15530=ORIENTED_EDGE('',*,*,#11832,.F.);
#15531=ORIENTED_EDGE('',*,*,#11831,.F.);
#15532=ORIENTED_EDGE('',*,*,#11825,.F.);
#15533=ORIENTED_EDGE('',*,*,#11833,.F.);
#15534=ORIENTED_EDGE('',*,*,#11834,.T.);
#15535=ORIENTED_EDGE('',*,*,#11835,.F.);
#15536=ORIENTED_EDGE('',*,*,#11836,.F.);
#15537=ORIENTED_EDGE('',*,*,#11837,.F.);
#15538=ORIENTED_EDGE('',*,*,#11836,.T.);
#15539=ORIENTED_EDGE('',*,*,#11838,.T.);
#15540=ORIENTED_EDGE('',*,*,#11839,.F.);
#15541=ORIENTED_EDGE('',*,*,#11838,.F.);
#15542=ORIENTED_EDGE('',*,*,#11835,.T.);
#15543=ORIENTED_EDGE('',*,*,#11840,.T.);
#15544=ORIENTED_EDGE('',*,*,#11841,.F.);
#15545=ORIENTED_EDGE('',*,*,#11840,.F.);
#15546=ORIENTED_EDGE('',*,*,#11834,.F.);
#15547=ORIENTED_EDGE('',*,*,#11842,.F.);
#15548=ORIENTED_EDGE('',*,*,#11843,.T.);
#15549=ORIENTED_EDGE('',*,*,#11844,.F.);
#15550=ORIENTED_EDGE('',*,*,#11845,.F.);
#15551=ORIENTED_EDGE('',*,*,#11846,.F.);
#15552=ORIENTED_EDGE('',*,*,#11845,.T.);
#15553=ORIENTED_EDGE('',*,*,#11847,.T.);
#15554=ORIENTED_EDGE('',*,*,#11848,.F.);
#15555=ORIENTED_EDGE('',*,*,#11847,.F.);
#15556=ORIENTED_EDGE('',*,*,#11844,.T.);
#15557=ORIENTED_EDGE('',*,*,#11849,.T.);
#15558=ORIENTED_EDGE('',*,*,#11850,.F.);
#15559=ORIENTED_EDGE('',*,*,#11849,.F.);
#15560=ORIENTED_EDGE('',*,*,#11843,.F.);
#15561=ORIENTED_EDGE('',*,*,#11851,.F.);
#15562=ORIENTED_EDGE('',*,*,#11852,.T.);
#15563=ORIENTED_EDGE('',*,*,#11853,.F.);
#15564=ORIENTED_EDGE('',*,*,#11854,.F.);
#15565=ORIENTED_EDGE('',*,*,#11855,.F.);
#15566=ORIENTED_EDGE('',*,*,#11854,.T.);
#15567=ORIENTED_EDGE('',*,*,#11856,.T.);
#15568=ORIENTED_EDGE('',*,*,#11857,.F.);
#15569=ORIENTED_EDGE('',*,*,#11856,.F.);
#15570=ORIENTED_EDGE('',*,*,#11853,.T.);
#15571=ORIENTED_EDGE('',*,*,#11858,.T.);
#15572=ORIENTED_EDGE('',*,*,#11859,.F.);
#15573=ORIENTED_EDGE('',*,*,#11858,.F.);
#15574=ORIENTED_EDGE('',*,*,#11852,.F.);
#15575=ORIENTED_EDGE('',*,*,#11860,.F.);
#15576=ORIENTED_EDGE('',*,*,#11861,.T.);
#15577=ORIENTED_EDGE('',*,*,#11862,.F.);
#15578=ORIENTED_EDGE('',*,*,#11863,.F.);
#15579=ORIENTED_EDGE('',*,*,#11864,.F.);
#15580=ORIENTED_EDGE('',*,*,#11865,.F.);
#15581=ORIENTED_EDGE('',*,*,#11866,.F.);
#15582=ORIENTED_EDGE('',*,*,#11867,.F.);
#15583=ORIENTED_EDGE('',*,*,#11868,.F.);
#15584=ORIENTED_EDGE('',*,*,#11861,.F.);
#15585=ORIENTED_EDGE('',*,*,#11866,.T.);
#15586=ORIENTED_EDGE('',*,*,#11869,.T.);
#15587=ORIENTED_EDGE('',*,*,#11870,.T.);
#15588=ORIENTED_EDGE('',*,*,#11871,.F.);
#15589=ORIENTED_EDGE('',*,*,#11865,.T.);
#15590=ORIENTED_EDGE('',*,*,#11872,.T.);
#15591=ORIENTED_EDGE('',*,*,#11873,.T.);
#15592=ORIENTED_EDGE('',*,*,#11869,.F.);
#15593=ORIENTED_EDGE('',*,*,#11864,.T.);
#15594=ORIENTED_EDGE('',*,*,#11874,.T.);
#15595=ORIENTED_EDGE('',*,*,#11875,.T.);
#15596=ORIENTED_EDGE('',*,*,#11872,.F.);
#15597=ORIENTED_EDGE('',*,*,#11870,.F.);
#15598=ORIENTED_EDGE('',*,*,#11873,.F.);
#15599=ORIENTED_EDGE('',*,*,#11875,.F.);
#15600=ORIENTED_EDGE('',*,*,#11876,.F.);
#15601=ORIENTED_EDGE('',*,*,#11877,.F.);
#15602=ORIENTED_EDGE('',*,*,#11878,.T.);
#15603=ORIENTED_EDGE('',*,*,#11879,.F.);
#15604=ORIENTED_EDGE('',*,*,#11878,.F.);
#15605=ORIENTED_EDGE('',*,*,#11880,.F.);
#15606=ORIENTED_EDGE('',*,*,#11881,.F.);
#15607=ORIENTED_EDGE('',*,*,#11863,.T.);
#15608=ORIENTED_EDGE('',*,*,#11882,.T.);
#15609=ORIENTED_EDGE('',*,*,#11876,.T.);
#15610=ORIENTED_EDGE('',*,*,#11874,.F.);
#15611=ORIENTED_EDGE('',*,*,#11879,.T.);
#15612=ORIENTED_EDGE('',*,*,#11883,.F.);
#15613=ORIENTED_EDGE('',*,*,#11860,.T.);
#15614=ORIENTED_EDGE('',*,*,#11884,.F.);
#15615=ORIENTED_EDGE('',*,*,#11867,.T.);
#15616=ORIENTED_EDGE('',*,*,#11871,.T.);
#15617=ORIENTED_EDGE('',*,*,#11881,.T.);
#15618=ORIENTED_EDGE('',*,*,#11885,.F.);
#15619=ORIENTED_EDGE('',*,*,#11862,.T.);
#15620=ORIENTED_EDGE('',*,*,#11868,.T.);
#15621=ORIENTED_EDGE('',*,*,#11885,.T.);
#15622=ORIENTED_EDGE('',*,*,#11880,.T.);
#15623=ORIENTED_EDGE('',*,*,#11877,.T.);
#15624=ORIENTED_EDGE('',*,*,#11882,.F.);
#15625=ORIENTED_EDGE('',*,*,#11886,.F.);
#15626=ORIENTED_EDGE('',*,*,#11887,.T.);
#15627=ORIENTED_EDGE('',*,*,#11888,.T.);
#15628=ORIENTED_EDGE('',*,*,#11887,.F.);
#15629=ORIENTED_EDGE('',*,*,#11888,.F.);
#15630=ORIENTED_EDGE('',*,*,#11889,.T.);
#15631=ORIENTED_EDGE('',*,*,#11889,.F.);
#15632=ORIENTED_EDGE('',*,*,#11890,.F.);
#15633=ORIENTED_EDGE('',*,*,#11886,.T.);
#15634=ORIENTED_EDGE('',*,*,#11559,.F.);
#15635=ORIENTED_EDGE('',*,*,#11560,.F.);
#15636=ORIENTED_EDGE('',*,*,#11891,.T.);
#15637=ORIENTED_EDGE('',*,*,#11890,.T.);
#15638=ORIENTED_EDGE('',*,*,#11891,.F.);
#15639=ORIENTED_EDGE('',*,*,#11549,.T.);
#15640=ORIENTED_EDGE('',*,*,#11553,.T.);
#15641=ORIENTED_EDGE('',*,*,#11556,.T.);
#15642=ORIENTED_EDGE('',*,*,#11525,.T.);
#15643=ORIENTED_EDGE('',*,*,#11565,.T.);
#15644=ORIENTED_EDGE('',*,*,#11567,.T.);
#15645=ORIENTED_EDGE('',*,*,#11569,.T.);
#15646=ORIENTED_EDGE('',*,*,#11892,.F.);
#15647=ORIENTED_EDGE('',*,*,#11884,.T.);
#15648=ORIENTED_EDGE('',*,*,#11893,.T.);
#15649=ORIENTED_EDGE('',*,*,#11892,.T.);
#15650=ORIENTED_EDGE('',*,*,#11893,.F.);
#15651=ORIENTED_EDGE('',*,*,#11588,.T.);
#15652=ORIENTED_EDGE('',*,*,#11894,.F.);
#15653=ORIENTED_EDGE('',*,*,#11848,.T.);
#15654=ORIENTED_EDGE('',*,*,#11850,.T.);
#15655=ORIENTED_EDGE('',*,*,#11842,.T.);
#15656=ORIENTED_EDGE('',*,*,#11895,.F.);
#15657=ORIENTED_EDGE('',*,*,#11603,.T.);
#15658=ORIENTED_EDGE('',*,*,#11605,.T.);
#15659=ORIENTED_EDGE('',*,*,#11597,.T.);
#15660=ORIENTED_EDGE('',*,*,#11896,.F.);
#15661=ORIENTED_EDGE('',*,*,#11839,.T.);
#15662=ORIENTED_EDGE('',*,*,#11841,.T.);
#15663=ORIENTED_EDGE('',*,*,#11833,.T.);
#15664=ORIENTED_EDGE('',*,*,#11897,.F.);
#15665=ORIENTED_EDGE('',*,*,#11612,.T.);
#15666=ORIENTED_EDGE('',*,*,#11614,.T.);
#15667=ORIENTED_EDGE('',*,*,#11606,.T.);
#15668=ORIENTED_EDGE('',*,*,#11898,.F.);
#15669=ORIENTED_EDGE('',*,*,#11830,.T.);
#15670=ORIENTED_EDGE('',*,*,#11832,.T.);
#15671=ORIENTED_EDGE('',*,*,#11824,.T.);
#15672=ORIENTED_EDGE('',*,*,#11899,.F.);
#15673=ORIENTED_EDGE('',*,*,#11621,.T.);
#15674=ORIENTED_EDGE('',*,*,#11623,.T.);
#15675=ORIENTED_EDGE('',*,*,#11615,.T.);
#15676=ORIENTED_EDGE('',*,*,#11900,.F.);
#15677=ORIENTED_EDGE('',*,*,#11821,.T.);
#15678=ORIENTED_EDGE('',*,*,#11823,.T.);
#15679=ORIENTED_EDGE('',*,*,#11815,.T.);
#15680=ORIENTED_EDGE('',*,*,#11901,.F.);
#15681=ORIENTED_EDGE('',*,*,#11630,.T.);
#15682=ORIENTED_EDGE('',*,*,#11632,.T.);
#15683=ORIENTED_EDGE('',*,*,#11624,.T.);
#15684=ORIENTED_EDGE('',*,*,#11902,.F.);
#15685=ORIENTED_EDGE('',*,*,#11812,.T.);
#15686=ORIENTED_EDGE('',*,*,#11814,.T.);
#15687=ORIENTED_EDGE('',*,*,#11806,.T.);
#15688=ORIENTED_EDGE('',*,*,#11903,.F.);
#15689=ORIENTED_EDGE('',*,*,#11639,.T.);
#15690=ORIENTED_EDGE('',*,*,#11641,.T.);
#15691=ORIENTED_EDGE('',*,*,#11633,.T.);
#15692=ORIENTED_EDGE('',*,*,#11904,.F.);
#15693=ORIENTED_EDGE('',*,*,#11803,.T.);
#15694=ORIENTED_EDGE('',*,*,#11805,.T.);
#15695=ORIENTED_EDGE('',*,*,#11797,.T.);
#15696=ORIENTED_EDGE('',*,*,#11905,.F.);
#15697=ORIENTED_EDGE('',*,*,#11648,.T.);
#15698=ORIENTED_EDGE('',*,*,#11650,.T.);
#15699=ORIENTED_EDGE('',*,*,#11642,.T.);
#15700=ORIENTED_EDGE('',*,*,#11906,.F.);
#15701=ORIENTED_EDGE('',*,*,#11793,.T.);
#15702=ORIENTED_EDGE('',*,*,#11795,.T.);
#15703=ORIENTED_EDGE('',*,*,#11907,.T.);
#15704=ORIENTED_EDGE('',*,*,#11883,.T.);
#15705=ORIENTED_EDGE('',*,*,#11907,.F.);
#15706=ORIENTED_EDGE('',*,*,#11796,.T.);
#15707=ORIENTED_EDGE('',*,*,#11786,.T.);
#15708=ORIENTED_EDGE('',*,*,#11908,.F.);
#15709=ORIENTED_EDGE('',*,*,#11783,.T.);
#15710=ORIENTED_EDGE('',*,*,#11785,.T.);
#15711=ORIENTED_EDGE('',*,*,#11777,.T.);
#15712=ORIENTED_EDGE('',*,*,#11909,.F.);
#15713=ORIENTED_EDGE('',*,*,#11666,.T.);
#15714=ORIENTED_EDGE('',*,*,#11668,.T.);
#15715=ORIENTED_EDGE('',*,*,#11660,.T.);
#15716=ORIENTED_EDGE('',*,*,#11910,.F.);
#15717=ORIENTED_EDGE('',*,*,#11774,.T.);
#15718=ORIENTED_EDGE('',*,*,#11776,.T.);
#15719=ORIENTED_EDGE('',*,*,#11768,.T.);
#15720=ORIENTED_EDGE('',*,*,#11911,.F.);
#15721=ORIENTED_EDGE('',*,*,#11675,.T.);
#15722=ORIENTED_EDGE('',*,*,#11677,.T.);
#15723=ORIENTED_EDGE('',*,*,#11669,.T.);
#15724=ORIENTED_EDGE('',*,*,#11912,.F.);
#15725=ORIENTED_EDGE('',*,*,#11765,.T.);
#15726=ORIENTED_EDGE('',*,*,#11767,.T.);
#15727=ORIENTED_EDGE('',*,*,#11759,.T.);
#15728=ORIENTED_EDGE('',*,*,#11913,.F.);
#15729=ORIENTED_EDGE('',*,*,#11684,.T.);
#15730=ORIENTED_EDGE('',*,*,#11686,.T.);
#15731=ORIENTED_EDGE('',*,*,#11678,.T.);
#15732=ORIENTED_EDGE('',*,*,#11914,.F.);
#15733=ORIENTED_EDGE('',*,*,#11756,.T.);
#15734=ORIENTED_EDGE('',*,*,#11758,.T.);
#15735=ORIENTED_EDGE('',*,*,#11750,.T.);
#15736=ORIENTED_EDGE('',*,*,#11915,.F.);
#15737=ORIENTED_EDGE('',*,*,#11693,.T.);
#15738=ORIENTED_EDGE('',*,*,#11695,.T.);
#15739=ORIENTED_EDGE('',*,*,#11687,.T.);
#15740=ORIENTED_EDGE('',*,*,#11916,.F.);
#15741=ORIENTED_EDGE('',*,*,#11747,.T.);
#15742=ORIENTED_EDGE('',*,*,#11749,.T.);
#15743=ORIENTED_EDGE('',*,*,#11741,.T.);
#15744=ORIENTED_EDGE('',*,*,#11917,.F.);
#15745=ORIENTED_EDGE('',*,*,#11702,.T.);
#15746=ORIENTED_EDGE('',*,*,#11704,.T.);
#15747=ORIENTED_EDGE('',*,*,#11696,.T.);
#15748=ORIENTED_EDGE('',*,*,#11918,.F.);
#15749=ORIENTED_EDGE('',*,*,#11738,.T.);
#15750=ORIENTED_EDGE('',*,*,#11740,.T.);
#15751=ORIENTED_EDGE('',*,*,#11732,.T.);
#15752=ORIENTED_EDGE('',*,*,#11919,.F.);
#15753=ORIENTED_EDGE('',*,*,#11711,.T.);
#15754=ORIENTED_EDGE('',*,*,#11713,.T.);
#15755=ORIENTED_EDGE('',*,*,#11705,.T.);
#15756=ORIENTED_EDGE('',*,*,#11920,.F.);
#15757=ORIENTED_EDGE('',*,*,#11729,.T.);
#15758=ORIENTED_EDGE('',*,*,#11731,.T.);
#15759=ORIENTED_EDGE('',*,*,#11723,.T.);
#15760=ORIENTED_EDGE('',*,*,#11921,.F.);
#15761=ORIENTED_EDGE('',*,*,#11720,.T.);
#15762=ORIENTED_EDGE('',*,*,#11722,.T.);
#15763=ORIENTED_EDGE('',*,*,#11714,.T.);
#15764=ORIENTED_EDGE('',*,*,#11922,.F.);
#15765=ORIENTED_EDGE('',*,*,#11657,.T.);
#15766=ORIENTED_EDGE('',*,*,#11659,.T.);
#15767=ORIENTED_EDGE('',*,*,#11654,.T.);
#15768=ORIENTED_EDGE('',*,*,#11923,.F.);
#15769=ORIENTED_EDGE('',*,*,#11857,.T.);
#15770=ORIENTED_EDGE('',*,*,#11859,.T.);
#15771=ORIENTED_EDGE('',*,*,#11851,.T.);
#15772=ORIENTED_EDGE('',*,*,#11924,.F.);
#15773=ORIENTED_EDGE('',*,*,#11594,.T.);
#15774=ORIENTED_EDGE('',*,*,#11596,.T.);
#15775=ORIENTED_EDGE('',*,*,#11925,.F.);
#15776=ORIENTED_EDGE('',*,*,#11926,.T.);
#15777=ORIENTED_EDGE('',*,*,#11792,.T.);
#15778=ORIENTED_EDGE('',*,*,#11906,.T.);
#15779=ORIENTED_EDGE('',*,*,#11646,.T.);
#15780=ORIENTED_EDGE('',*,*,#11905,.T.);
#15781=ORIENTED_EDGE('',*,*,#11801,.T.);
#15782=ORIENTED_EDGE('',*,*,#11904,.T.);
#15783=ORIENTED_EDGE('',*,*,#11637,.T.);
#15784=ORIENTED_EDGE('',*,*,#11903,.T.);
#15785=ORIENTED_EDGE('',*,*,#11810,.T.);
#15786=ORIENTED_EDGE('',*,*,#11902,.T.);
#15787=ORIENTED_EDGE('',*,*,#11628,.T.);
#15788=ORIENTED_EDGE('',*,*,#11901,.T.);
#15789=ORIENTED_EDGE('',*,*,#11819,.T.);
#15790=ORIENTED_EDGE('',*,*,#11900,.T.);
#15791=ORIENTED_EDGE('',*,*,#11619,.T.);
#15792=ORIENTED_EDGE('',*,*,#11899,.T.);
#15793=ORIENTED_EDGE('',*,*,#11828,.T.);
#15794=ORIENTED_EDGE('',*,*,#11898,.T.);
#15795=ORIENTED_EDGE('',*,*,#11610,.T.);
#15796=ORIENTED_EDGE('',*,*,#11897,.T.);
#15797=ORIENTED_EDGE('',*,*,#11837,.T.);
#15798=ORIENTED_EDGE('',*,*,#11896,.T.);
#15799=ORIENTED_EDGE('',*,*,#11601,.T.);
#15800=ORIENTED_EDGE('',*,*,#11895,.T.);
#15801=ORIENTED_EDGE('',*,*,#11846,.T.);
#15802=ORIENTED_EDGE('',*,*,#11894,.T.);
#15803=ORIENTED_EDGE('',*,*,#11592,.T.);
#15804=ORIENTED_EDGE('',*,*,#11924,.T.);
#15805=ORIENTED_EDGE('',*,*,#11855,.T.);
#15806=ORIENTED_EDGE('',*,*,#11923,.T.);
#15807=ORIENTED_EDGE('',*,*,#11651,.T.);
#15808=ORIENTED_EDGE('',*,*,#11922,.T.);
#15809=ORIENTED_EDGE('',*,*,#11718,.T.);
#15810=ORIENTED_EDGE('',*,*,#11921,.T.);
#15811=ORIENTED_EDGE('',*,*,#11727,.T.);
#15812=ORIENTED_EDGE('',*,*,#11920,.T.);
#15813=ORIENTED_EDGE('',*,*,#11709,.T.);
#15814=ORIENTED_EDGE('',*,*,#11919,.T.);
#15815=ORIENTED_EDGE('',*,*,#11736,.T.);
#15816=ORIENTED_EDGE('',*,*,#11918,.T.);
#15817=ORIENTED_EDGE('',*,*,#11700,.T.);
#15818=ORIENTED_EDGE('',*,*,#11917,.T.);
#15819=ORIENTED_EDGE('',*,*,#11745,.T.);
#15820=ORIENTED_EDGE('',*,*,#11916,.T.);
#15821=ORIENTED_EDGE('',*,*,#11691,.T.);
#15822=ORIENTED_EDGE('',*,*,#11915,.T.);
#15823=ORIENTED_EDGE('',*,*,#11754,.T.);
#15824=ORIENTED_EDGE('',*,*,#11914,.T.);
#15825=ORIENTED_EDGE('',*,*,#11682,.T.);
#15826=ORIENTED_EDGE('',*,*,#11913,.T.);
#15827=ORIENTED_EDGE('',*,*,#11763,.T.);
#15828=ORIENTED_EDGE('',*,*,#11912,.T.);
#15829=ORIENTED_EDGE('',*,*,#11673,.T.);
#15830=ORIENTED_EDGE('',*,*,#11911,.T.);
#15831=ORIENTED_EDGE('',*,*,#11772,.T.);
#15832=ORIENTED_EDGE('',*,*,#11910,.T.);
#15833=ORIENTED_EDGE('',*,*,#11664,.T.);
#15834=ORIENTED_EDGE('',*,*,#11909,.T.);
#15835=ORIENTED_EDGE('',*,*,#11781,.T.);
#15836=ORIENTED_EDGE('',*,*,#11908,.T.);
#15837=ORIENTED_EDGE('',*,*,#11790,.T.);
#15838=ORIENTED_EDGE('',*,*,#11926,.F.);
#15839=ORIENTED_EDGE('',*,*,#11925,.T.);
#15840=ORIENTED_EDGE('',*,*,#11570,.T.);
#15841=ORIENTED_EDGE('',*,*,#11586,.T.);
#15842=ORIENTED_EDGE('',*,*,#11583,.T.);
#15843=ORIENTED_EDGE('',*,*,#11580,.T.);
#15844=ORIENTED_EDGE('',*,*,#11577,.T.);
#15845=ORIENTED_EDGE('',*,*,#11574,.T.);
#21349=CONICAL_SURFACE('',#23433,1.18258529610859,1.0471975511966);
#21350=CONICAL_SURFACE('',#23438,1.18258529610859,1.0471975511966);
#21351=CONICAL_SURFACE('',#23450,0.3,0.982793723247329);
#21352=CONICAL_SURFACE('',#23453,0.7931,0.785398163397448);
#21353=CONICAL_SURFACE('',#23488,0.87,0.785398163397447);
#21589=ADVANCED_FACE('',(#2759),#2434,.T.);
#21590=ADVANCED_FACE('',(#2760),#2435,.T.);
#21591=ADVANCED_FACE('',(#2761),#2436,.T.);
#21592=ADVANCED_FACE('',(#2762),#2437,.T.);
#21593=ADVANCED_FACE('',(#2763),#2438,.T.);
#21594=ADVANCED_FACE('',(#2764),#2439,.T.);
#21595=ADVANCED_FACE('',(#2765),#2440,.T.);
#21596=ADVANCED_FACE('',(#2766),#2441,.T.);
#21597=ADVANCED_FACE('',(#2767),#318,.T.);
#21598=ADVANCED_FACE('',(#2768),#319,.F.);
#21599=ADVANCED_FACE('',(#2769),#320,.F.);
#21600=ADVANCED_FACE('',(#2770),#1836,.T.);
#21601=ADVANCED_FACE('',(#2771),#2442,.T.);
#21602=ADVANCED_FACE('',(#2772),#321,.F.);
#21603=ADVANCED_FACE('',(#2773),#322,.F.);
#21604=ADVANCED_FACE('',(#2774),#323,.T.);
#21605=ADVANCED_FACE('',(#2775),#1837,.F.);
#21606=ADVANCED_FACE('',(#2776),#1838,.F.);
#21607=ADVANCED_FACE('',(#2777),#1839,.F.);
#21608=ADVANCED_FACE('',(#2778),#1840,.F.);
#21609=ADVANCED_FACE('',(#2779),#1841,.F.);
#21610=ADVANCED_FACE('',(#2780),#1842,.F.);
#21611=ADVANCED_FACE('',(#2781),#1843,.F.);
#21612=ADVANCED_FACE('',(#2782),#1844,.F.);
#21613=ADVANCED_FACE('',(#2783),#1845,.F.);
#21614=ADVANCED_FACE('',(#2784),#1846,.F.);
#21615=ADVANCED_FACE('',(#2785),#1847,.F.);
#21616=ADVANCED_FACE('',(#2786),#1848,.F.);
#21617=ADVANCED_FACE('',(#2787),#1849,.F.);
#21618=ADVANCED_FACE('',(#2788),#1850,.F.);
#21619=ADVANCED_FACE('',(#2789),#1851,.F.);
#21620=ADVANCED_FACE('',(#2790),#1852,.F.);
#21621=ADVANCED_FACE('',(#2791),#1853,.F.);
#21622=ADVANCED_FACE('',(#2792),#1854,.F.);
#21623=ADVANCED_FACE('',(#2793),#1855,.F.);
#21624=ADVANCED_FACE('',(#2794),#1856,.F.);
#21625=ADVANCED_FACE('',(#2795),#1857,.F.);
#21626=ADVANCED_FACE('',(#2796),#1858,.F.);
#21627=ADVANCED_FACE('',(#2797),#1859,.F.);
#21628=ADVANCED_FACE('',(#2798),#1860,.F.);
#21629=ADVANCED_FACE('',(#2799),#1861,.F.);
#21630=ADVANCED_FACE('',(#2800),#1862,.F.);
#21631=ADVANCED_FACE('',(#2801),#1863,.F.);
#21632=ADVANCED_FACE('',(#2802),#1864,.F.);
#21633=ADVANCED_FACE('',(#2803),#1865,.F.);
#21634=ADVANCED_FACE('',(#2804),#1866,.F.);
#21635=ADVANCED_FACE('',(#2805),#1867,.F.);
#21636=ADVANCED_FACE('',(#2806),#1868,.F.);
#21637=ADVANCED_FACE('',(#2807),#1869,.F.);
#21638=ADVANCED_FACE('',(#2808),#1870,.F.);
#21639=ADVANCED_FACE('',(#2809),#1871,.F.);
#21640=ADVANCED_FACE('',(#2810),#1872,.F.);
#21641=ADVANCED_FACE('',(#2811),#1873,.F.);
#21642=ADVANCED_FACE('',(#2812),#1874,.F.);
#21643=ADVANCED_FACE('',(#2813),#1875,.F.);
#21644=ADVANCED_FACE('',(#2814),#1876,.F.);
#21645=ADVANCED_FACE('',(#2815),#1877,.F.);
#21646=ADVANCED_FACE('',(#2816),#1878,.F.);
#21647=ADVANCED_FACE('',(#2817),#1879,.F.);
#21648=ADVANCED_FACE('',(#2818),#1880,.F.);
#21649=ADVANCED_FACE('',(#2819),#1881,.F.);
#21650=ADVANCED_FACE('',(#2820),#1882,.F.);
#21651=ADVANCED_FACE('',(#2821),#1883,.F.);
#21652=ADVANCED_FACE('',(#2822),#1884,.F.);
#21653=ADVANCED_FACE('',(#2823),#1885,.F.);
#21654=ADVANCED_FACE('',(#2824),#1886,.F.);
#21655=ADVANCED_FACE('',(#2825),#1887,.F.);
#21656=ADVANCED_FACE('',(#2826),#1888,.F.);
#21657=ADVANCED_FACE('',(#2827),#1889,.F.);
#21658=ADVANCED_FACE('',(#2828),#1890,.F.);
#21659=ADVANCED_FACE('',(#2829),#1891,.F.);
#21660=ADVANCED_FACE('',(#2830),#1892,.F.);
#21661=ADVANCED_FACE('',(#2831),#1893,.F.);
#21662=ADVANCED_FACE('',(#2832),#1894,.F.);
#21663=ADVANCED_FACE('',(#2833),#1895,.F.);
#21664=ADVANCED_FACE('',(#2834),#1896,.F.);
#21665=ADVANCED_FACE('',(#2835),#1897,.F.);
#21666=ADVANCED_FACE('',(#2836),#1898,.F.);
#21667=ADVANCED_FACE('',(#2837),#1899,.F.);
#21668=ADVANCED_FACE('',(#2838),#1900,.F.);
#21669=ADVANCED_FACE('',(#2839),#1901,.F.);
#21670=ADVANCED_FACE('',(#2840),#1902,.F.);
#21671=ADVANCED_FACE('',(#2841),#1903,.F.);
#21672=ADVANCED_FACE('',(#2842),#1904,.F.);
#21673=ADVANCED_FACE('',(#2843),#1905,.F.);
#21674=ADVANCED_FACE('',(#2844),#1906,.F.);
#21675=ADVANCED_FACE('',(#2845),#1907,.F.);
#21676=ADVANCED_FACE('',(#2846),#1908,.F.);
#21677=ADVANCED_FACE('',(#2847),#1909,.F.);
#21678=ADVANCED_FACE('',(#2848),#1910,.F.);
#21679=ADVANCED_FACE('',(#2849),#1911,.F.);
#21680=ADVANCED_FACE('',(#2850),#1912,.F.);
#21681=ADVANCED_FACE('',(#2851),#1913,.F.);
#21682=ADVANCED_FACE('',(#2852),#1914,.F.);
#21683=ADVANCED_FACE('',(#2853),#1915,.F.);
#21684=ADVANCED_FACE('',(#2854),#1916,.F.);
#21685=ADVANCED_FACE('',(#2855),#1917,.F.);
#21686=ADVANCED_FACE('',(#2856),#1918,.F.);
#21687=ADVANCED_FACE('',(#2857),#1919,.F.);
#21688=ADVANCED_FACE('',(#2858),#1920,.F.);
#21689=ADVANCED_FACE('',(#2859),#1921,.F.);
#21690=ADVANCED_FACE('',(#2860),#1922,.F.);
#21691=ADVANCED_FACE('',(#2861),#1923,.F.);
#21692=ADVANCED_FACE('',(#2862),#1924,.F.);
#21693=ADVANCED_FACE('',(#2863),#1925,.F.);
#21694=ADVANCED_FACE('',(#2864),#1926,.F.);
#21695=ADVANCED_FACE('',(#2865),#1927,.F.);
#21696=ADVANCED_FACE('',(#2866),#1928,.F.);
#21697=ADVANCED_FACE('',(#2867),#1929,.F.);
#21698=ADVANCED_FACE('',(#2868),#1930,.F.);
#21699=ADVANCED_FACE('',(#2869),#1931,.F.);
#21700=ADVANCED_FACE('',(#2870),#1932,.F.);
#21701=ADVANCED_FACE('',(#2871),#1933,.F.);
#21702=ADVANCED_FACE('',(#2872),#1934,.F.);
#21703=ADVANCED_FACE('',(#2873),#1935,.F.);
#21704=ADVANCED_FACE('',(#2874),#1936,.F.);
#21705=ADVANCED_FACE('',(#2875),#1937,.F.);
#21706=ADVANCED_FACE('',(#2876),#1938,.F.);
#21707=ADVANCED_FACE('',(#2877),#1939,.F.);
#21708=ADVANCED_FACE('',(#2878),#1940,.F.);
#21709=ADVANCED_FACE('',(#2879),#1941,.F.);
#21710=ADVANCED_FACE('',(#2880),#1942,.F.);
#21711=ADVANCED_FACE('',(#2881),#1943,.F.);
#21712=ADVANCED_FACE('',(#2882),#1944,.F.);
#21713=ADVANCED_FACE('',(#2883),#1945,.F.);
#21714=ADVANCED_FACE('',(#2884),#1946,.F.);
#21715=ADVANCED_FACE('',(#2885),#1947,.F.);
#21716=ADVANCED_FACE('',(#2886),#1948,.F.);
#21717=ADVANCED_FACE('',(#2887),#1949,.F.);
#21718=ADVANCED_FACE('',(#2888),#1950,.F.);
#21719=ADVANCED_FACE('',(#2889),#1951,.F.);
#21720=ADVANCED_FACE('',(#2890),#1952,.F.);
#21721=ADVANCED_FACE('',(#2891),#1953,.F.);
#21722=ADVANCED_FACE('',(#2892),#1954,.F.);
#21723=ADVANCED_FACE('',(#2893),#1955,.F.);
#21724=ADVANCED_FACE('',(#2894),#1956,.F.);
#21725=ADVANCED_FACE('',(#2895),#1957,.F.);
#21726=ADVANCED_FACE('',(#2896),#1958,.F.);
#21727=ADVANCED_FACE('',(#2897),#1959,.F.);
#21728=ADVANCED_FACE('',(#2898),#1960,.F.);
#21729=ADVANCED_FACE('',(#2899),#1961,.F.);
#21730=ADVANCED_FACE('',(#2900),#1962,.F.);
#21731=ADVANCED_FACE('',(#2901),#1963,.F.);
#21732=ADVANCED_FACE('',(#2902),#21349,.T.);
#21733=ADVANCED_FACE('',(#2903),#1964,.T.);
#21734=ADVANCED_FACE('',(#2904),#1965,.T.);
#21735=ADVANCED_FACE('',(#2905),#1966,.T.);
#21736=ADVANCED_FACE('',(#2906),#21350,.T.);
#21737=ADVANCED_FACE('',(#2907),#1967,.T.);
#21738=ADVANCED_FACE('',(#2908,#1629),#1968,.T.);
#21739=ADVANCED_FACE('',(#2909,#1630),#1969,.F.);
#21740=ADVANCED_FACE('',(#2910),#1970,.T.);
#21741=ADVANCED_FACE('',(#2911),#1971,.T.);
#21742=ADVANCED_FACE('',(#2912),#2443,.F.);
#21743=ADVANCED_FACE('',(#2913),#21351,.F.);
#21744=ADVANCED_FACE('',(#2914,#1631),#1972,.T.);
#21745=ADVANCED_FACE('',(#2915),#21352,.T.);
#21746=ADVANCED_FACE('',(#2916,#1632),#1973,.T.);
#21747=ADVANCED_FACE('',(#2917),#2444,.T.);
#21748=ADVANCED_FACE('',(#2918),#2445,.T.);
#21749=ADVANCED_FACE('',(#2919),#21353,.T.);
#21750=ADVANCED_FACE('',(#2920,#1633),#1974,.T.);
#22810=CLOSED_SHELL('',(#21589,#21590,#21591,#21592,#21593,#21594,#21595,
#21596,#21597,#21598,#21599,#21600,#21601,#21602,#21603,#21604,#21605,#21606,
#21607,#21608,#21609,#21610,#21611,#21612,#21613,#21614,#21615,#21616,#21617,
#21618,#21619,#21620,#21621,#21622,#21623,#21624,#21625,#21626,#21627,#21628,
#21629,#21630,#21631,#21632,#21633,#21634,#21635,#21636,#21637,#21638,#21639,
#21640,#21641,#21642,#21643,#21644,#21645,#21646,#21647,#21648,#21649,#21650,
#21651,#21652,#21653,#21654,#21655,#21656,#21657,#21658,#21659,#21660,#21661,
#21662,#21663,#21664,#21665,#21666,#21667,#21668,#21669,#21670,#21671,#21672,
#21673,#21674,#21675,#21676,#21677,#21678,#21679,#21680,#21681,#21682,#21683,
#21684,#21685,#21686,#21687,#21688,#21689,#21690,#21691,#21692,#21693,#21694,
#21695,#21696,#21697,#21698,#21699,#21700,#21701,#21702,#21703,#21704,#21705,
#21706,#21707,#21708,#21709,#21710,#21711,#21712,#21713,#21714,#21715,#21716,
#21717,#21718,#21719,#21720,#21721,#21722,#21723,#21724,#21725,#21726,#21727,
#21728,#21729,#21730,#21731,#21732,#21733,#21734,#21735,#21736,#21737,#21738,
#21739,#21740,#21741,#21742,#21743,#21744,#21745,#21746,#21747,#21748,#21749,
#21750));
#23228=AXIS2_PLACEMENT_3D('',#32296,#25566,#25567);
#23229=AXIS2_PLACEMENT_3D('',#32297,#25568,#25569);
#23230=AXIS2_PLACEMENT_3D('',#32314,#25571,#25572);
#23231=AXIS2_PLACEMENT_3D('',#32325,#25573,#25574);
#23232=AXIS2_PLACEMENT_3D('',#32363,#25576,#25577);
#23233=AXIS2_PLACEMENT_3D('',#32401,#25579,#25580);
#23234=AXIS2_PLACEMENT_3D('',#32438,#25582,#25583);
#23235=AXIS2_PLACEMENT_3D('',#32475,#25585,#25586);
#23236=AXIS2_PLACEMENT_3D('',#32513,#25588,#25589);
#23237=AXIS2_PLACEMENT_3D('',#32551,#25591,#25592);
#23238=AXIS2_PLACEMENT_3D('',#32556,#25594,#25595);
#23239=AXIS2_PLACEMENT_3D('',#34639,#25596,#25597);
#23240=AXIS2_PLACEMENT_3D('',#34641,#25598,#25599);
#23241=AXIS2_PLACEMENT_3D('',#34642,#25600,#25601);
#23242=AXIS2_PLACEMENT_3D('',#34708,#25602,#25603);
#23243=AXIS2_PLACEMENT_3D('',#34709,#25604,#25605);
#23244=AXIS2_PLACEMENT_3D('',#36391,#25606,#25607);
#23245=AXIS2_PLACEMENT_3D('',#36400,#25612,#25613);
#23246=AXIS2_PLACEMENT_3D('',#36406,#25617,#25618);
#23247=AXIS2_PLACEMENT_3D('',#36412,#25622,#25623);
#23248=AXIS2_PLACEMENT_3D('',#36418,#25627,#25628);
#23249=AXIS2_PLACEMENT_3D('',#36424,#25632,#25633);
#23250=AXIS2_PLACEMENT_3D('',#36427,#25636,#25637);
#23251=AXIS2_PLACEMENT_3D('',#36428,#25638,#25639);
#23252=AXIS2_PLACEMENT_3D('',#36437,#25644,#25645);
#23253=AXIS2_PLACEMENT_3D('',#36439,#25646,#25647);
#23254=AXIS2_PLACEMENT_3D('',#36441,#25649,#25650);
#23255=AXIS2_PLACEMENT_3D('',#36445,#25653,#25654);
#23256=AXIS2_PLACEMENT_3D('',#36446,#25655,#25656);
#23257=AXIS2_PLACEMENT_3D('',#36447,#25657,#25658);
#23258=AXIS2_PLACEMENT_3D('',#36456,#25663,#25664);
#23259=AXIS2_PLACEMENT_3D('',#36458,#25665,#25666);
#23260=AXIS2_PLACEMENT_3D('',#36460,#25668,#25669);
#23261=AXIS2_PLACEMENT_3D('',#36464,#25672,#25673);
#23262=AXIS2_PLACEMENT_3D('',#36465,#25674,#25675);
#23263=AXIS2_PLACEMENT_3D('',#36466,#25676,#25677);
#23264=AXIS2_PLACEMENT_3D('',#36475,#25682,#25683);
#23265=AXIS2_PLACEMENT_3D('',#36477,#25684,#25685);
#23266=AXIS2_PLACEMENT_3D('',#36479,#25687,#25688);
#23267=AXIS2_PLACEMENT_3D('',#36483,#25691,#25692);
#23268=AXIS2_PLACEMENT_3D('',#36484,#25693,#25694);
#23269=AXIS2_PLACEMENT_3D('',#36485,#25695,#25696);
#23270=AXIS2_PLACEMENT_3D('',#36494,#25701,#25702);
#23271=AXIS2_PLACEMENT_3D('',#36496,#25703,#25704);
#23272=AXIS2_PLACEMENT_3D('',#36498,#25706,#25707);
#23273=AXIS2_PLACEMENT_3D('',#36502,#25710,#25711);
#23274=AXIS2_PLACEMENT_3D('',#36503,#25712,#25713);
#23275=AXIS2_PLACEMENT_3D('',#36504,#25714,#25715);
#23276=AXIS2_PLACEMENT_3D('',#36513,#25720,#25721);
#23277=AXIS2_PLACEMENT_3D('',#36515,#25722,#25723);
#23278=AXIS2_PLACEMENT_3D('',#36517,#25725,#25726);
#23279=AXIS2_PLACEMENT_3D('',#36521,#25729,#25730);
#23280=AXIS2_PLACEMENT_3D('',#36522,#25731,#25732);
#23281=AXIS2_PLACEMENT_3D('',#36523,#25733,#25734);
#23282=AXIS2_PLACEMENT_3D('',#36532,#25739,#25740);
#23283=AXIS2_PLACEMENT_3D('',#36534,#25741,#25742);
#23284=AXIS2_PLACEMENT_3D('',#36536,#25744,#25745);
#23285=AXIS2_PLACEMENT_3D('',#36540,#25748,#25749);
#23286=AXIS2_PLACEMENT_3D('',#36541,#25750,#25751);
#23287=AXIS2_PLACEMENT_3D('',#36542,#25752,#25753);
#23288=AXIS2_PLACEMENT_3D('',#36551,#25758,#25759);
#23289=AXIS2_PLACEMENT_3D('',#36553,#25760,#25761);
#23290=AXIS2_PLACEMENT_3D('',#36555,#25763,#25764);
#23291=AXIS2_PLACEMENT_3D('',#36559,#25767,#25768);
#23292=AXIS2_PLACEMENT_3D('',#36560,#25769,#25770);
#23293=AXIS2_PLACEMENT_3D('',#36561,#25771,#25772);
#23294=AXIS2_PLACEMENT_3D('',#36564,#25773,#25774);
#23295=AXIS2_PLACEMENT_3D('',#36568,#25777,#25778);
#23296=AXIS2_PLACEMENT_3D('',#36574,#25782,#25783);
#23297=AXIS2_PLACEMENT_3D('',#36578,#25786,#25787);
#23298=AXIS2_PLACEMENT_3D('',#36579,#25788,#25789);
#23299=AXIS2_PLACEMENT_3D('',#36580,#25790,#25791);
#23300=AXIS2_PLACEMENT_3D('',#36589,#25796,#25797);
#23301=AXIS2_PLACEMENT_3D('',#36591,#25798,#25799);
#23302=AXIS2_PLACEMENT_3D('',#36593,#25801,#25802);
#23303=AXIS2_PLACEMENT_3D('',#36597,#25805,#25806);
#23304=AXIS2_PLACEMENT_3D('',#36598,#25807,#25808);
#23305=AXIS2_PLACEMENT_3D('',#36599,#25809,#25810);
#23306=AXIS2_PLACEMENT_3D('',#36608,#25815,#25816);
#23307=AXIS2_PLACEMENT_3D('',#36610,#25817,#25818);
#23308=AXIS2_PLACEMENT_3D('',#36612,#25820,#25821);
#23309=AXIS2_PLACEMENT_3D('',#36616,#25824,#25825);
#23310=AXIS2_PLACEMENT_3D('',#36617,#25826,#25827);
#23311=AXIS2_PLACEMENT_3D('',#36618,#25828,#25829);
#23312=AXIS2_PLACEMENT_3D('',#36627,#25834,#25835);
#23313=AXIS2_PLACEMENT_3D('',#36629,#25836,#25837);
#23314=AXIS2_PLACEMENT_3D('',#36631,#25839,#25840);
#23315=AXIS2_PLACEMENT_3D('',#36635,#25843,#25844);
#23316=AXIS2_PLACEMENT_3D('',#36636,#25845,#25846);
#23317=AXIS2_PLACEMENT_3D('',#36637,#25847,#25848);
#23318=AXIS2_PLACEMENT_3D('',#36646,#25853,#25854);
#23319=AXIS2_PLACEMENT_3D('',#36648,#25855,#25856);
#23320=AXIS2_PLACEMENT_3D('',#36650,#25858,#25859);
#23321=AXIS2_PLACEMENT_3D('',#36654,#25862,#25863);
#23322=AXIS2_PLACEMENT_3D('',#36655,#25864,#25865);
#23323=AXIS2_PLACEMENT_3D('',#36656,#25866,#25867);
#23324=AXIS2_PLACEMENT_3D('',#36665,#25872,#25873);
#23325=AXIS2_PLACEMENT_3D('',#36667,#25874,#25875);
#23326=AXIS2_PLACEMENT_3D('',#36669,#25877,#25878);
#23327=AXIS2_PLACEMENT_3D('',#36673,#25881,#25882);
#23328=AXIS2_PLACEMENT_3D('',#36674,#25883,#25884);
#23329=AXIS2_PLACEMENT_3D('',#36675,#25885,#25886);
#23330=AXIS2_PLACEMENT_3D('',#36684,#25891,#25892);
#23331=AXIS2_PLACEMENT_3D('',#36686,#25893,#25894);
#23332=AXIS2_PLACEMENT_3D('',#36688,#25896,#25897);
#23333=AXIS2_PLACEMENT_3D('',#36692,#25900,#25901);
#23334=AXIS2_PLACEMENT_3D('',#36693,#25902,#25903);
#23335=AXIS2_PLACEMENT_3D('',#36694,#25904,#25905);
#23336=AXIS2_PLACEMENT_3D('',#36703,#25910,#25911);
#23337=AXIS2_PLACEMENT_3D('',#36705,#25912,#25913);
#23338=AXIS2_PLACEMENT_3D('',#36707,#25915,#25916);
#23339=AXIS2_PLACEMENT_3D('',#36711,#25919,#25920);
#23340=AXIS2_PLACEMENT_3D('',#36712,#25921,#25922);
#23341=AXIS2_PLACEMENT_3D('',#36713,#25923,#25924);
#23342=AXIS2_PLACEMENT_3D('',#36722,#25929,#25930);
#23343=AXIS2_PLACEMENT_3D('',#36724,#25931,#25932);
#23344=AXIS2_PLACEMENT_3D('',#36726,#25934,#25935);
#23345=AXIS2_PLACEMENT_3D('',#36730,#25938,#25939);
#23346=AXIS2_PLACEMENT_3D('',#36731,#25940,#25941);
#23347=AXIS2_PLACEMENT_3D('',#36732,#25942,#25943);
#23348=AXIS2_PLACEMENT_3D('',#36741,#25948,#25949);
#23349=AXIS2_PLACEMENT_3D('',#36743,#25950,#25951);
#23350=AXIS2_PLACEMENT_3D('',#36745,#25953,#25954);
#23351=AXIS2_PLACEMENT_3D('',#36749,#25957,#25958);
#23352=AXIS2_PLACEMENT_3D('',#36750,#25959,#25960);
#23353=AXIS2_PLACEMENT_3D('',#36751,#25961,#25962);
#23354=AXIS2_PLACEMENT_3D('',#36760,#25967,#25968);
#23355=AXIS2_PLACEMENT_3D('',#36762,#25969,#25970);
#23356=AXIS2_PLACEMENT_3D('',#36764,#25972,#25973);
#23357=AXIS2_PLACEMENT_3D('',#36768,#25976,#25977);
#23358=AXIS2_PLACEMENT_3D('',#36769,#25978,#25979);
#23359=AXIS2_PLACEMENT_3D('',#36770,#25980,#25981);
#23360=AXIS2_PLACEMENT_3D('',#36779,#25986,#25987);
#23361=AXIS2_PLACEMENT_3D('',#36781,#25988,#25989);
#23362=AXIS2_PLACEMENT_3D('',#36783,#25991,#25992);
#23363=AXIS2_PLACEMENT_3D('',#36787,#25995,#25996);
#23364=AXIS2_PLACEMENT_3D('',#36788,#25997,#25998);
#23365=AXIS2_PLACEMENT_3D('',#36789,#25999,#26000);
#23366=AXIS2_PLACEMENT_3D('',#36798,#26005,#26006);
#23367=AXIS2_PLACEMENT_3D('',#36800,#26007,#26008);
#23368=AXIS2_PLACEMENT_3D('',#36802,#26010,#26011);
#23369=AXIS2_PLACEMENT_3D('',#36806,#26014,#26015);
#23370=AXIS2_PLACEMENT_3D('',#36807,#26016,#26017);
#23371=AXIS2_PLACEMENT_3D('',#36808,#26018,#26019);
#23372=AXIS2_PLACEMENT_3D('',#36817,#26024,#26025);
#23373=AXIS2_PLACEMENT_3D('',#36819,#26026,#26027);
#23374=AXIS2_PLACEMENT_3D('',#36821,#26029,#26030);
#23375=AXIS2_PLACEMENT_3D('',#36825,#26033,#26034);
#23376=AXIS2_PLACEMENT_3D('',#36826,#26035,#26036);
#23377=AXIS2_PLACEMENT_3D('',#36827,#26037,#26038);
#23378=AXIS2_PLACEMENT_3D('',#36836,#26043,#26044);
#23379=AXIS2_PLACEMENT_3D('',#36838,#26045,#26046);
#23380=AXIS2_PLACEMENT_3D('',#36840,#26048,#26049);
#23381=AXIS2_PLACEMENT_3D('',#36844,#26052,#26053);
#23382=AXIS2_PLACEMENT_3D('',#36845,#26054,#26055);
#23383=AXIS2_PLACEMENT_3D('',#36846,#26056,#26057);
#23384=AXIS2_PLACEMENT_3D('',#36855,#26062,#26063);
#23385=AXIS2_PLACEMENT_3D('',#36857,#26064,#26065);
#23386=AXIS2_PLACEMENT_3D('',#36860,#26067,#26068);
#23387=AXIS2_PLACEMENT_3D('',#36861,#26069,#26070);
#23388=AXIS2_PLACEMENT_3D('',#36865,#26073,#26074);
#23389=AXIS2_PLACEMENT_3D('',#36867,#26075,#26076);
#23390=AXIS2_PLACEMENT_3D('',#36868,#26077,#26078);
#23391=AXIS2_PLACEMENT_3D('',#36869,#26079,#26080);
#23392=AXIS2_PLACEMENT_3D('',#36878,#26085,#26086);
#23393=AXIS2_PLACEMENT_3D('',#36880,#26087,#26088);
#23394=AXIS2_PLACEMENT_3D('',#36882,#26090,#26091);
#23395=AXIS2_PLACEMENT_3D('',#36886,#26094,#26095);
#23396=AXIS2_PLACEMENT_3D('',#36887,#26096,#26097);
#23397=AXIS2_PLACEMENT_3D('',#36888,#26098,#26099);
#23398=AXIS2_PLACEMENT_3D('',#36897,#26104,#26105);
#23399=AXIS2_PLACEMENT_3D('',#36899,#26106,#26107);
#23400=AXIS2_PLACEMENT_3D('',#36901,#26109,#26110);
#23401=AXIS2_PLACEMENT_3D('',#36905,#26113,#26114);
#23402=AXIS2_PLACEMENT_3D('',#36906,#26115,#26116);
#23403=AXIS2_PLACEMENT_3D('',#36907,#26117,#26118);
#23404=AXIS2_PLACEMENT_3D('',#36916,#26123,#26124);
#23405=AXIS2_PLACEMENT_3D('',#36918,#26125,#26126);
#23406=AXIS2_PLACEMENT_3D('',#36920,#26128,#26129);
#23407=AXIS2_PLACEMENT_3D('',#36924,#26132,#26133);
#23408=AXIS2_PLACEMENT_3D('',#36925,#26134,#26135);
#23409=AXIS2_PLACEMENT_3D('',#36926,#26136,#26137);
#23410=AXIS2_PLACEMENT_3D('',#36935,#26142,#26143);
#23411=AXIS2_PLACEMENT_3D('',#36937,#26144,#26145);
#23412=AXIS2_PLACEMENT_3D('',#36939,#26147,#26148);
#23413=AXIS2_PLACEMENT_3D('',#36943,#26151,#26152);
#23414=AXIS2_PLACEMENT_3D('',#36944,#26153,#26154);
#23415=AXIS2_PLACEMENT_3D('',#36945,#26155,#26156);
#23416=AXIS2_PLACEMENT_3D('',#36954,#26161,#26162);
#23417=AXIS2_PLACEMENT_3D('',#36956,#26163,#26164);
#23418=AXIS2_PLACEMENT_3D('',#36958,#26166,#26167);
#23419=AXIS2_PLACEMENT_3D('',#36962,#26170,#26171);
#23420=AXIS2_PLACEMENT_3D('',#36963,#26172,#26173);
#23421=AXIS2_PLACEMENT_3D('',#36964,#26174,#26175);
#23422=AXIS2_PLACEMENT_3D('',#36973,#26180,#26181);
#23423=AXIS2_PLACEMENT_3D('',#36975,#26182,#26183);
#23424=AXIS2_PLACEMENT_3D('',#36977,#26185,#26186);
#23425=AXIS2_PLACEMENT_3D('',#36981,#26189,#26190);
#23426=AXIS2_PLACEMENT_3D('',#36982,#26191,#26192);
#23427=AXIS2_PLACEMENT_3D('',#36983,#26193,#26194);
#23428=AXIS2_PLACEMENT_3D('',#36992,#26199,#26200);
#23429=AXIS2_PLACEMENT_3D('',#36994,#26201,#26202);
#23430=AXIS2_PLACEMENT_3D('',#36996,#26204,#26205);
#23431=AXIS2_PLACEMENT_3D('',#37000,#26208,#26209);
#23432=AXIS2_PLACEMENT_3D('',#37001,#26210,#26211);
#23433=AXIS2_PLACEMENT_3D('',#37002,#26212,#26213);
#23434=AXIS2_PLACEMENT_3D('',#37004,#26214,#26215);
#23435=AXIS2_PLACEMENT_3D('',#37034,#26217,#26218);
#23436=AXIS2_PLACEMENT_3D('',#37042,#26221,#26222);
#23437=AXIS2_PLACEMENT_3D('',#37048,#26224,#26225);
#23438=AXIS2_PLACEMENT_3D('',#37054,#26227,#26228);
#23439=AXIS2_PLACEMENT_3D('',#37065,#26230,#26231);
#23440=AXIS2_PLACEMENT_3D('',#37073,#26232,#26233);
#23441=AXIS2_PLACEMENT_3D('',#37075,#26235,#26236);
#23442=AXIS2_PLACEMENT_3D('',#37077,#26237,#26238);
#23443=AXIS2_PLACEMENT_3D('',#37078,#26239,#26240);
#23444=AXIS2_PLACEMENT_3D('',#37080,#26241,#26242);
#23445=AXIS2_PLACEMENT_3D('',#37081,#26243,#26244);
#23446=AXIS2_PLACEMENT_3D('',#37083,#26246,#26247);
#23447=AXIS2_PLACEMENT_3D('',#37084,#26248,#26249);
#23448=AXIS2_PLACEMENT_3D('',#37086,#26250,#26251);
#23449=AXIS2_PLACEMENT_3D('',#37089,#26253,#26254);
#23450=AXIS2_PLACEMENT_3D('',#37090,#26255,#26256);
#23451=AXIS2_PLACEMENT_3D('',#37093,#26258,#26259);
#23452=AXIS2_PLACEMENT_3D('',#37095,#26260,#26261);
#23453=AXIS2_PLACEMENT_3D('',#37096,#26262,#26263);
#23454=AXIS2_PLACEMENT_3D('',#37098,#26265,#26266);
#23455=AXIS2_PLACEMENT_3D('',#37100,#26267,#26268);
#23456=AXIS2_PLACEMENT_3D('',#37101,#26269,#26270);
#23457=AXIS2_PLACEMENT_3D('',#37103,#26272,#26273);
#23458=AXIS2_PLACEMENT_3D('',#37104,#26274,#26275);
#23459=AXIS2_PLACEMENT_3D('',#37105,#26276,#26277);
#23460=AXIS2_PLACEMENT_3D('',#37106,#26278,#26279);
#23461=AXIS2_PLACEMENT_3D('',#37107,#26280,#26281);
#23462=AXIS2_PLACEMENT_3D('',#37108,#26282,#26283);
#23463=AXIS2_PLACEMENT_3D('',#37109,#26284,#26285);
#23464=AXIS2_PLACEMENT_3D('',#37110,#26286,#26287);
#23465=AXIS2_PLACEMENT_3D('',#37111,#26288,#26289);
#23466=AXIS2_PLACEMENT_3D('',#37112,#26290,#26291);
#23467=AXIS2_PLACEMENT_3D('',#37113,#26292,#26293);
#23468=AXIS2_PLACEMENT_3D('',#37114,#26294,#26295);
#23469=AXIS2_PLACEMENT_3D('',#37115,#26296,#26297);
#23470=AXIS2_PLACEMENT_3D('',#37116,#26298,#26299);
#23471=AXIS2_PLACEMENT_3D('',#37118,#26301,#26302);
#23472=AXIS2_PLACEMENT_3D('',#37119,#26303,#26304);
#23473=AXIS2_PLACEMENT_3D('',#37120,#26305,#26306);
#23474=AXIS2_PLACEMENT_3D('',#37121,#26307,#26308);
#23475=AXIS2_PLACEMENT_3D('',#37122,#26309,#26310);
#23476=AXIS2_PLACEMENT_3D('',#37123,#26311,#26312);
#23477=AXIS2_PLACEMENT_3D('',#37124,#26313,#26314);
#23478=AXIS2_PLACEMENT_3D('',#37125,#26315,#26316);
#23479=AXIS2_PLACEMENT_3D('',#37126,#26317,#26318);
#23480=AXIS2_PLACEMENT_3D('',#37127,#26319,#26320);
#23481=AXIS2_PLACEMENT_3D('',#37128,#26321,#26322);
#23482=AXIS2_PLACEMENT_3D('',#37129,#26323,#26324);
#23483=AXIS2_PLACEMENT_3D('',#37130,#26325,#26326);
#23484=AXIS2_PLACEMENT_3D('',#37131,#26327,#26328);
#23485=AXIS2_PLACEMENT_3D('',#37132,#26329,#26330);
#23486=AXIS2_PLACEMENT_3D('',#37133,#26331,#26332);
#23487=AXIS2_PLACEMENT_3D('',#37134,#26333,#26334);
#23488=AXIS2_PLACEMENT_3D('',#37135,#26335,#26336);
#23489=AXIS2_PLACEMENT_3D('',#37137,#26337,#26338);
#23490=AXIS2_PLACEMENT_3D('',#37139,#26340,#26341);
#25566=DIRECTION('axis',(0.,0.,1.));
#25567=DIRECTION('refdir',(1.,0.,0.));
#25568=DIRECTION('center_axis',(0.,0.,1.));
#25569=DIRECTION('ref_axis',(0.160995516601036,-0.986955137599661,0.));
#25570=DIRECTION('',(0.,0.,1.));
#25571=DIRECTION('center_axis',(0.,0.,1.));
#25572=DIRECTION('ref_axis',(1.,2.60858704573983E-14,0.));
#25573=DIRECTION('center_axis',(0.,0.,1.));
#25574=DIRECTION('ref_axis',(1.,2.60858704573983E-14,0.));
#25575=DIRECTION('',(0.,0.,1.));
#25576=DIRECTION('center_axis',(0.,0.,1.));
#25577=DIRECTION('ref_axis',(1.,2.60858704573983E-14,0.));
#25578=DIRECTION('',(0.,0.,1.));
#25579=DIRECTION('center_axis',(0.,0.,1.));
#25580=DIRECTION('ref_axis',(1.,2.60858704573983E-14,0.));
#25581=DIRECTION('',(0.,0.,1.));
#25582=DIRECTION('center_axis',(0.,0.,1.));
#25583=DIRECTION('ref_axis',(1.,2.60858704573983E-14,0.));
#25584=DIRECTION('',(0.,0.,1.));
#25585=DIRECTION('center_axis',(0.,0.,1.));
#25586=DIRECTION('ref_axis',(1.,2.60858704573983E-14,0.));
#25587=DIRECTION('',(0.,0.,1.));
#25588=DIRECTION('center_axis',(0.,0.,1.));
#25589=DIRECTION('ref_axis',(1.,2.60858704573983E-14,0.));
#25590=DIRECTION('',(0.,0.,1.));
#25591=DIRECTION('center_axis',(0.,0.,1.));
#25592=DIRECTION('ref_axis',(1.,2.60858704573983E-14,0.));
#25593=DIRECTION('',(0.,0.,1.));
#25594=DIRECTION('center_axis',(0.,0.,-1.));
#25595=DIRECTION('ref_axis',(1.,2.60858704573983E-14,0.));
#25596=DIRECTION('center_axis',(0.,0.,1.));
#25597=DIRECTION('ref_axis',(1.,0.,0.));
#25598=DIRECTION('center_axis',(0.,0.,1.));
#25599=DIRECTION('ref_axis',(1.,0.,0.));
#25600=DIRECTION('center_axis',(0.,0.,1.));
#25601=DIRECTION('ref_axis',(1.,0.,0.));
#25602=DIRECTION('center_axis',(0.,0.,-1.));
#25603=DIRECTION('ref_axis',(1.,2.60858704573983E-14,0.));
#25604=DIRECTION('center_axis',(0.,0.,1.));
#25605=DIRECTION('ref_axis',(-0.997062769070685,0.0765887363330732,0.));
#25606=DIRECTION('center_axis',(0.866025403784439,0.5,0.));
#25607=DIRECTION('ref_axis',(0.5,-0.866025403784439,0.));
#25608=DIRECTION('',(0.5,-0.866025403784439,0.));
#25609=DIRECTION('',(0.,0.,-1.));
#25610=DIRECTION('',(0.5,-0.866025403784439,0.));
#25611=DIRECTION('',(0.,0.,-1.));
#25612=DIRECTION('center_axis',(1.20185167898973E-16,1.,0.));
#25613=DIRECTION('ref_axis',(1.,-1.20185167898973E-16,0.));
#25614=DIRECTION('',(1.,-1.20185167898973E-16,0.));
#25615=DIRECTION('',(0.,0.,-1.));
#25616=DIRECTION('',(1.,-1.20185167898973E-16,0.));
#25617=DIRECTION('center_axis',(-0.866025403784439,0.5,0.));
#25618=DIRECTION('ref_axis',(0.5,0.866025403784439,0.));
#25619=DIRECTION('',(0.5,0.866025403784439,0.));
#25620=DIRECTION('',(0.,0.,-1.));
#25621=DIRECTION('',(0.5,0.866025403784439,0.));
#25622=DIRECTION('center_axis',(-0.866025403784439,-0.5,0.));
#25623=DIRECTION('ref_axis',(-0.5,0.866025403784439,0.));
#25624=DIRECTION('',(-0.5,0.866025403784439,0.));
#25625=DIRECTION('',(0.,0.,-1.));
#25626=DIRECTION('',(-0.5,0.866025403784439,0.));
#25627=DIRECTION('center_axis',(-2.40370335797945E-16,-1.,0.));
#25628=DIRECTION('ref_axis',(-1.,2.40370335797945E-16,0.));
#25629=DIRECTION('',(-1.,2.40370335797945E-16,0.));
#25630=DIRECTION('',(0.,0.,-1.));
#25631=DIRECTION('',(-1.,2.40370335797945E-16,0.));
#25632=DIRECTION('center_axis',(0.866025403784439,-0.5,0.));
#25633=DIRECTION('ref_axis',(-0.5,-0.866025403784439,0.));
#25634=DIRECTION('',(-0.5,-0.866025403784439,0.));
#25635=DIRECTION('',(-0.5,-0.866025403784439,0.));
#25636=DIRECTION('center_axis',(0.,0.,-1.));
#25637=DIRECTION('ref_axis',(-1.,0.,0.));
#25638=DIRECTION('center_axis',(-0.890221906442363,-0.455527120257538,0.));
#25639=DIRECTION('ref_axis',(-0.455527120257538,0.890221906442363,0.));
#25640=DIRECTION('',(0.,0.,1.));
#25641=DIRECTION('',(-0.455527120257538,0.890221906442363,0.));
#25642=DIRECTION('',(0.,0.,-1.));
#25643=DIRECTION('',(-0.455527120257538,0.890221906442363,0.));
#25644=DIRECTION('center_axis',(0.,0.,1.));
#25645=DIRECTION('ref_axis',(1.,0.,0.));
#25646=DIRECTION('center_axis',(0.,0.,1.));
#25647=DIRECTION('ref_axis',(1.,0.,0.));
#25648=DIRECTION('',(0.966370941490094,0.257152101767709,0.));
#25649=DIRECTION('center_axis',(-0.257152101767709,0.966370941490094,0.));
#25650=DIRECTION('ref_axis',(0.966370941490094,0.257152101767709,0.));
#25651=DIRECTION('',(0.,0.,-1.));
#25652=DIRECTION('',(0.966370941490094,0.257152101767709,0.));
#25653=DIRECTION('center_axis',(0.,0.,-1.));
#25654=DIRECTION('ref_axis',(-1.,0.,0.));
#25655=DIRECTION('center_axis',(0.,0.,-1.));
#25656=DIRECTION('ref_axis',(1.,0.,0.));
#25657=DIRECTION('center_axis',(-0.998537750647894,-0.0540588617253913,
0.));
#25658=DIRECTION('ref_axis',(-0.0540588617253913,0.998537750647894,0.));
#25659=DIRECTION('',(0.,0.,1.));
#25660=DIRECTION('',(-0.0540588617253913,0.998537750647894,0.));
#25661=DIRECTION('',(0.,0.,-1.));
#25662=DIRECTION('',(-0.0540588617253913,0.998537750647894,0.));
#25663=DIRECTION('center_axis',(0.,0.,1.));
#25664=DIRECTION('ref_axis',(1.,0.,0.));
#25665=DIRECTION('center_axis',(0.,0.,1.));
#25666=DIRECTION('ref_axis',(1.,0.,0.));
#25667=DIRECTION('',(0.987416966628963,-0.158138338214543,0.));
#25668=DIRECTION('center_axis',(0.158138338214543,0.987416966628963,0.));
#25669=DIRECTION('ref_axis',(0.987416966628963,-0.158138338214543,0.));
#25670=DIRECTION('',(0.,0.,-1.));
#25671=DIRECTION('',(0.987416966628963,-0.158138338214543,0.));
#25672=DIRECTION('center_axis',(0.,0.,-1.));
#25673=DIRECTION('ref_axis',(-1.,0.,0.));
#25674=DIRECTION('center_axis',(0.,0.,-1.));
#25675=DIRECTION('ref_axis',(1.,0.,0.));
#25676=DIRECTION('center_axis',(-0.934197346335725,0.356756665108433,0.));
#25677=DIRECTION('ref_axis',(0.356756665108433,0.934197346335725,0.));
#25678=DIRECTION('',(0.,0.,1.));
#25679=DIRECTION('',(0.356756665108433,0.934197346335725,0.));
#25680=DIRECTION('',(0.,0.,-1.));
#25681=DIRECTION('',(0.356756665108433,0.934197346335725,0.));
#25682=DIRECTION('center_axis',(0.,0.,1.));
#25683=DIRECTION('ref_axis',(1.,0.,0.));
#25684=DIRECTION('center_axis',(0.,0.,1.));
#25685=DIRECTION('ref_axis',(1.,0.,0.));
#25686=DIRECTION('',(0.837729627836157,-0.546085222877798,0.));
#25687=DIRECTION('center_axis',(0.546085222877798,0.837729627836157,0.));
#25688=DIRECTION('ref_axis',(0.837729627836157,-0.546085222877798,0.));
#25689=DIRECTION('',(0.,0.,-1.));
#25690=DIRECTION('',(0.837729627836157,-0.546085222877798,0.));
#25691=DIRECTION('center_axis',(0.,0.,-1.));
#25692=DIRECTION('ref_axis',(-1.,0.,0.));
#25693=DIRECTION('center_axis',(0.,0.,-1.));
#25694=DIRECTION('ref_axis',(1.,0.,0.));
#25695=DIRECTION('center_axis',(-0.708325733925652,0.705885723512444,0.));
#25696=DIRECTION('ref_axis',(0.705885723512444,0.708325733925652,0.));
#25697=DIRECTION('',(0.,0.,1.));
#25698=DIRECTION('',(0.705885723512444,0.708325733925652,0.));
#25699=DIRECTION('',(0.,0.,-1.));
#25700=DIRECTION('',(0.705885723512444,0.708325733925652,0.));
#25701=DIRECTION('center_axis',(0.,0.,1.));
#25702=DIRECTION('ref_axis',(1.,0.,0.));
#25703=DIRECTION('center_axis',(0.,0.,1.));
#25704=DIRECTION('ref_axis',(1.,0.,0.));
#25705=DIRECTION('',(0.543191225855731,-0.839609011476978,0.));
#25706=DIRECTION('center_axis',(0.839609011476978,0.543191225855731,0.));
#25707=DIRECTION('ref_axis',(0.543191225855731,-0.839609011476978,0.));
#25708=DIRECTION('',(0.,0.,-1.));
#25709=DIRECTION('',(0.543191225855731,-0.839609011476978,0.));
#25710=DIRECTION('center_axis',(0.,0.,-1.));
#25711=DIRECTION('ref_axis',(-1.,0.,0.));
#25712=DIRECTION('center_axis',(0.,0.,-1.));
#25713=DIRECTION('ref_axis',(1.,0.,0.));
#25714=DIRECTION('center_axis',(-0.359978167182565,0.932960727550673,0.));
#25715=DIRECTION('ref_axis',(0.932960727550673,0.359978167182565,0.));
#25716=DIRECTION('',(0.,0.,1.));
#25717=DIRECTION('',(0.932960727550673,0.359978167182565,0.));
#25718=DIRECTION('',(0.,0.,-1.));
#25719=DIRECTION('',(0.932960727550673,0.359978167182565,0.));
#25720=DIRECTION('center_axis',(0.,0.,1.));
#25721=DIRECTION('ref_axis',(1.,0.,0.));
#25722=DIRECTION('center_axis',(0.,0.,1.));
#25723=DIRECTION('ref_axis',(1.,0.,0.));
#25724=DIRECTION('',(0.154730126187482,-0.987956774383376,0.));
#25725=DIRECTION('center_axis',(0.987956774383376,0.154730126187482,0.));
#25726=DIRECTION('ref_axis',(0.154730126187482,-0.987956774383376,0.));
#25727=DIRECTION('',(0.,0.,-1.));
#25728=DIRECTION('',(0.154730126187482,-0.987956774383376,0.));
#25729=DIRECTION('center_axis',(0.,0.,-1.));
#25730=DIRECTION('ref_axis',(-1.,0.,0.));
#25731=DIRECTION('center_axis',(0.,0.,-1.));
#25732=DIRECTION('ref_axis',(1.,0.,0.));
#25733=DIRECTION('center_axis',(0.0506128949653782,0.998718346113269,0.));
#25734=DIRECTION('ref_axis',(0.998718346113269,-0.0506128949653782,0.));
#25735=DIRECTION('',(0.,0.,1.));
#25736=DIRECTION('',(0.998718346113269,-0.0506128949653782,0.));
#25737=DIRECTION('',(0.,0.,-1.));
#25738=DIRECTION('',(0.998718346113269,-0.0506128949653782,0.));
#25739=DIRECTION('center_axis',(0.,0.,1.));
#25740=DIRECTION('ref_axis',(1.,0.,0.));
#25741=DIRECTION('center_axis',(0.,0.,1.));
#25742=DIRECTION('ref_axis',(1.,0.,0.));
#25743=DIRECTION('',(-0.260485217977654,-0.96547783569336,0.));
#25744=DIRECTION('center_axis',(0.96547783569336,-0.260485217977654,0.));
#25745=DIRECTION('ref_axis',(-0.260485217977654,-0.96547783569336,0.));
#25746=DIRECTION('',(0.,0.,-1.));
#25747=DIRECTION('',(-0.260485217977654,-0.96547783569336,0.));
#25748=DIRECTION('center_axis',(0.,0.,-1.));
#25749=DIRECTION('ref_axis',(-1.,0.,0.));
#25750=DIRECTION('center_axis',(0.,0.,-1.));
#25751=DIRECTION('ref_axis',(1.,0.,0.));
#25752=DIRECTION('center_axis',(0.452452527770092,0.891788489561541,0.));
#25753=DIRECTION('ref_axis',(0.891788489561541,-0.452452527770092,0.));
#25754=DIRECTION('',(0.,0.,1.));
#25755=DIRECTION('',(0.891788489561541,-0.452452527770092,0.));
#25756=DIRECTION('',(0.,0.,-1.));
#25757=DIRECTION('',(0.891788489561541,-0.452452527770092,0.));
#25758=DIRECTION('center_axis',(0.,0.,1.));
#25759=DIRECTION('ref_axis',(1.,0.,0.));
#25760=DIRECTION('center_axis',(0.,0.,1.));
#25761=DIRECTION('ref_axis',(1.,0.,0.));
#25762=DIRECTION('',(-0.630660301520536,-0.776059008121178,0.));
#25763=DIRECTION('center_axis',(0.776059008121178,-0.630660301520536,0.));
#25764=DIRECTION('ref_axis',(-0.630660301520536,-0.776059008121178,0.));
#25765=DIRECTION('',(0.,0.,-1.));
#25766=DIRECTION('',(-0.630660301520536,-0.776059008121178,0.));
#25767=DIRECTION('center_axis',(0.,0.,-1.));
#25768=DIRECTION('ref_axis',(-1.,0.,0.));
#25769=DIRECTION('center_axis',(0.,0.,-1.));
#25770=DIRECTION('ref_axis',(1.,0.,0.));
#25771=DIRECTION('center_axis',(0.,0.,1.));
#25772=DIRECTION('ref_axis',(1.,0.,0.));
#25773=DIRECTION('center_axis',(0.,0.,1.));
#25774=DIRECTION('ref_axis',(1.,0.,0.));
#25775=DIRECTION('',(-0.778230601363197,0.627978607200816,0.));
#25776=DIRECTION('',(0.778230601363197,0.627978607200816,0.));
#25777=DIRECTION('center_axis',(-0.627978607200816,-0.778230601363197,0.));
#25778=DIRECTION('ref_axis',(-0.778230601363197,0.627978607200816,0.));
#25779=DIRECTION('',(0.,0.,1.));
#25780=DIRECTION('',(-0.778230601363197,0.627978607200816,0.));
#25781=DIRECTION('',(0.,0.,-1.));
#25782=DIRECTION('center_axis',(-0.627978607200816,0.778230601363197,0.));
#25783=DIRECTION('ref_axis',(0.778230601363197,0.627978607200816,0.));
#25784=DIRECTION('',(0.,0.,-1.));
#25785=DIRECTION('',(0.778230601363197,0.627978607200816,0.));
#25786=DIRECTION('center_axis',(0.,0.,-1.));
#25787=DIRECTION('ref_axis',(-1.,0.,0.));
#25788=DIRECTION('center_axis',(0.,0.,-1.));
#25789=DIRECTION('ref_axis',(1.,0.,0.));
#25790=DIRECTION('center_axis',(0.89022190644236,0.455527120257544,0.));
#25791=DIRECTION('ref_axis',(0.455527120257544,-0.89022190644236,0.));
#25792=DIRECTION('',(0.,0.,1.));
#25793=DIRECTION('',(0.455527120257544,-0.89022190644236,0.));
#25794=DIRECTION('',(0.,0.,-1.));
#25795=DIRECTION('',(0.455527120257544,-0.89022190644236,0.));
#25796=DIRECTION('center_axis',(0.,0.,1.));
#25797=DIRECTION('ref_axis',(1.,0.,0.));
#25798=DIRECTION('center_axis',(0.,0.,1.));
#25799=DIRECTION('ref_axis',(1.,0.,0.));
#25800=DIRECTION('',(-0.966370941490095,-0.257152101767705,0.));
#25801=DIRECTION('center_axis',(0.257152101767705,-0.966370941490095,0.));
#25802=DIRECTION('ref_axis',(-0.966370941490095,-0.257152101767705,0.));
#25803=DIRECTION('',(0.,0.,-1.));
#25804=DIRECTION('',(-0.966370941490095,-0.257152101767705,0.));
#25805=DIRECTION('center_axis',(0.,0.,-1.));
#25806=DIRECTION('ref_axis',(-1.,0.,0.));
#25807=DIRECTION('center_axis',(0.,0.,-1.));
#25808=DIRECTION('ref_axis',(1.,0.,0.));
#25809=DIRECTION('center_axis',(0.998537750647894,0.0540588617253865,0.));
#25810=DIRECTION('ref_axis',(0.0540588617253865,-0.998537750647894,0.));
#25811=DIRECTION('',(0.,0.,1.));
#25812=DIRECTION('',(0.0540588617253865,-0.998537750647894,0.));
#25813=DIRECTION('',(0.,0.,-1.));
#25814=DIRECTION('',(0.0540588617253865,-0.998537750647894,0.));
#25815=DIRECTION('center_axis',(0.,0.,1.));
#25816=DIRECTION('ref_axis',(1.,0.,0.));
#25817=DIRECTION('center_axis',(0.,0.,1.));
#25818=DIRECTION('ref_axis',(1.,0.,0.));
#25819=DIRECTION('',(-0.987416966628962,0.15813833821455,0.));
#25820=DIRECTION('center_axis',(-0.15813833821455,-0.987416966628962,0.));
#25821=DIRECTION('ref_axis',(-0.987416966628962,0.15813833821455,0.));
#25822=DIRECTION('',(0.,0.,-1.));
#25823=DIRECTION('',(-0.987416966628962,0.15813833821455,0.));
#25824=DIRECTION('center_axis',(0.,0.,-1.));
#25825=DIRECTION('ref_axis',(-1.,0.,0.));
#25826=DIRECTION('center_axis',(0.,0.,-1.));
#25827=DIRECTION('ref_axis',(1.,0.,0.));
#25828=DIRECTION('center_axis',(0.934197346335727,-0.356756665108427,0.));
#25829=DIRECTION('ref_axis',(-0.356756665108427,-0.934197346335727,0.));
#25830=DIRECTION('',(0.,0.,1.));
#25831=DIRECTION('',(-0.356756665108427,-0.934197346335727,0.));
#25832=DIRECTION('',(0.,0.,-1.));
#25833=DIRECTION('',(-0.356756665108427,-0.934197346335727,0.));
#25834=DIRECTION('center_axis',(0.,0.,1.));
#25835=DIRECTION('ref_axis',(1.,0.,0.));
#25836=DIRECTION('center_axis',(0.,0.,1.));
#25837=DIRECTION('ref_axis',(1.,0.,0.));
#25838=DIRECTION('',(-0.837729627836154,0.546085222877803,0.));
#25839=DIRECTION('center_axis',(-0.546085222877803,-0.837729627836154,0.));
#25840=DIRECTION('ref_axis',(-0.837729627836154,0.546085222877803,0.));
#25841=DIRECTION('',(0.,0.,-1.));
#25842=DIRECTION('',(-0.837729627836154,0.546085222877803,0.));
#25843=DIRECTION('center_axis',(0.,0.,-1.));
#25844=DIRECTION('ref_axis',(-1.,0.,0.));
#25845=DIRECTION('center_axis',(0.,0.,-1.));
#25846=DIRECTION('ref_axis',(1.,0.,0.));
#25847=DIRECTION('center_axis',(0.708325733925657,-0.70588572351244,0.));
#25848=DIRECTION('ref_axis',(-0.70588572351244,-0.708325733925657,0.));
#25849=DIRECTION('',(0.,0.,1.));
#25850=DIRECTION('',(-0.70588572351244,-0.708325733925657,0.));
#25851=DIRECTION('',(0.,0.,-1.));
#25852=DIRECTION('',(-0.70588572351244,-0.708325733925657,0.));
#25853=DIRECTION('center_axis',(0.,0.,1.));
#25854=DIRECTION('ref_axis',(1.,0.,0.));
#25855=DIRECTION('center_axis',(0.,0.,1.));
#25856=DIRECTION('ref_axis',(1.,0.,0.));
#25857=DIRECTION('',(-0.543191225855725,0.839609011476982,0.));
#25858=DIRECTION('center_axis',(-0.839609011476982,-0.543191225855725,0.));
#25859=DIRECTION('ref_axis',(-0.543191225855725,0.839609011476982,0.));
#25860=DIRECTION('',(0.,0.,-1.));
#25861=DIRECTION('',(-0.543191225855725,0.839609011476982,0.));
#25862=DIRECTION('center_axis',(0.,0.,-1.));
#25863=DIRECTION('ref_axis',(-1.,0.,0.));
#25864=DIRECTION('center_axis',(0.,0.,-1.));
#25865=DIRECTION('ref_axis',(1.,0.,0.));
#25866=DIRECTION('center_axis',(0.359978167182562,-0.932960727550674,0.));
#25867=DIRECTION('ref_axis',(-0.932960727550674,-0.359978167182562,0.));
#25868=DIRECTION('',(0.,0.,1.));
#25869=DIRECTION('',(-0.932960727550674,-0.359978167182562,0.));
#25870=DIRECTION('',(0.,0.,-1.));
#25871=DIRECTION('',(-0.932960727550674,-0.359978167182562,0.));
#25872=DIRECTION('center_axis',(0.,0.,1.));
#25873=DIRECTION('ref_axis',(1.,0.,0.));
#25874=DIRECTION('center_axis',(0.,0.,1.));
#25875=DIRECTION('ref_axis',(1.,0.,0.));
#25876=DIRECTION('',(-0.154730126187479,0.987956774383377,0.));
#25877=DIRECTION('center_axis',(-0.987956774383377,-0.154730126187479,0.));
#25878=DIRECTION('ref_axis',(-0.154730126187479,0.987956774383377,0.));
#25879=DIRECTION('',(0.,0.,-1.));
#25880=DIRECTION('',(-0.154730126187479,0.987956774383377,0.));
#25881=DIRECTION('center_axis',(0.,0.,-1.));
#25882=DIRECTION('ref_axis',(-1.,0.,0.));
#25883=DIRECTION('center_axis',(0.,0.,-1.));
#25884=DIRECTION('ref_axis',(1.,0.,0.));
#25885=DIRECTION('center_axis',(-0.0506128949653805,-0.998718346113269,
0.));
#25886=DIRECTION('ref_axis',(-0.998718346113269,0.0506128949653805,0.));
#25887=DIRECTION('',(0.,0.,1.));
#25888=DIRECTION('',(-0.998718346113269,0.0506128949653805,0.));
#25889=DIRECTION('',(0.,0.,-1.));
#25890=DIRECTION('',(-0.998718346113269,0.0506128949653805,0.));
#25891=DIRECTION('center_axis',(0.,0.,1.));
#25892=DIRECTION('ref_axis',(1.,0.,0.));
#25893=DIRECTION('center_axis',(0.,0.,1.));
#25894=DIRECTION('ref_axis',(1.,0.,0.));
#25895=DIRECTION('',(0.260485217977653,0.96547783569336,0.));
#25896=DIRECTION('center_axis',(-0.96547783569336,0.260485217977653,0.));
#25897=DIRECTION('ref_axis',(0.260485217977653,0.96547783569336,0.));
#25898=DIRECTION('',(0.,0.,-1.));
#25899=DIRECTION('',(0.260485217977653,0.96547783569336,0.));
#25900=DIRECTION('center_axis',(0.,0.,-1.));
#25901=DIRECTION('ref_axis',(-1.,0.,0.));
#25902=DIRECTION('center_axis',(0.,0.,-1.));
#25903=DIRECTION('ref_axis',(1.,0.,0.));
#25904=DIRECTION('center_axis',(-0.452452527770092,-0.891788489561541,0.));
#25905=DIRECTION('ref_axis',(-0.891788489561541,0.452452527770092,0.));
#25906=DIRECTION('',(0.,0.,1.));
#25907=DIRECTION('',(-0.891788489561541,0.452452527770092,0.));
#25908=DIRECTION('',(0.,0.,-1.));
#25909=DIRECTION('',(-0.891788489561541,0.452452527770092,0.));
#25910=DIRECTION('center_axis',(0.,0.,1.));
#25911=DIRECTION('ref_axis',(1.,0.,0.));
#25912=DIRECTION('center_axis',(0.,0.,1.));
#25913=DIRECTION('ref_axis',(1.,0.,0.));
#25914=DIRECTION('',(0.630660301520534,0.77605900812118,0.));
#25915=DIRECTION('center_axis',(-0.77605900812118,0.630660301520534,0.));
#25916=DIRECTION('ref_axis',(0.630660301520534,0.77605900812118,0.));
#25917=DIRECTION('',(0.,0.,-1.));
#25918=DIRECTION('',(0.630660301520534,0.77605900812118,0.));
#25919=DIRECTION('center_axis',(0.,0.,-1.));
#25920=DIRECTION('ref_axis',(-1.,0.,0.));
#25921=DIRECTION('center_axis',(0.,0.,-1.));
#25922=DIRECTION('ref_axis',(1.,0.,0.));
#25923=DIRECTION('center_axis',(-0.257152101767705,-0.966370941490095,0.));
#25924=DIRECTION('ref_axis',(-0.966370941490095,0.257152101767705,0.));
#25925=DIRECTION('',(0.,0.,1.));
#25926=DIRECTION('',(-0.966370941490095,0.257152101767705,0.));
#25927=DIRECTION('',(0.,0.,-1.));
#25928=DIRECTION('',(-0.966370941490095,0.257152101767705,0.));
#25929=DIRECTION('center_axis',(0.,0.,1.));
#25930=DIRECTION('ref_axis',(1.,0.,0.));
#25931=DIRECTION('center_axis',(0.,0.,1.));
#25932=DIRECTION('ref_axis',(1.,0.,0.));
#25933=DIRECTION('',(0.455527120257543,0.89022190644236,0.));
#25934=DIRECTION('center_axis',(-0.89022190644236,0.455527120257543,0.));
#25935=DIRECTION('ref_axis',(0.455527120257543,0.89022190644236,0.));
#25936=DIRECTION('',(0.,0.,-1.));
#25937=DIRECTION('',(0.455527120257543,0.89022190644236,0.));
#25938=DIRECTION('center_axis',(0.,0.,-1.));
#25939=DIRECTION('ref_axis',(-1.,0.,0.));
#25940=DIRECTION('center_axis',(0.,0.,-1.));
#25941=DIRECTION('ref_axis',(1.,0.,0.));
#25942=DIRECTION('center_axis',(0.158138338214546,-0.987416966628963,0.));
#25943=DIRECTION('ref_axis',(-0.987416966628963,-0.158138338214546,0.));
#25944=DIRECTION('',(0.,0.,1.));
#25945=DIRECTION('',(-0.987416966628963,-0.158138338214546,0.));
#25946=DIRECTION('',(0.,0.,-1.));
#25947=DIRECTION('',(-0.987416966628963,-0.158138338214546,0.));
#25948=DIRECTION('center_axis',(0.,0.,1.));
#25949=DIRECTION('ref_axis',(1.,0.,0.));
#25950=DIRECTION('center_axis',(0.,0.,1.));
#25951=DIRECTION('ref_axis',(1.,0.,0.));
#25952=DIRECTION('',(0.0540588617253865,0.998537750647894,0.));
#25953=DIRECTION('center_axis',(-0.998537750647894,0.0540588617253865,0.));
#25954=DIRECTION('ref_axis',(0.0540588617253865,0.998537750647894,0.));
#25955=DIRECTION('',(0.,0.,-1.));
#25956=DIRECTION('',(0.0540588617253865,0.998537750647894,0.));
#25957=DIRECTION('center_axis',(0.,0.,-1.));
#25958=DIRECTION('ref_axis',(-1.,0.,0.));
#25959=DIRECTION('center_axis',(0.,0.,-1.));
#25960=DIRECTION('ref_axis',(1.,0.,0.));
#25961=DIRECTION('center_axis',(0.546085222877805,-0.837729627836152,0.));
#25962=DIRECTION('ref_axis',(-0.837729627836152,-0.546085222877805,0.));
#25963=DIRECTION('',(0.,0.,1.));
#25964=DIRECTION('',(-0.837729627836152,-0.546085222877805,0.));
#25965=DIRECTION('',(0.,0.,-1.));
#25966=DIRECTION('',(-0.837729627836152,-0.546085222877805,0.));
#25967=DIRECTION('center_axis',(0.,0.,1.));
#25968=DIRECTION('ref_axis',(1.,0.,0.));
#25969=DIRECTION('center_axis',(0.,0.,1.));
#25970=DIRECTION('ref_axis',(1.,0.,0.));
#25971=DIRECTION('',(-0.356756665108427,0.934197346335727,0.));
#25972=DIRECTION('center_axis',(-0.934197346335727,-0.356756665108427,0.));
#25973=DIRECTION('ref_axis',(-0.356756665108427,0.934197346335727,0.));
#25974=DIRECTION('',(0.,0.,-1.));
#25975=DIRECTION('',(-0.356756665108427,0.934197346335727,0.));
#25976=DIRECTION('center_axis',(0.,0.,-1.));
#25977=DIRECTION('ref_axis',(-1.,0.,0.));
#25978=DIRECTION('center_axis',(0.,0.,-1.));
#25979=DIRECTION('ref_axis',(1.,0.,0.));
#25980=DIRECTION('center_axis',(0.839609011476981,-0.543191225855727,0.));
#25981=DIRECTION('ref_axis',(-0.543191225855727,-0.839609011476981,0.));
#25982=DIRECTION('',(0.,0.,1.));
#25983=DIRECTION('',(-0.543191225855727,-0.839609011476981,0.));
#25984=DIRECTION('',(0.,0.,-1.));
#25985=DIRECTION('',(-0.543191225855727,-0.839609011476981,0.));
#25986=DIRECTION('center_axis',(0.,0.,1.));
#25987=DIRECTION('ref_axis',(1.,0.,0.));
#25988=DIRECTION('center_axis',(0.,0.,1.));
#25989=DIRECTION('ref_axis',(1.,0.,0.));
#25990=DIRECTION('',(-0.70588572351244,0.708325733925656,0.));
#25991=DIRECTION('center_axis',(-0.708325733925656,-0.70588572351244,0.));
#25992=DIRECTION('ref_axis',(-0.70588572351244,0.708325733925656,0.));
#25993=DIRECTION('',(0.,0.,-1.));
#25994=DIRECTION('',(-0.70588572351244,0.708325733925656,0.));
#25995=DIRECTION('center_axis',(0.,0.,-1.));
#25996=DIRECTION('ref_axis',(-1.,0.,0.));
#25997=DIRECTION('center_axis',(0.,0.,-1.));
#25998=DIRECTION('ref_axis',(1.,0.,0.));
#25999=DIRECTION('center_axis',(0.987956774383378,-0.154730126187475,0.));
#26000=DIRECTION('ref_axis',(-0.154730126187475,-0.987956774383378,0.));
#26001=DIRECTION('',(0.,0.,1.));
#26002=DIRECTION('',(-0.154730126187475,-0.987956774383378,0.));
#26003=DIRECTION('',(0.,0.,-1.));
#26004=DIRECTION('',(-0.154730126187475,-0.987956774383378,0.));
#26005=DIRECTION('center_axis',(0.,0.,1.));
#26006=DIRECTION('ref_axis',(1.,0.,0.));
#26007=DIRECTION('center_axis',(0.,0.,1.));
#26008=DIRECTION('ref_axis',(1.,0.,0.));
#26009=DIRECTION('',(-0.932960727550675,0.359978167182561,0.));
#26010=DIRECTION('center_axis',(-0.359978167182561,-0.932960727550675,0.));
#26011=DIRECTION('ref_axis',(-0.932960727550675,0.359978167182561,0.));
#26012=DIRECTION('',(0.,0.,-1.));
#26013=DIRECTION('',(-0.932960727550675,0.359978167182561,0.));
#26014=DIRECTION('center_axis',(0.,0.,-1.));
#26015=DIRECTION('ref_axis',(-1.,0.,0.));
#26016=DIRECTION('center_axis',(0.,0.,-1.));
#26017=DIRECTION('ref_axis',(1.,0.,0.));
#26018=DIRECTION('center_axis',(0.965477835693359,0.260485217977657,0.));
#26019=DIRECTION('ref_axis',(0.260485217977657,-0.965477835693359,0.));
#26020=DIRECTION('',(0.,0.,1.));
#26021=DIRECTION('',(0.260485217977657,-0.965477835693359,0.));
#26022=DIRECTION('',(0.,0.,-1.));
#26023=DIRECTION('',(0.260485217977657,-0.965477835693359,0.));
#26024=DIRECTION('center_axis',(0.,0.,1.));
#26025=DIRECTION('ref_axis',(1.,0.,0.));
#26026=DIRECTION('center_axis',(0.,0.,1.));
#26027=DIRECTION('ref_axis',(1.,0.,0.));
#26028=DIRECTION('',(-0.998718346113269,-0.0506128949653804,0.));
#26029=DIRECTION('center_axis',(0.0506128949653804,-0.998718346113269,0.));
#26030=DIRECTION('ref_axis',(-0.998718346113269,-0.0506128949653804,0.));
#26031=DIRECTION('',(0.,0.,-1.));
#26032=DIRECTION('',(-0.998718346113269,-0.0506128949653804,0.));
#26033=DIRECTION('center_axis',(0.,0.,-1.));
#26034=DIRECTION('ref_axis',(-1.,0.,0.));
#26035=DIRECTION('center_axis',(0.,0.,-1.));
#26036=DIRECTION('ref_axis',(1.,0.,0.));
#26037=DIRECTION('center_axis',(0.77605900812118,0.630660301520534,0.));
#26038=DIRECTION('ref_axis',(0.630660301520534,-0.77605900812118,0.));
#26039=DIRECTION('',(0.,0.,1.));
#26040=DIRECTION('',(0.630660301520534,-0.77605900812118,0.));
#26041=DIRECTION('',(0.,0.,-1.));
#26042=DIRECTION('',(0.630660301520534,-0.77605900812118,0.));
#26043=DIRECTION('center_axis',(0.,0.,1.));
#26044=DIRECTION('ref_axis',(1.,0.,0.));
#26045=DIRECTION('center_axis',(0.,0.,1.));
#26046=DIRECTION('ref_axis',(1.,0.,0.));
#26047=DIRECTION('',(-0.891788489561542,-0.452452527770089,0.));
#26048=DIRECTION('center_axis',(0.452452527770089,-0.891788489561542,0.));
#26049=DIRECTION('ref_axis',(-0.891788489561542,-0.452452527770089,0.));
#26050=DIRECTION('',(0.,0.,-1.));
#26051=DIRECTION('',(-0.891788489561542,-0.452452527770089,0.));
#26052=DIRECTION('center_axis',(0.,0.,-1.));
#26053=DIRECTION('ref_axis',(-1.,0.,0.));
#26054=DIRECTION('center_axis',(0.,0.,-1.));
#26055=DIRECTION('ref_axis',(1.,0.,0.));
#26056=DIRECTION('center_axis',(0.627978607200814,0.778230601363199,0.));
#26057=DIRECTION('ref_axis',(0.778230601363199,-0.627978607200814,0.));
#26058=DIRECTION('',(0.,0.,1.));
#26059=DIRECTION('',(0.778230601363199,-0.627978607200814,0.));
#26060=DIRECTION('',(0.,0.,-1.));
#26061=DIRECTION('',(0.778230601363199,-0.627978607200814,0.));
#26062=DIRECTION('center_axis',(0.,0.,1.));
#26063=DIRECTION('ref_axis',(1.,0.,0.));
#26064=DIRECTION('center_axis',(0.,0.,1.));
#26065=DIRECTION('ref_axis',(1.,0.,0.));
#26066=DIRECTION('',(-0.778230601363197,-0.627978607200817,0.));
#26067=DIRECTION('center_axis',(0.,0.,1.));
#26068=DIRECTION('ref_axis',(1.,0.,0.));
#26069=DIRECTION('center_axis',(0.627978607200817,-0.778230601363197,0.));
#26070=DIRECTION('ref_axis',(-0.778230601363197,-0.627978607200817,0.));
#26071=DIRECTION('',(0.,0.,-1.));
#26072=DIRECTION('',(-0.778230601363197,-0.627978607200817,0.));
#26073=DIRECTION('center_axis',(0.,0.,-1.));
#26074=DIRECTION('ref_axis',(-1.,0.,0.));
#26075=DIRECTION('center_axis',(0.,0.,-1.));
#26076=DIRECTION('ref_axis',(1.,0.,0.));
#26077=DIRECTION('center_axis',(0.,0.,-1.));
#26078=DIRECTION('ref_axis',(1.,0.,0.));
#26079=DIRECTION('center_axis',(0.257152101767705,0.966370941490095,0.));
#26080=DIRECTION('ref_axis',(0.966370941490095,-0.257152101767705,0.));
#26081=DIRECTION('',(0.,0.,1.));
#26082=DIRECTION('',(0.966370941490095,-0.257152101767705,0.));
#26083=DIRECTION('',(0.,0.,-1.));
#26084=DIRECTION('',(0.966370941490095,-0.257152101767705,0.));
#26085=DIRECTION('center_axis',(0.,0.,1.));
#26086=DIRECTION('ref_axis',(1.,0.,0.));
#26087=DIRECTION('center_axis',(0.,0.,1.));
#26088=DIRECTION('ref_axis',(1.,0.,0.));
#26089=DIRECTION('',(-0.455527120257545,-0.890221906442359,0.));
#26090=DIRECTION('center_axis',(0.890221906442359,-0.455527120257545,0.));
#26091=DIRECTION('ref_axis',(-0.455527120257545,-0.890221906442359,0.));
#26092=DIRECTION('',(0.,0.,-1.));
#26093=DIRECTION('',(-0.455527120257545,-0.890221906442359,0.));
#26094=DIRECTION('center_axis',(0.,0.,-1.));
#26095=DIRECTION('ref_axis',(-1.,0.,0.));
#26096=DIRECTION('center_axis',(0.,0.,-1.));
#26097=DIRECTION('ref_axis',(1.,0.,0.));
#26098=DIRECTION('center_axis',(-0.158138338214545,0.987416966628963,0.));
#26099=DIRECTION('ref_axis',(0.987416966628963,0.158138338214545,0.));
#26100=DIRECTION('',(0.,0.,1.));
#26101=DIRECTION('',(0.987416966628963,0.158138338214545,0.));
#26102=DIRECTION('',(0.,0.,-1.));
#26103=DIRECTION('',(0.987416966628963,0.158138338214545,0.));
#26104=DIRECTION('center_axis',(0.,0.,1.));
#26105=DIRECTION('ref_axis',(1.,0.,0.));
#26106=DIRECTION('center_axis',(0.,0.,1.));
#26107=DIRECTION('ref_axis',(1.,0.,0.));
#26108=DIRECTION('',(-0.054058861725389,-0.998537750647894,0.));
#26109=DIRECTION('center_axis',(0.998537750647894,-0.054058861725389,0.));
#26110=DIRECTION('ref_axis',(-0.054058861725389,-0.998537750647894,0.));
#26111=DIRECTION('',(0.,0.,-1.));
#26112=DIRECTION('',(-0.054058861725389,-0.998537750647894,0.));
#26113=DIRECTION('center_axis',(0.,0.,-1.));
#26114=DIRECTION('ref_axis',(-1.,0.,0.));
#26115=DIRECTION('center_axis',(0.,0.,-1.));
#26116=DIRECTION('ref_axis',(1.,0.,0.));
#26117=DIRECTION('center_axis',(-0.546085222877805,0.837729627836152,0.));
#26118=DIRECTION('ref_axis',(0.837729627836152,0.546085222877805,0.));
#26119=DIRECTION('',(0.,0.,1.));
#26120=DIRECTION('',(0.837729627836152,0.546085222877805,0.));
#26121=DIRECTION('',(0.,0.,-1.));
#26122=DIRECTION('',(0.837729627836152,0.546085222877805,0.));
#26123=DIRECTION('center_axis',(0.,0.,1.));
#26124=DIRECTION('ref_axis',(1.,0.,0.));
#26125=DIRECTION('center_axis',(0.,0.,1.));
#26126=DIRECTION('ref_axis',(1.,0.,0.));
#26127=DIRECTION('',(0.356756665108425,-0.934197346335727,0.));
#26128=DIRECTION('center_axis',(0.934197346335727,0.356756665108425,0.));
#26129=DIRECTION('ref_axis',(0.356756665108425,-0.934197346335727,0.));
#26130=DIRECTION('',(0.,0.,-1.));
#26131=DIRECTION('',(0.356756665108425,-0.934197346335727,0.));
#26132=DIRECTION('center_axis',(0.,0.,-1.));
#26133=DIRECTION('ref_axis',(-1.,0.,0.));
#26134=DIRECTION('center_axis',(0.,0.,-1.));
#26135=DIRECTION('ref_axis',(1.,0.,0.));
#26136=DIRECTION('center_axis',(-0.839609011476982,0.543191225855725,0.));
#26137=DIRECTION('ref_axis',(0.543191225855725,0.839609011476982,0.));
#26138=DIRECTION('',(0.,0.,1.));
#26139=DIRECTION('',(0.543191225855725,0.839609011476982,0.));
#26140=DIRECTION('',(0.,0.,-1.));
#26141=DIRECTION('',(0.543191225855725,0.839609011476982,0.));
#26142=DIRECTION('center_axis',(0.,0.,1.));
#26143=DIRECTION('ref_axis',(1.,0.,0.));
#26144=DIRECTION('center_axis',(0.,0.,1.));
#26145=DIRECTION('ref_axis',(1.,0.,0.));
#26146=DIRECTION('',(0.705885723512444,-0.708325733925652,0.));
#26147=DIRECTION('center_axis',(0.708325733925652,0.705885723512444,0.));
#26148=DIRECTION('ref_axis',(0.705885723512444,-0.708325733925652,0.));
#26149=DIRECTION('',(0.,0.,-1.));
#26150=DIRECTION('',(0.705885723512444,-0.708325733925652,0.));
#26151=DIRECTION('center_axis',(0.,0.,-1.));
#26152=DIRECTION('ref_axis',(-1.,0.,0.));
#26153=DIRECTION('center_axis',(0.,0.,-1.));
#26154=DIRECTION('ref_axis',(1.,0.,0.));
#26155=DIRECTION('center_axis',(-0.987956774383376,0.154730126187482,0.));
#26156=DIRECTION('ref_axis',(0.154730126187482,0.987956774383376,0.));
#26157=DIRECTION('',(0.,0.,1.));
#26158=DIRECTION('',(0.154730126187482,0.987956774383376,0.));
#26159=DIRECTION('',(0.,0.,-1.));
#26160=DIRECTION('',(0.154730126187482,0.987956774383376,0.));
#26161=DIRECTION('center_axis',(0.,0.,1.));
#26162=DIRECTION('ref_axis',(1.,0.,0.));
#26163=DIRECTION('center_axis',(0.,0.,1.));
#26164=DIRECTION('ref_axis',(1.,0.,0.));
#26165=DIRECTION('',(0.932960727550677,-0.359978167182556,0.));
#26166=DIRECTION('center_axis',(0.359978167182556,0.932960727550677,0.));
#26167=DIRECTION('ref_axis',(0.932960727550677,-0.359978167182556,0.));
#26168=DIRECTION('',(0.,0.,-1.));
#26169=DIRECTION('',(0.932960727550677,-0.359978167182556,0.));
#26170=DIRECTION('center_axis',(0.,0.,-1.));
#26171=DIRECTION('ref_axis',(-1.,0.,0.));
#26172=DIRECTION('center_axis',(0.,0.,-1.));
#26173=DIRECTION('ref_axis',(1.,0.,0.));
#26174=DIRECTION('center_axis',(-0.965477835693361,-0.260485217977651,0.));
#26175=DIRECTION('ref_axis',(-0.260485217977651,0.965477835693361,0.));
#26176=DIRECTION('',(0.,0.,1.));
#26177=DIRECTION('',(-0.260485217977651,0.965477835693361,0.));
#26178=DIRECTION('',(0.,0.,-1.));
#26179=DIRECTION('',(-0.260485217977651,0.965477835693361,0.));
#26180=DIRECTION('center_axis',(0.,0.,1.));
#26181=DIRECTION('ref_axis',(1.,0.,0.));
#26182=DIRECTION('center_axis',(0.,0.,1.));
#26183=DIRECTION('ref_axis',(1.,0.,0.));
#26184=DIRECTION('',(0.998718346113269,0.0506128949653851,0.));
#26185=DIRECTION('center_axis',(-0.0506128949653851,0.998718346113269,0.));
#26186=DIRECTION('ref_axis',(0.998718346113269,0.0506128949653851,0.));
#26187=DIRECTION('',(0.,0.,-1.));
#26188=DIRECTION('',(0.998718346113269,0.0506128949653851,0.));
#26189=DIRECTION('center_axis',(0.,0.,-1.));
#26190=DIRECTION('ref_axis',(-1.,0.,0.));
#26191=DIRECTION('center_axis',(0.,0.,-1.));
#26192=DIRECTION('ref_axis',(1.,0.,0.));
#26193=DIRECTION('center_axis',(-0.776059008121178,-0.630660301520536,0.));
#26194=DIRECTION('ref_axis',(-0.630660301520536,0.776059008121178,0.));
#26195=DIRECTION('',(0.,0.,1.));
#26196=DIRECTION('',(-0.630660301520536,0.776059008121178,0.));
#26197=DIRECTION('',(0.,0.,-1.));
#26198=DIRECTION('',(-0.630660301520536,0.776059008121178,0.));
#26199=DIRECTION('center_axis',(0.,0.,1.));
#26200=DIRECTION('ref_axis',(1.,0.,0.));
#26201=DIRECTION('center_axis',(0.,0.,1.));
#26202=DIRECTION('ref_axis',(1.,0.,0.));
#26203=DIRECTION('',(0.891788489561539,0.452452527770095,0.));
#26204=DIRECTION('center_axis',(-0.452452527770095,0.891788489561539,0.));
#26205=DIRECTION('ref_axis',(0.891788489561539,0.452452527770095,0.));
#26206=DIRECTION('',(0.,0.,-1.));
#26207=DIRECTION('',(0.891788489561539,0.452452527770095,0.));
#26208=DIRECTION('center_axis',(0.,0.,-1.));
#26209=DIRECTION('ref_axis',(-1.,0.,0.));
#26210=DIRECTION('center_axis',(0.,0.,-1.));
#26211=DIRECTION('ref_axis',(1.,0.,0.));
#26212=DIRECTION('center_axis',(0.,0.,1.));
#26213=DIRECTION('ref_axis',(1.,0.,0.));
#26214=DIRECTION('center_axis',(0.,0.,-1.));
#26215=DIRECTION('ref_axis',(1.,0.,0.));
#26216=DIRECTION('',(-0.866025403784439,-1.06057523872491E-16,0.5));
#26217=DIRECTION('center_axis',(0.5,-0.866025403784439,0.));
#26218=DIRECTION('ref_axis',(0.866025403784439,0.5,0.));
#26219=DIRECTION('',(0.,0.,1.));
#26220=DIRECTION('',(0.,0.,1.));
#26221=DIRECTION('center_axis',(1.,-3.49629579342466E-16,0.));
#26222=DIRECTION('ref_axis',(3.49629579342466E-16,1.,0.));
#26223=DIRECTION('',(0.,0.,1.));
#26224=DIRECTION('center_axis',(0.5,0.866025403784439,0.));
#26225=DIRECTION('ref_axis',(-0.866025403784439,0.5,0.));
#26226=DIRECTION('',(0.,0.,1.));
#26227=DIRECTION('center_axis',(0.,0.,-1.));
#26228=DIRECTION('ref_axis',(1.,0.,0.));
#26229=DIRECTION('',(0.866025403784439,1.06057523872491E-16,0.5));
#26230=DIRECTION('center_axis',(0.,0.,1.));
#26231=DIRECTION('ref_axis',(1.,0.,0.));
#26232=DIRECTION('center_axis',(-0.5,0.866025403784439,0.));
#26233=DIRECTION('ref_axis',(-0.866025403784439,-0.5,0.));
#26234=DIRECTION('',(0.,0.,1.));
#26235=DIRECTION('center_axis',(0.,0.,1.));
#26236=DIRECTION('ref_axis',(1.,0.,0.));
#26237=DIRECTION('center_axis',(0.,0.,1.));
#26238=DIRECTION('ref_axis',(1.,0.,0.));
#26239=DIRECTION('center_axis',(0.,0.,1.));
#26240=DIRECTION('ref_axis',(1.,0.,0.));
#26241=DIRECTION('center_axis',(0.,0.,-1.));
#26242=DIRECTION('ref_axis',(1.,0.,0.));
#26243=DIRECTION('center_axis',(-0.5,-0.866025403784439,0.));
#26244=DIRECTION('ref_axis',(0.866025403784439,-0.5,0.));
#26245=DIRECTION('',(0.,0.,1.));
#26246=DIRECTION('center_axis',(-1.,0.,0.));
#26247=DIRECTION('ref_axis',(0.,-1.,0.));
#26248=DIRECTION('center_axis',(0.,0.,1.));
#26249=DIRECTION('ref_axis',(1.,0.,0.));
#26250=DIRECTION('center_axis',(0.,0.,1.));
#26251=DIRECTION('ref_axis',(1.,0.,0.));
#26252=DIRECTION('',(0.,0.,1.));
#26253=DIRECTION('center_axis',(0.,0.,1.));
#26254=DIRECTION('ref_axis',(1.,0.,0.));
#26255=DIRECTION('center_axis',(0.,0.,-1.));
#26256=DIRECTION('ref_axis',(1.,0.,0.));
#26257=DIRECTION('',(0.832050294337844,1.01896772969045E-16,0.554700196225229));
#26258=DIRECTION('center_axis',(0.,0.,-1.));
#26259=DIRECTION('ref_axis',(-1.,0.,0.));
#26260=DIRECTION('center_axis',(0.,0.,1.));
#26261=DIRECTION('ref_axis',(1.,0.,0.));
#26262=DIRECTION('center_axis',(0.,0.,1.));
#26263=DIRECTION('ref_axis',(1.,0.,0.));
#26264=DIRECTION('',(0.707106781186547,8.65956056235493E-17,-0.707106781186548));
#26265=DIRECTION('center_axis',(0.,0.,1.));
#26266=DIRECTION('ref_axis',(1.,0.,0.));
#26267=DIRECTION('center_axis',(0.,0.,1.));
#26268=DIRECTION('ref_axis',(1.,0.,0.));
#26269=DIRECTION('center_axis',(0.,0.,1.));
#26270=DIRECTION('ref_axis',(1.,0.,0.));
#26271=DIRECTION('',(0.,0.,-1.));
#26272=DIRECTION('center_axis',(0.,0.,1.));
#26273=DIRECTION('ref_axis',(1.,0.,0.));
#26274=DIRECTION('center_axis',(0.,0.,1.));
#26275=DIRECTION('ref_axis',(1.,0.,0.));
#26276=DIRECTION('center_axis',(0.,0.,1.));
#26277=DIRECTION('ref_axis',(1.,0.,0.));
#26278=DIRECTION('center_axis',(0.,0.,1.));
#26279=DIRECTION('ref_axis',(1.,0.,0.));
#26280=DIRECTION('center_axis',(0.,0.,1.));
#26281=DIRECTION('ref_axis',(1.,0.,0.));
#26282=DIRECTION('center_axis',(0.,0.,1.));
#26283=DIRECTION('ref_axis',(1.,0.,0.));
#26284=DIRECTION('center_axis',(0.,0.,1.));
#26285=DIRECTION('ref_axis',(1.,0.,0.));
#26286=DIRECTION('center_axis',(0.,0.,1.));
#26287=DIRECTION('ref_axis',(1.,0.,0.));
#26288=DIRECTION('center_axis',(0.,0.,1.));
#26289=DIRECTION('ref_axis',(1.,0.,0.));
#26290=DIRECTION('center_axis',(0.,0.,1.));
#26291=DIRECTION('ref_axis',(1.,0.,0.));
#26292=DIRECTION('center_axis',(0.,0.,1.));
#26293=DIRECTION('ref_axis',(1.,0.,0.));
#26294=DIRECTION('center_axis',(0.,0.,1.));
#26295=DIRECTION('ref_axis',(1.,0.,0.));
#26296=DIRECTION('center_axis',(0.,0.,1.));
#26297=DIRECTION('ref_axis',(1.,0.,0.));
#26298=DIRECTION('center_axis',(0.,0.,1.));
#26299=DIRECTION('ref_axis',(1.,0.,0.));
#26300=DIRECTION('',(0.,0.,-1.));
#26301=DIRECTION('center_axis',(0.,0.,1.));
#26302=DIRECTION('ref_axis',(1.,0.,0.));
#26303=DIRECTION('center_axis',(0.,0.,1.));
#26304=DIRECTION('ref_axis',(1.,0.,0.));
#26305=DIRECTION('center_axis',(0.,0.,1.));
#26306=DIRECTION('ref_axis',(1.,0.,0.));
#26307=DIRECTION('center_axis',(0.,0.,1.));
#26308=DIRECTION('ref_axis',(1.,0.,0.));
#26309=DIRECTION('center_axis',(0.,0.,1.));
#26310=DIRECTION('ref_axis',(1.,0.,0.));
#26311=DIRECTION('center_axis',(0.,0.,1.));
#26312=DIRECTION('ref_axis',(1.,0.,0.));
#26313=DIRECTION('center_axis',(0.,0.,1.));
#26314=DIRECTION('ref_axis',(1.,0.,0.));
#26315=DIRECTION('center_axis',(0.,0.,1.));
#26316=DIRECTION('ref_axis',(1.,0.,0.));
#26317=DIRECTION('center_axis',(0.,0.,1.));
#26318=DIRECTION('ref_axis',(1.,0.,0.));
#26319=DIRECTION('center_axis',(0.,0.,1.));
#26320=DIRECTION('ref_axis',(1.,0.,0.));
#26321=DIRECTION('center_axis',(0.,0.,1.));
#26322=DIRECTION('ref_axis',(1.,0.,0.));
#26323=DIRECTION('center_axis',(0.,0.,1.));
#26324=DIRECTION('ref_axis',(1.,0.,0.));
#26325=DIRECTION('center_axis',(0.,0.,1.));
#26326=DIRECTION('ref_axis',(1.,0.,0.));
#26327=DIRECTION('center_axis',(0.,0.,1.));
#26328=DIRECTION('ref_axis',(1.,0.,0.));
#26329=DIRECTION('center_axis',(0.,0.,1.));
#26330=DIRECTION('ref_axis',(1.,0.,0.));
#26331=DIRECTION('center_axis',(0.,0.,1.));
#26332=DIRECTION('ref_axis',(1.,0.,0.));
#26333=DIRECTION('center_axis',(0.,0.,1.));
#26334=DIRECTION('ref_axis',(1.,0.,0.));
#26335=DIRECTION('center_axis',(0.,0.,-1.));
#26336=DIRECTION('ref_axis',(1.,0.,0.));
#26337=DIRECTION('center_axis',(0.,0.,1.));
#26338=DIRECTION('ref_axis',(1.,0.,0.));
#26339=DIRECTION('',(-0.707106781186547,-8.65956056235492E-17,-0.707106781186548));
#26340=DIRECTION('center_axis',(0.,0.,1.));
#26341=DIRECTION('ref_axis',(1.,0.,0.));
#32296=CARTESIAN_POINT('',(0.,0.,0.));
#32297=CARTESIAN_POINT('Origin',(0.,0.,-1.33003901172249));
#32298=CARTESIAN_POINT('',(-0.747455179358203,1.21560254491701E-5,-0.193723222248808));
#32299=CARTESIAN_POINT('',(-0.747444078220075,-6.40459137760119E-6,-0.187197830382768));
#32300=CARTESIAN_POINT('',(-0.7475,-1.95907305151415E-14,-1.33003901172249));
#32301=CARTESIAN_POINT('',(0.708694801171174,0.237542783106662,-0.12));
#32302=CARTESIAN_POINT('Ctrl Pts',(-0.747455179358203,1.21560254491664E-5,
-0.193723222248808));
#32303=CARTESIAN_POINT('Ctrl Pts',(-0.747409043365027,-0.0764700511820524,
-0.191546603424787));
#32304=CARTESIAN_POINT('Ctrl Pts',(-0.717056524628233,-0.275197846725069,
-0.185891997066606));
#32305=CARTESIAN_POINT('Ctrl Pts',(-0.543630981761309,-0.556730447339977,
-0.176759403174265));
#32306=CARTESIAN_POINT('Ctrl Pts',(-0.217353554555294,-0.747156946739445,
-0.166325440571784));
#32307=CARTESIAN_POINT('Ctrl Pts',(0.160155550638919,-0.761465819139253,
-0.155891477969304));
#32308=CARTESIAN_POINT('Ctrl Pts',(0.499915663487151,-0.59630128045638,
-0.145457515366823));
#32309=CARTESIAN_POINT('Ctrl Pts',(0.721838643854921,-0.290560778341041,
-0.135023552764343));
#32310=CARTESIAN_POINT('Ctrl Pts',(0.763953513632068,0.0137597889773607,
-0.126537714308735));
#32311=CARTESIAN_POINT('Ctrl Pts',(0.725795582116324,0.186572354342476,
-0.121529863387287));
#32312=CARTESIAN_POINT('Ctrl Pts',(0.708694801171174,0.237542783106662,
-0.12));
#32313=CARTESIAN_POINT('',(0.747395528060274,0.0124969850565471,-0.12));
#32314=CARTESIAN_POINT('Origin',(0.,0.,-0.12));
#32315=CARTESIAN_POINT('Ctrl Pts',(-0.747444078220075,-6.40459137765323E-6,
-0.187197830382768));
#32316=CARTESIAN_POINT('Ctrl Pts',(-0.747460394071194,-0.0538175344429383,
-0.185666478793473));
#32317=CARTESIAN_POINT('Ctrl Pts',(-0.728699568742349,-0.229832596850158,
-0.180657139670018));
#32318=CARTESIAN_POINT('Ctrl Pts',(-0.591963456523644,-0.505033918677001,
-0.172169813012403));
#32319=CARTESIAN_POINT('Ctrl Pts',(-0.284343786563683,-0.724320025643106,
-0.161735850409922));
#32320=CARTESIAN_POINT('Ctrl Pts',(0.09031673140191,-0.772864465068915,
-0.151301887807442));
#32321=CARTESIAN_POINT('Ctrl Pts',(0.44365235923649,-0.639262442637623,
-0.140867925204961));
#32322=CARTESIAN_POINT('Ctrl Pts',(0.692489824641788,-0.354929918130683,
-0.13043396260248));
#32323=CARTESIAN_POINT('Ctrl Pts',(0.749438361810141,-0.109676867461678,
-0.12347798753416));
#32324=CARTESIAN_POINT('Ctrl Pts',(0.747395528060274,0.012496985056547,
-0.12));
#32325=CARTESIAN_POINT('Origin',(0.,0.,-1.33003901172249));
#32326=CARTESIAN_POINT('',(-0.747444051384665,-6.42748184059897E-6,-0.327407432775125));
#32327=CARTESIAN_POINT('',(-0.747492032740272,-1.77696257388504E-5,-0.320882040909084));
#32328=CARTESIAN_POINT('',(-0.7475,-1.95907305151415E-14,-1.33003901172249));
#32329=CARTESIAN_POINT('Ctrl Pts',(-0.747444051384665,-6.42748184055686E-6,
-0.327407432775125));
#32330=CARTESIAN_POINT('Ctrl Pts',(-0.747460735268479,-0.0535655898421367,
-0.325883248386414));
#32331=CARTESIAN_POINT('Ctrl Pts',(-0.728815731862446,-0.229328242581168,
-0.320881076463544));
#32332=CARTESIAN_POINT('Ctrl Pts',(-0.592475727944849,-0.504436944883207,
-0.312400917006513));
#32333=CARTESIAN_POINT('Ctrl Pts',(-0.285071300054314,-0.724029331642755,
-0.301966954404032));
#32334=CARTESIAN_POINT('Ctrl Pts',(0.0895271131383019,-0.772961199617318,
-0.291532991801552));
#32335=CARTESIAN_POINT('Ctrl Pts',(0.443023143994601,-0.639698844990308,
-0.281099029199071));
#32336=CARTESIAN_POINT('Ctrl Pts',(0.692094455558156,-0.355653462496774,
-0.27066506659659));
#32337=CARTESIAN_POINT('Ctrl Pts',(0.778032597283115,0.0122227909580681,
-0.26023110399411));
#32338=CARTESIAN_POINT('Ctrl Pts',(0.680581143349384,0.377218004776158,
-0.249797141391629));
#32339=CARTESIAN_POINT('Ctrl Pts',(0.422710313521399,0.653299414263413,
-0.239363178789149));
#32340=CARTESIAN_POINT('Ctrl Pts',(0.0652026943778876,0.775391960536891,
-0.228929216186668));
#32341=CARTESIAN_POINT('Ctrl Pts',(-0.307673823063876,0.714717431064052,
-0.218495253584187));
#32342=CARTESIAN_POINT('Ctrl Pts',(-0.608028707877235,0.485577090895019,
-0.208061290981707));
#32343=CARTESIAN_POINT('Ctrl Pts',(-0.732306246915869,0.213659075752679,
-0.199803947203247));
#32344=CARTESIAN_POINT('Ctrl Pts',(-0.747482763396927,0.0457397543737755,
-0.195024590958948));
#32345=CARTESIAN_POINT('Ctrl Pts',(-0.747455179358203,1.21560254491664E-5,
-0.193723222248808));
#32346=CARTESIAN_POINT('Ctrl Pts',(-0.747492032740272,-1.77696257388088E-5,
-0.320882040909084));
#32347=CARTESIAN_POINT('Ctrl Pts',(-0.747521461794713,-0.0308968347335437,
-0.3200031237551));
#32348=CARTESIAN_POINT('Ctrl Pts',(-0.738208053524619,-0.183950674319053,
-0.315646219066956));
#32349=CARTESIAN_POINT('Ctrl Pts',(-0.635857117988058,-0.448519615362849,
-0.307811326844651));
#32350=CARTESIAN_POINT('Ctrl Pts',(-0.349675784487423,-0.695133774103561,
-0.29737736424217));
#32351=CARTESIAN_POINT('Ctrl Pts',(0.0189274157531888,-0.777898369643474,
-0.28694340163969));
#32352=CARTESIAN_POINT('Ctrl Pts',(0.383069251609914,-0.67730500314506,
-0.276509439037209));
#32353=CARTESIAN_POINT('Ctrl Pts',(0.656918053157321,-0.417064487823481,
-0.266075476434728));
#32354=CARTESIAN_POINT('Ctrl Pts',(0.775925115315038,-0.0585179376441977,
-0.255641513832248));
#32355=CARTESIAN_POINT('Ctrl Pts',(0.712039292365909,0.313821812003488,
-0.245207551229767));
#32356=CARTESIAN_POINT('Ctrl Pts',(0.480319196218496,0.612190866640263,
-0.234773588627287));
#32357=CARTESIAN_POINT('Ctrl Pts',(0.135383189993241,0.766260668703223,
-0.224339626024806));
#32358=CARTESIAN_POINT('Ctrl Pts',(-0.241463591288354,0.739715845333339,
-0.213905663422325));
#32359=CARTESIAN_POINT('Ctrl Pts',(-0.561395755032469,0.5388126158932,-0.203471700819845));
#32360=CARTESIAN_POINT('Ctrl Pts',(-0.721466439761005,0.25903244063098,
-0.194569089806659));
#32361=CARTESIAN_POINT('Ctrl Pts',(-0.747423337703997,0.0683976642946542,
-0.189144466327633));
#32362=CARTESIAN_POINT('Ctrl Pts',(-0.747444078220075,-6.40459137765323E-6,
-0.187197830382768));
#32363=CARTESIAN_POINT('Origin',(0.,0.,-1.33003901172249));
#32364=CARTESIAN_POINT('',(-0.747492771866375,-1.77854026472873E-5,-0.46109164330144));
#32365=CARTESIAN_POINT('',(-0.747552914013562,-7.59237280062441E-6,-0.4545662514354));
#32366=CARTESIAN_POINT('',(-0.7475,-1.95907305151415E-14,-1.33003901172249));
#32367=CARTESIAN_POINT('Ctrl Pts',(-0.747492771866375,-1.77854026472586E-5,
-0.46109164330144));
#32368=CARTESIAN_POINT('Ctrl Pts',(-0.747522042549813,-0.0306449575355944,
-0.460219893348041));
#32369=CARTESIAN_POINT('Ctrl Pts',(-0.738300189612618,-0.18344667931334,
-0.455870155860481));
#32370=CARTESIAN_POINT('Ctrl Pts',(-0.636310057828871,-0.44787680201301,
-0.448042430838761));
#32371=CARTESIAN_POINT('Ctrl Pts',(-0.350378094607072,-0.694780044542982,
-0.43760846823628));
#32372=CARTESIAN_POINT('Ctrl Pts',(0.0181412792138254,-0.777917099351843,
-0.4271745056338));
#32373=CARTESIAN_POINT('Ctrl Pts',(0.382384582988461,-0.677691781098534,
-0.416740543031318));
#32374=CARTESIAN_POINT('Ctrl Pts',(0.656496245978095,-0.417728139454399,
-0.406306580428839));
#32375=CARTESIAN_POINT('Ctrl Pts',(0.775865572452267,-0.0593020485231105,
-0.395872617826357));
#32376=CARTESIAN_POINT('Ctrl Pts',(0.71235609003925,0.313102092711011,-0.385438655223877));
#32377=CARTESIAN_POINT('Ctrl Pts',(0.480937580760022,0.611705127399056,
-0.375004692621396));
#32378=CARTESIAN_POINT('Ctrl Pts',(0.136157562681014,0.766123513283346,
-0.364570730018916));
#32379=CARTESIAN_POINT('Ctrl Pts',(-0.240716072858233,0.739959385191357,
-0.354136767416435));
#32380=CARTESIAN_POINT('Ctrl Pts',(-0.560850667196364,0.539379874112098,
-0.343702804813955));
#32381=CARTESIAN_POINT('Ctrl Pts',(-0.721333836132674,0.259535992032654,
-0.334793026600185));
#32382=CARTESIAN_POINT('Ctrl Pts',(-0.747422664848419,0.0686493471490407,
-0.329361235920574));
#32383=CARTESIAN_POINT('Ctrl Pts',(-0.747444051384665,-6.42748184055686E-6,
-0.327407432775125));
#32384=CARTESIAN_POINT('Ctrl Pts',(-0.747552914013562,-7.5923728006114E-6,
-0.4545662514354));
#32385=CARTESIAN_POINT('Ctrl Pts',(-0.747557174200553,-0.00796275413960644,
-0.454339768716726));
#32386=CARTESIAN_POINT('Ctrl Pts',(-0.745521898301695,-0.138079373049215,
-0.450635298463892));
#32387=CARTESIAN_POINT('Ctrl Pts',(-0.674371225051026,-0.388210728933218,
-0.443452840676899));
#32388=CARTESIAN_POINT('Ctrl Pts',(-0.412054943730941,-0.660071846530996,
-0.433018878074418));
#32389=CARTESIAN_POINT('Ctrl Pts',(-0.0526134386847218,-0.776347824950465,
-0.422584915471937));
#32390=CARTESIAN_POINT('Ctrl Pts',(0.319229548446936,-0.709631323036316,
-0.412150952869456));
#32391=CARTESIAN_POINT('Ctrl Pts',(0.615827130120359,-0.475648047450979,
-0.401716990266976));
#32392=CARTESIAN_POINT('Ctrl Pts',(0.767268468189365,-0.129550055793601,
-0.391283027664495));
#32393=CARTESIAN_POINT('Ctrl Pts',(0.737857415668762,0.24708410184319,-0.380849065062015));
#32394=CARTESIAN_POINT('Ctrl Pts',(0.534526434095284,0.565478213973463,
-0.370415102459534));
#32395=CARTESIAN_POINT('Ctrl Pts',(0.205202547258304,0.750583795355781,
-0.359981139857054));
#32396=CARTESIAN_POINT('Ctrl Pts',(-0.172489509004567,0.758769720339229,
-0.349547177254573));
#32397=CARTESIAN_POINT('Ctrl Pts',(-0.509524166428113,0.588106489551379,
-0.339113214652093));
#32398=CARTESIAN_POINT('Ctrl Pts',(-0.708185410677574,0.304874056256314,
-0.329558169203596));
#32399=CARTESIAN_POINT('Ctrl Pts',(-0.747405007264242,0.0912955733047001,
-0.32348111128926));
#32400=CARTESIAN_POINT('Ctrl Pts',(-0.747492032740272,-1.77696257388088E-5,
-0.320882040909084));
#32401=CARTESIAN_POINT('Origin',(0.,0.,-1.33003901172249));
#32402=CARTESIAN_POINT('',(-0.747553321122146,-7.36938304350496E-6,-0.594775853827756));
#32403=CARTESIAN_POINT('',(-0.747538056636856,1.3017034258378E-5,-0.588250461961716));
#32404=CARTESIAN_POINT('',(-0.7475,-1.95907305151415E-14,-1.33003901172249));
#32405=CARTESIAN_POINT('Ctrl Pts',(-0.747553321122146,-7.36938304344778E-6,
-0.594775853827756));
#32406=CARTESIAN_POINT('Ctrl Pts',(-0.747557343204729,-0.00771077241775835,
-0.594556538309667));
#32407=CARTESIAN_POINT('Ctrl Pts',(-0.745590310689939,-0.137575565048739,
-0.590859235257418));
#32408=CARTESIAN_POINT('Ctrl Pts',(-0.674763198638613,-0.387529025027261,
-0.583683944671008));
#32409=CARTESIAN_POINT('Ctrl Pts',(-0.412721788492088,-0.659655095318368,
-0.573249982068528));
#32410=CARTESIAN_POINT('Ctrl Pts',(-0.0533979730410232,-0.776294258609905,
-0.562816019466047));
#32411=CARTESIAN_POINT('Ctrl Pts',(0.318512246619028,-0.709953567657274,
-0.552382056863567));
#32412=CARTESIAN_POINT('Ctrl Pts',(0.615346135603009,-0.476270146948173,
-0.541948094261086));
#32413=CARTESIAN_POINT('Ctrl Pts',(0.767137155915032,-0.130325375465362,
-0.531514131658606));
#32414=CARTESIAN_POINT('Ctrl Pts',(0.738106737168653,0.246338312127524,
-0.521080169056125));
#32415=CARTESIAN_POINT('Ctrl Pts',(0.535097621960438,0.56493774386907,-0.510646206453644));
#32416=CARTESIAN_POINT('Ctrl Pts',(0.20596096711532,0.750376038730258,-0.500212243851164));
#32417=CARTESIAN_POINT('Ctrl Pts',(-0.171722623797873,0.758943647414989,
-0.489778281248683));
#32418=CARTESIAN_POINT('Ctrl Pts',(-0.50892957801762,0.588621104017174,
-0.479344318646202));
#32419=CARTESIAN_POINT('Ctrl Pts',(-0.708026179252433,0.305377277568616,
-0.469782105997122));
#32420=CARTESIAN_POINT('Ctrl Pts',(-0.747405262420699,0.0915471027789014,
-0.463697880882201));
#32421=CARTESIAN_POINT('Ctrl Pts',(-0.747492771866375,-1.77854026472586E-5,
-0.46109164330144));
#32422=CARTESIAN_POINT('Ctrl Pts',(-0.747538056636856,1.30170342583693E-5,
-0.588250461961716));
#32423=CARTESIAN_POINT('Ctrl Pts',(-0.747449782311829,-0.107195335869156,
-0.585198426144193));
#32424=CARTESIAN_POINT('Ctrl Pts',(-0.697538394050389,-0.33665395487388,
-0.578668402792509));
#32425=CARTESIAN_POINT('Ctrl Pts',(-0.470949408769067,-0.619427779176751,
-0.568660391906665));
#32426=CARTESIAN_POINT('Ctrl Pts',(-0.123709349589919,-0.768231811408391,
-0.558226429304186));
#32427=CARTESIAN_POINT('Ctrl Pts',(0.252690166207058,-0.735956383991622,
-0.547792466701704));
#32428=CARTESIAN_POINT('Ctrl Pts',(0.569528234436075,-0.530209118571064,
-0.537358504099224));
#32429=CARTESIAN_POINT('Ctrl Pts',(0.752123144005562,-0.199486579716444,
-0.526924541496743));
#32430=CARTESIAN_POINT('Ctrl Pts',(0.757435558261682,0.178256821234392,
-0.516490578894262));
#32431=CARTESIAN_POINT('Ctrl Pts',(0.58421329122536,0.513983413731816,-0.506056616291782));
#32432=CARTESIAN_POINT('Ctrl Pts',(0.273286459598611,0.728559283954182,
-0.495622653689301));
#32433=CARTESIAN_POINT('Ctrl Pts',(-0.102056559562226,0.77140688218741,
-0.485188691086821));
#32434=CARTESIAN_POINT('Ctrl Pts',(-0.453343888260034,0.63242662674262,
-0.47475472848434));
#32435=CARTESIAN_POINT('Ctrl Pts',(-0.692468131949325,0.350629951601099,
-0.464547248600534));
#32436=CARTESIAN_POINT('Ctrl Pts',(-0.74749175253247,0.114200886509031,
-0.457817756250887));
#32437=CARTESIAN_POINT('Ctrl Pts',(-0.747552914013562,-7.5923728006114E-6,
-0.4545662514354));
#32438=CARTESIAN_POINT('Origin',(0.,0.,-1.33003901172249));
#32439=CARTESIAN_POINT('',(-0.747537418840408,1.31793815494462E-5,-0.728460064354072));
#32440=CARTESIAN_POINT('',(-0.747472643624562,1.62103417218756E-5,-0.721934672488032));
#32441=CARTESIAN_POINT('',(-0.7475,-1.95907305151415E-14,-1.33003901172249));
#32442=CARTESIAN_POINT('Ctrl Pts',(-0.747537418840408,1.31793815494417E-5,
-0.728460064354072));
#32443=CARTESIAN_POINT('Ctrl Pts',(-0.747448558105652,-0.106943676944281,
-0.725415195737133));
#32444=CARTESIAN_POINT('Ctrl Pts',(-0.697716187447847,-0.336151536347626,
-0.718892339586034));
#32445=CARTESIAN_POINT('Ctrl Pts',(-0.471575149406303,-0.618951531170265,
-0.708891495900776));
#32446=CARTESIAN_POINT('Ctrl Pts',(-0.124485645778937,-0.768106401138927,
-0.698457533298295));
#32447=CARTESIAN_POINT('Ctrl Pts',(0.251946294775516,-0.736211371838605,
-0.688023570695814));
#32448=CARTESIAN_POINT('Ctrl Pts',(0.568992125251126,-0.530784401501965,
-0.677589608093334));
#32449=CARTESIAN_POINT('Ctrl Pts',(0.751921163041749,-0.200246558136555,
-0.667155645490853));
#32450=CARTESIAN_POINT('Ctrl Pts',(0.757615314330881,0.177491281382809,
-0.656721682888373));
#32451=CARTESIAN_POINT('Ctrl Pts',(0.584732414132281,0.513392757388168,
-0.646287720285892));
#32452=CARTESIAN_POINT('Ctrl Pts',(0.274022587194125,0.728282734371089,
-0.635853757683411));
#32453=CARTESIAN_POINT('Ctrl Pts',(-0.101276939472296,0.771509624701284,
-0.625419795080931));
#32454=CARTESIAN_POINT('Ctrl Pts',(-0.452704539459628,0.632884443977129,
-0.61498583247845));
#32455=CARTESIAN_POINT('Ctrl Pts',(-0.692281540434249,0.351131872468854,
-0.604771185394059));
#32456=CARTESIAN_POINT('Ctrl Pts',(-0.747493559514422,0.114452674833002,
-0.598034525843827));
#32457=CARTESIAN_POINT('Ctrl Pts',(-0.747553321122146,-7.36938304344778E-6,
-0.594775853827756));
#32458=CARTESIAN_POINT('Ctrl Pts',(-0.747472643624562,1.6210341721886E-5,
-0.721934672488032));
#32459=CARTESIAN_POINT('Ctrl Pts',(-0.747402612221546,-0.0842954619945286,
-0.719535071105819));
#32460=CARTESIAN_POINT('Ctrl Pts',(-0.712499566770547,-0.290865199736191,
-0.713657482189446));
#32461=CARTESIAN_POINT('Ctrl Pts',(-0.525861117638763,-0.573545293931951,
-0.704301905738913));
#32462=CARTESIAN_POINT('Ctrl Pts',(-0.193759067069451,-0.753618964174968,
-0.693867943136433));
#32463=CARTESIAN_POINT('Ctrl Pts',(0.184013817024176,-0.756057560229359,
-0.683433980533952));
#32464=CARTESIAN_POINT('Ctrl Pts',(0.518412914638575,-0.580286282081279,
-0.673000017931472));
#32465=CARTESIAN_POINT('Ctrl Pts',(0.73061721497504,-0.267736072313561,
-0.66256605532899));
#32466=CARTESIAN_POINT('Ctrl Pts',(0.770608169635336,0.107922046529211,
-0.652132092726511));
#32467=CARTESIAN_POINT('Ctrl Pts',(0.62895953467438,0.458141924492798,-0.64169813012403));
#32468=CARTESIAN_POINT('Ctrl Pts',(0.339059224908714,0.700373444128258,
-0.63126416752155));
#32469=CARTESIAN_POINT('Ctrl Pts',(-0.0307605314660666,0.777520359180197,
-0.620830204919068));
#32470=CARTESIAN_POINT('Ctrl Pts',(-0.393329741412471,0.671398416557692,
-0.610396242316588));
#32471=CARTESIAN_POINT('Ctrl Pts',(-0.663187433844332,0.407021555727391,
-0.599962279714107));
#32472=CARTESIAN_POINT('Ctrl Pts',(-0.74351458894893,0.152101734785081,
-0.59258035292915));
#32473=CARTESIAN_POINT('Ctrl Pts',(-0.747550376479259,0.0149753519108121,
-0.588676413678353));
#32474=CARTESIAN_POINT('Ctrl Pts',(-0.747538056636856,1.30170342583693E-5,
-0.588250461961716));
#32475=CARTESIAN_POINT('Origin',(0.,0.,-1.33003901172249));
#32476=CARTESIAN_POINT('',(-0.747472002174668,1.61159471936433E-5,-0.862144274880388));
#32477=CARTESIAN_POINT('',(-0.747440403350747,2.49991181699993E-7,-0.855618883014348));
#32478=CARTESIAN_POINT('',(-0.7475,-1.95907305151415E-14,-1.33003901172249));
#32479=CARTESIAN_POINT('Ctrl Pts',(-0.747472002174668,1.61159471936609E-5,
-0.862144274880388));
#32480=CARTESIAN_POINT('Ctrl Pts',(-0.747402682287736,-0.0840439390973367,
-0.85975184069876));
#32481=CARTESIAN_POINT('Ctrl Pts',(-0.712650382827925,-0.290361716183338,
-0.853881418982972));
#32482=CARTESIAN_POINT('Ctrl Pts',(-0.526440462347927,-0.573013576696855,
-0.844533009733022));
#32483=CARTESIAN_POINT('Ctrl Pts',(-0.194520560057907,-0.753422770554806,
-0.834099047130545));
#32484=CARTESIAN_POINT('Ctrl Pts',(0.183249666810382,-0.75624313490388,
-0.823665084528061));
#32485=CARTESIAN_POINT('Ctrl Pts',(0.517826224589069,-0.580809883355642,
-0.813231121925582));
#32486=CARTESIAN_POINT('Ctrl Pts',(0.730346273449163,-0.268474282445113,
-0.802797159323101));
#32487=CARTESIAN_POINT('Ctrl Pts',(0.770716840097934,0.107143230607854,
-0.79236319672062));
#32488=CARTESIAN_POINT('Ctrl Pts',(0.629422202475751,0.457506077015547,
-0.781929234118141));
#32489=CARTESIAN_POINT('Ctrl Pts',(0.339766834898865,0.700030440322704,
-0.771495271515659));
#32490=CARTESIAN_POINT('Ctrl Pts',(-0.0299747696136733,0.777551048267703,
-0.76106130891318));
#32491=CARTESIAN_POINT('Ctrl Pts',(-0.392651039152918,0.671795564831834,
-0.750627346310697));
#32492=CARTESIAN_POINT('Ctrl Pts',(-0.662775767680288,0.407691551606601,
-0.740193383708218));
#32493=CARTESIAN_POINT('Ctrl Pts',(-0.743438739207481,0.152605612016257,
-0.732804289722675));
#32494=CARTESIAN_POINT('Ctrl Pts',(-0.747550058881758,0.0152273129384333,
-0.728893183271293));
#32495=CARTESIAN_POINT('Ctrl Pts',(-0.747537418840408,1.31793815494417E-5,
-0.728460064354072));
#32496=CARTESIAN_POINT('Ctrl Pts',(-0.747440403350747,2.49991181703463E-7,
-0.855618883014348));
#32497=CARTESIAN_POINT('Ctrl Pts',(-0.747439664227336,-0.0613952789202318,
-0.853871716067446));
#32498=CARTESIAN_POINT('Ctrl Pts',(-0.725057127938405,-0.245007983420982,
-0.848646561586384));
#32499=CARTESIAN_POINT('Ctrl Pts',(-0.576325689361536,-0.522812412838008,
-0.83994341957116));
#32500=CARTESIAN_POINT('Ctrl Pts',(-0.262170190030731,-0.732632862145289,
-0.82950945696868));
#32501=CARTESIAN_POINT('Ctrl Pts',(0.113781287599418,-0.769764858789943,
-0.819075494366201));
#32502=CARTESIAN_POINT('Ctrl Pts',(0.462913446150841,-0.625456042107332,
-0.808641531763718));
#32503=CARTESIAN_POINT('Ctrl Pts',(0.702932553865032,-0.333721356752229,
-0.79820756916124));
#32504=CARTESIAN_POINT('Ctrl Pts',(0.77726385077405,0.0366745895092527,
-0.787773606558758));
#32505=CARTESIAN_POINT('Ctrl Pts',(0.668386751451239,0.398425990267,-0.777339643956278));
#32506=CARTESIAN_POINT('Ctrl Pts',(0.401964611697131,0.666264639748313,
-0.766905681353798));
#32507=CARTESIAN_POINT('Ctrl Pts',(0.040795634331005,0.777058450475451,
-0.756471718751315));
#32508=CARTESIAN_POINT('Ctrl Pts',(-0.329989257542916,0.704692279751986,
-0.746037756148836));
#32509=CARTESIAN_POINT('Ctrl Pts',(-0.622992579377319,0.46622351428963,
-0.735603793546354));
#32510=CARTESIAN_POINT('Ctrl Pts',(-0.735537269423189,0.19797773894019,
-0.727569432326087));
#32511=CARTESIAN_POINT('Ctrl Pts',(-0.747504115891486,0.0379060617849294,
-0.72301305863998));
#32512=CARTESIAN_POINT('Ctrl Pts',(-0.747472643624562,1.6210341721886E-5,
-0.721934672488032));
#32513=CARTESIAN_POINT('Origin',(0.,0.,-1.33003901172249));
#32514=CARTESIAN_POINT('',(-0.747440394010334,2.88097106332193E-8,-0.995828485406703));
#32515=CARTESIAN_POINT('',(-0.747471187093045,-1.59917937688214E-5,-0.989303093540664));
#32516=CARTESIAN_POINT('',(-0.7475,-1.95907305151415E-14,-1.33003901172249));
#32517=CARTESIAN_POINT('Ctrl Pts',(-0.747440394010334,2.88097106414253E-8,
-0.995828485406703));
#32518=CARTESIAN_POINT('Ctrl Pts',(-0.747440305752117,-0.0611436444929983,
-0.994088485660386));
#32519=CARTESIAN_POINT('Ctrl Pts',(-0.72518211407954,-0.244504027566076,
-0.988870498379908));
#32520=CARTESIAN_POINT('Ctrl Pts',(-0.576853733233578,-0.522229725565815,
-0.980174523565273));
#32521=CARTESIAN_POINT('Ctrl Pts',(-0.262910442753167,-0.732367543071951,
-0.969740560962789));
#32522=CARTESIAN_POINT('Ctrl Pts',(0.113003322331734,-0.769879451565163,
-0.959306598360312));
#32523=CARTESIAN_POINT('Ctrl Pts',(0.462281136078415,-0.62592353336717,
-0.948872635757828));
#32524=CARTESIAN_POINT('Ctrl Pts',(0.702594943458043,-0.334431555819591,
-0.938438673155349));
#32525=CARTESIAN_POINT('Ctrl Pts',(0.777300516433143,0.0358890839459625,
-0.928004710552868));
#32526=CARTESIAN_POINT('Ctrl Pts',(0.668789051521523,0.397750328889649,
-0.917570747950388));
#32527=CARTESIAN_POINT('Ctrl Pts',(0.402637719871008,0.665858082479754,
-0.907136785347906));
#32528=CARTESIAN_POINT('Ctrl Pts',(0.0415808928872853,0.777016826591823,
-0.896702822745427));
#32529=CARTESIAN_POINT('Ctrl Pts',(-0.329276941530812,0.705025400441648,
-0.886268860142945));
#32530=CARTESIAN_POINT('Ctrl Pts',(-0.622521105437113,0.466852859850312,
-0.875834897540466));
#32531=CARTESIAN_POINT('Ctrl Pts',(-0.735437461077155,0.198481764760452,
-0.867793369119612));
#32532=CARTESIAN_POINT('Ctrl Pts',(-0.747503455677645,0.038157886060821,
-0.86322982823292));
#32533=CARTESIAN_POINT('Ctrl Pts',(-0.747472002174668,1.61159471936609E-5,
-0.862144274880388));
#32534=CARTESIAN_POINT('Ctrl Pts',(-0.747471187093045,-1.59917937688492E-5,
-0.989303093540664));
#32535=CARTESIAN_POINT('Ctrl Pts',(-0.747502606642687,-0.0384803988601526,
-0.988208361029073));
#32536=CARTESIAN_POINT('Ctrl Pts',(-0.735309243690986,-0.199127278369176,
-0.983635640983321));
#32537=CARTESIAN_POINT('Ctrl Pts',(-0.621916351700688,-0.467658178639457,
-0.975584933403408));
#32538=CARTESIAN_POINT('Ctrl Pts',(-0.328364174807739,-0.705450981188055,
-0.965150970800928));
#32539=CARTESIAN_POINT('Ctrl Pts',(0.0425865250681795,-0.776962359283856,
-0.954717008198448));
#32540=CARTESIAN_POINT('Ctrl Pts',(0.403499180542327,-0.665336403825431,
-0.944283045595967));
#32541=CARTESIAN_POINT('Ctrl Pts',(0.669303286159028,-0.39688440440999,
-0.933849082993487));
#32542=CARTESIAN_POINT('Ctrl Pts',(0.777346315469044,-0.0348830195569227,
-0.923415120391006));
#32543=CARTESIAN_POINT('Ctrl Pts',(0.702161510858137,0.335340620697416,
-0.912981157788526));
#32544=CARTESIAN_POINT('Ctrl Pts',(0.461470637519422,0.626521324425118,
-0.902547195186045));
#32545=CARTESIAN_POINT('Ctrl Pts',(0.112006796904714,0.770025062366403,
-0.892113232583564));
#32546=CARTESIAN_POINT('Ctrl Pts',(-0.263858098652974,0.732026654580471,
-0.881679269981083));
#32547=CARTESIAN_POINT('Ctrl Pts',(-0.577529159980994,0.521482682939162,
-0.871245307378604));
#32548=CARTESIAN_POINT('Ctrl Pts',(-0.72534176137517,0.24385860707159,-0.862558511723024));
#32549=CARTESIAN_POINT('Ctrl Pts',(-0.747441135558977,0.0608213670538152,
-0.857349703601606));
#32550=CARTESIAN_POINT('Ctrl Pts',(-0.747440403350747,2.49991181703463E-7,
-0.855618883014348));
#32551=CARTESIAN_POINT('Origin',(0.,0.,-1.33003901172249));
#32552=CARTESIAN_POINT('',(-0.7475,-1.95907305151415E-14,-1.12625));
#32553=CARTESIAN_POINT('',(-0.747536615034749,-1.54000427280421E-5,-1.12298730406698));
#32554=CARTESIAN_POINT('',(-0.7475,-1.95907305151415E-14,-1.33003901172249));
#32555=CARTESIAN_POINT('',(-0.738728321778977,-0.114178441930235,-1.12625));
#32556=CARTESIAN_POINT('Origin',(0.,0.,-1.12625));
#32557=CARTESIAN_POINT('Ctrl Pts',(-0.738728321778978,-0.114178441930233,
-1.12625));
#32558=CARTESIAN_POINT('Ctrl Pts',(-0.720064014057805,-0.23493549980332,
-1.12277201246584));
#32559=CARTESIAN_POINT('Ctrl Pts',(-0.622428467720143,-0.467011987146764,
-1.11581603739752));
#32560=CARTESIAN_POINT('Ctrl Pts',(-0.329058176975965,-0.705127368582219,
-1.10538207479504));
#32561=CARTESIAN_POINT('Ctrl Pts',(0.0417919283474094,-0.777000661774149,
-1.09494811219256));
#32562=CARTESIAN_POINT('Ctrl Pts',(0.402831360764579,-0.665746034504356,
-1.08451414959008));
#32563=CARTESIAN_POINT('Ctrl Pts',(0.668899442574653,-0.397559467050135,
-1.0740801869876));
#32564=CARTESIAN_POINT('Ctrl Pts',(0.777311895666571,-0.0356691406410416,
-1.06364622438512));
#32565=CARTESIAN_POINT('Ctrl Pts',(0.702499416237836,0.334631148448012,
-1.05321226178264));
#32566=CARTESIAN_POINT('Ctrl Pts',(0.46210386898375,0.626054505003765,-1.04277829918015));
#32567=CARTESIAN_POINT('Ctrl Pts',(0.112784749994036,0.769911552166375,
-1.03234433657768));
#32568=CARTESIAN_POINT('Ctrl Pts',(-0.26311811085717,0.732292892594134,
-1.02191037397519));
#32569=CARTESIAN_POINT('Ctrl Pts',(-0.577001907123836,0.522066075167687,
-1.01147641137271));
#32570=CARTESIAN_POINT('Ctrl Pts',(-0.72521712885417,0.24436255769002,-1.00278244851655));
#32571=CARTESIAN_POINT('Ctrl Pts',(-0.747440482166499,0.0610730017965627,
-0.997566473194546));
#32572=CARTESIAN_POINT('Ctrl Pts',(-0.747440394010334,2.88097106414253E-8,
-0.995828485406703));
#32573=CARTESIAN_POINT('Ctrl Pts',(-0.747536615034749,-1.54000427279987E-5,
-1.12298730406698));
#32574=CARTESIAN_POINT('Ctrl Pts',(-0.747549574643972,-0.0155531187576177,
-1.1225450059907));
#32575=CARTESIAN_POINT('Ctrl Pts',(-0.743340401009097,-0.153262521212319,
-1.11862472038026));
#32576=CARTESIAN_POINT('Ctrl Pts',(-0.662248238305507,-0.408538693637011,
-1.11122644723566));
#32577=CARTESIAN_POINT('Ctrl Pts',(-0.391780881856493,-0.672308433025167,
-1.10079248463318));
#32578=CARTESIAN_POINT('Ctrl Pts',(-0.0289685614302378,-0.777586532369439,
-1.0903585220307));
#32579=CARTESIAN_POINT('Ctrl Pts',(0.34067266544482,-0.699591456600571,
-1.07992455942821));
#32580=CARTESIAN_POINT('Ctrl Pts',(0.630013764781801,-0.456690366635246,
-1.06949059682574));
#32581=CARTESIAN_POINT('Ctrl Pts',(0.770854889346008,-0.10614597677494,
-1.05905663422325));
#32582=CARTESIAN_POINT('Ctrl Pts',(0.729998172573568,0.269419497799131,
-1.04862267162077));
#32583=CARTESIAN_POINT('Ctrl Pts',(0.517074073818031,0.581479511865621,
-1.03818870901829));
#32584=CARTESIAN_POINT('Ctrl Pts',(0.182270729955255,0.756479721113076,
-1.02775474641581));
#32585=CARTESIAN_POINT('Ctrl Pts',(-0.195495525574094,0.753170354596226,
-1.01732078381333));
#32586=CARTESIAN_POINT('Ctrl Pts',(-0.527181654493517,0.572331754114923,
-1.00688682121085));
#32587=CARTESIAN_POINT('Ctrl Pts',(-0.712843111741136,0.289716880061177,
-0.997547591119961));
#32588=CARTESIAN_POINT('Ctrl Pts',(-0.747402786092163,0.083721807495523,
-0.991686348563233));
#32589=CARTESIAN_POINT('Ctrl Pts',(-0.747471187093045,-1.59917937688492E-5,
-0.989303093540664));
#32590=CARTESIAN_POINT('Ctrl Pts',(0.82685,-3.02682447659827E-15,-1.12625));
#32591=CARTESIAN_POINT('Ctrl Pts',(0.82685,0.135161967341268,-1.12277201246584));
#32592=CARTESIAN_POINT('Ctrl Pts',(0.759329854291358,0.405358483866949,
-1.11581603739752));
#32593=CARTESIAN_POINT('Ctrl Pts',(0.478857035684594,0.715228292912727,
-1.10538207479504));
#32594=CARTESIAN_POINT('Ctrl Pts',(0.0855976892416237,0.85645773182655,
-1.09494811219256));
#32595=CARTESIAN_POINT('Ctrl Pts',(-0.327878991306296,0.795839011623234,
-1.08451414959008));
#32596=CARTESIAN_POINT('Ctrl Pts',(-0.664050737432062,0.547619885496961,
-1.0740801869876));
#32597=CARTESIAN_POINT('Ctrl Pts',(-0.84371003918773,0.170328555651515,
-1.06364622438512));
#32598=CARTESIAN_POINT('Ctrl Pts',(-0.824493582456408,-0.247114352893222,
-1.05321226178264));
#32599=CARTESIAN_POINT('Ctrl Pts',(-0.610938970960343,-0.606308285553784,
-1.04277829918015));
#32600=CARTESIAN_POINT('Ctrl Pts',(-0.253378910006021,-0.82259057174209,
-1.03234433657767));
#32601=CARTESIAN_POINT('Ctrl Pts',(0.163904234062435,-0.844980061330928,
-1.02191037397519));
#32602=CARTESIAN_POINT('Ctrl Pts',(0.542553969616097,-0.668200044521288,
-1.01147641137271));
#32603=CARTESIAN_POINT('Ctrl Pts',(0.793318450980058,-0.333918875136032,
-1.00104244877023));
#32604=CARTESIAN_POINT('Ctrl Pts',(0.857090409214355,0.0790700506594116,
-0.990608486167751));
#32605=CARTESIAN_POINT('Ctrl Pts',(0.718838053513711,0.47342145348791,-0.980174523565272));
#32606=CARTESIAN_POINT('Ctrl Pts',(0.411148835382881,0.756182953459404,
-0.96974056096279));
#32607=CARTESIAN_POINT('Ctrl Pts',(0.00654795948643633,0.860705030962387,
-0.959306598360311));
#32608=CARTESIAN_POINT('Ctrl Pts',(-0.399596325757394,0.762350837560662,
-0.948872635757829));
#32609=CARTESIAN_POINT('Ctrl Pts',(-0.711552003832336,0.484303387427028,
-0.938438673155349));
#32610=CARTESIAN_POINT('Ctrl Pts',(-0.855788184097908,0.0921010751558475,
-0.928004710552867));
#32611=CARTESIAN_POINT('Ctrl Pts',(-0.798307045430395,-0.321810325775008,
-0.917570747950388));
#32612=CARTESIAN_POINT('Ctrl Pts',(-0.552657431316075,-0.659868008045783,
-0.907136785347907));
#32613=CARTESIAN_POINT('Ctrl Pts',(-0.176741265643768,-0.842388597645021,
-0.896702822745426));
#32614=CARTESIAN_POINT('Ctrl Pts',(0.240834477891075,-0.826350276046737,
-0.886268860142946));
#32615=CARTESIAN_POINT('Ctrl Pts',(0.60164327098714,-0.615533426310556,
-0.875834897540465));
#32616=CARTESIAN_POINT('Ctrl Pts',(0.820639089442,-0.259629561740577,-0.865400934937984));
#32617=CARTESIAN_POINT('Ctrl Pts',(0.846202560151336,0.15747143116726,-0.854966972335505));
#32618=CARTESIAN_POINT('Ctrl Pts',(0.672308132783287,0.537454927447039,
-0.844533009733023));
#32619=CARTESIAN_POINT('Ctrl Pts',(0.339944358537648,0.790755245029512,
-0.834099047130544));
#32620=CARTESIAN_POINT('Ctrl Pts',(-0.0725474966321842,0.857667117928167,
-0.823665084528062));
#32621=CARTESIAN_POINT('Ctrl Pts',(-0.467939224870045,0.722418788703156,
-0.813231121925582));
#32622=CARTESIAN_POINT('Ctrl Pts',(-0.75303327898166,0.416889559942562,
-0.802797159323101));
#32623=CARTESIAN_POINT('Ctrl Pts',(-0.860630310410644,0.0130955429679302,
-0.79236319672062));
#32624=CARTESIAN_POINT('Ctrl Pts',(-0.765368687391838,-0.393785216587893,
-0.78192923411814));
#32625=CARTESIAN_POINT('Ctrl Pts',(-0.489702469969954,-0.70784709884863,
-0.771495271515659));
#32626=CARTESIAN_POINT('Ctrl Pts',(-0.0986087769686508,-0.855062765852803,
-0.761061308913178));
#32627=CARTESIAN_POINT('Ctrl Pts',(0.315727931727778,-0.800732100998825,
-0.750627346310699));
#32628=CARTESIAN_POINT('Ctrl Pts',(0.655644598941733,-0.557661352723703,
-0.740193383708217));
#32629=CARTESIAN_POINT('Ctrl Pts',(0.841019670852427,-0.183144581362294,
-0.729759421105737));
#32630=CARTESIAN_POINT('Ctrl Pts',(0.828158500407521,0.234541089461659,
-0.719325458503256));
#32631=CARTESIAN_POINT('Ctrl Pts',(0.620092586381243,0.596943220715435,
-0.708891495900776));
#32632=CARTESIAN_POINT('Ctrl Pts',(0.265865020615963,0.818640223331329,
-0.698457533298294));
#32633=CARTESIAN_POINT('Ctrl Pts',(-0.151029429750584,0.847376029748488,
-0.688023570695815));
#32634=CARTESIAN_POINT('Ctrl Pts',(-0.532324823785286,0.676377340265815,
-0.677589608093333));
#32635=CARTESIAN_POINT('Ctrl Pts',(-0.788146252778427,0.345950153453385,
-0.667155645490854));
#32636=CARTESIAN_POINT('Ctrl Pts',(-0.858194201088188,-0.0660207366037423,
-0.656721682888372));
#32637=CARTESIAN_POINT('Ctrl Pts',(-0.725957708818034,-0.462429918420906,
-0.646287720285892));
#32638=CARTESIAN_POINT('Ctrl Pts',(-0.422606160274219,-0.749840021432156,
-0.635853757683412));
#32639=CARTESIAN_POINT('Ctrl Pts',(-0.0196423670795997,-0.860505782582898,
-0.625419795080931));
#32640=CARTESIAN_POINT('Ctrl Pts',(0.387951316682125,-0.768342241665588,
-0.61498583247845));
#32641=CARTESIAN_POINT('Ctrl Pts',(0.704101228197687,-0.495073211650161,
-0.604551869875969));
#32642=CARTESIAN_POINT('Ctrl Pts',(0.854287861381835,-0.105110771754113,
-0.594117907273489));
#32643=CARTESIAN_POINT('Ctrl Pts',(0.803110814976077,0.309627265129475,
-0.583683944671009));
#32644=CARTESIAN_POINT('Ctrl Pts',(0.562632999903826,0.651383244996612,
-0.573249982068528));
#32645=CARTESIAN_POINT('Ctrl Pts',(0.189537297769379,0.839602070743859,
-0.562816019466046));
#32646=CARTESIAN_POINT('Ctrl Pts',(-0.228234127178964,0.829918795807127,
-0.552382056863568));
#32647=CARTESIAN_POINT('Ctrl Pts',(-0.592208622855233,0.624615859115826,
-0.541948094261085));
#32648=CARTESIAN_POINT('Ctrl Pts',(-0.816593979116471,0.272085092781331,
-0.531514131658606));
#32649=CARTESIAN_POINT('Ctrl Pts',(-0.848500458175959,-0.14457868763508,
-0.521080169056125));
#32650=CARTESIAN_POINT('Ctrl Pts',(-0.68040740298517,-0.527163912275938,
-0.510646206453644));
#32651=CARTESIAN_POINT('Ctrl Pts',(-0.351935926797396,-0.785491647232708,
-0.500212243851164));
#32652=CARTESIAN_POINT('Ctrl Pts',(0.0594901556810227,-0.858671616987626,
-0.489778281248683));
#32653=CARTESIAN_POINT('Ctrl Pts',(0.456893849233147,-0.729454614747217,
-0.479344318646202));
#32654=CARTESIAN_POINT('Ctrl Pts',(0.746603367528272,-0.428298302633273,
-0.468910356043722));
#32655=CARTESIAN_POINT('Ctrl Pts',(0.86033145371393,-0.026188054405967,
-0.458476393441242));
#32656=CARTESIAN_POINT('Ctrl Pts',(0.771271328784717,0.382094964423424,
-0.44804243083876));
#32657=CARTESIAN_POINT('Ctrl Pts',(0.500415301388769,0.700314608286257,
-0.43760846823628));
#32658=CARTESIAN_POINT('Ctrl Pts',(0.111606683342934,0.853463515726457,
-0.427174505633799));
#32659=CARTESIAN_POINT('Ctrl Pts',(-0.303508679116189,0.805443049597213,
-0.416740543031319));
#32660=CARTESIAN_POINT('Ctrl Pts',(-0.647084192799484,0.567572085176716,
-0.406306580428838));
#32661=CARTESIAN_POINT('Ctrl Pts',(-0.838135879378579,0.195919044866888,
-0.395872617826358));
#32662=CARTESIAN_POINT('Ctrl Pts',(-0.831631060361419,-0.221913956041062,
-0.385438655223877));
#32663=CARTESIAN_POINT('Ctrl Pts',(-0.629102982738006,-0.587439751421952,
-0.375004692621396));
#32664=CARTESIAN_POINT('Ctrl Pts',(-0.27828941825328,-0.814500475222728,
-0.364570730018916));
#32665=CARTESIAN_POINT('Ctrl Pts',(0.138119578151258,-0.849575780352193,
-0.354136767416435));
#32666=CARTESIAN_POINT('Ctrl Pts',(0.521972491602107,-0.68439808771962,
-0.343702804813955));
#32667=CARTESIAN_POINT('Ctrl Pts',(0.782791582026738,-0.357901332117923,
-0.333268842211474));
#32668=CARTESIAN_POINT('Ctrl Pts',(0.859099337993374,0.0529561317558155,
-0.322834879608993));
#32669=CARTESIAN_POINT('Ctrl Pts',(0.732909304116493,0.451331337820343,
-0.312400917006513));
#32670=CARTESIAN_POINT('Ctrl Pts',(0.433965657579446,0.743323504356007,
-0.301966954404032));
#32671=CARTESIAN_POINT('Ctrl Pts',(0.0327322261453305,0.860107334350009,
-0.291532991801552));
#32672=CARTESIAN_POINT('Ctrl Pts',(-0.376216498791157,0.774155778332486,
-0.281099029199071));
#32673=CARTESIAN_POINT('Ctrl Pts',(-0.696487458167497,0.505728431782095,
-0.27066506659659));
#32674=CARTESIAN_POINT('Ctrl Pts',(-0.85258977678019,0.11809613232106,-0.26023110399411));
#32675=CARTESIAN_POINT('Ctrl Pts',(-0.807728669522179,-0.297372520979856,
-0.249797141391629));
#32676=CARTESIAN_POINT('Ctrl Pts',(-0.572478323412184,-0.642747704547972,
-0.239363178789149));
#32677=CARTESIAN_POINT('Ctrl Pts',(-0.202289451911266,-0.836621155292497,
-0.228929216186668));
#32678=CARTESIAN_POINT('Ctrl Pts',(0.215580939060966,-0.833295246691129,
-0.218495253584187));
#32679=CARTESIAN_POINT('Ctrl Pts',(0.582636887836429,-0.633553595935411,
-0.208061290981707));
#32680=CARTESIAN_POINT('Ctrl Pts',(0.812359822146787,-0.284477837654288,
-0.197627328379226));
#32681=CARTESIAN_POINT('Ctrl Pts',(0.850601954996979,0.131652867513652,
-0.187193365776746));
#32682=CARTESIAN_POINT('Ctrl Pts',(0.688349122337921,0.51675009114102,-0.176759403174265));
#32683=CARTESIAN_POINT('Ctrl Pts',(0.363846105084835,0.780047728610939,
-0.166325440571784));
#32684=CARTESIAN_POINT('Ctrl Pts',(-0.0464192020363249,0.859474361780549,
-0.155891477969304));
#32685=CARTESIAN_POINT('Ctrl Pts',(-0.445742392858126,0.736327430271745,
-0.145457515366823));
#32686=CARTESIAN_POINT('Ctrl Pts',(-0.740001245121628,0.439596369442954,
-0.135023552764343));
#32687=CARTESIAN_POINT('Ctrl Pts',(-0.859832124525603,0.0392974457347639,
-0.124589590161862));
#32688=CARTESIAN_POINT('Ctrl Pts',(-0.776998977184784,-0.370364573784867,
-0.114155627559381));
#32689=CARTESIAN_POINT('Ctrl Pts',(-0.599661254481026,-0.585112006191809,
-0.107199652491061));
#32690=CARTESIAN_POINT('Ctrl Pts',(-0.490897892427245,-0.665357183556688,
-0.103721664956901));
#32691=CARTESIAN_POINT('Ctrl Pts',(0.82685,-3.02682447659827E-15,-1.12910983122651));
#32692=CARTESIAN_POINT('Ctrl Pts',(0.82685,0.135162380594788,-1.12563184369234));
#32693=CARTESIAN_POINT('Ctrl Pts',(0.759329891769105,0.405358236621017,
-1.11867586862402));
#32694=CARTESIAN_POINT('Ctrl Pts',(0.478857042724245,0.715228435638403,
-1.10824190602154));
#32695=CARTESIAN_POINT('Ctrl Pts',(0.0855976953161789,0.856457696102362,
-1.09780794341906));
#32696=CARTESIAN_POINT('Ctrl Pts',(-0.327879002777267,0.795839066043265,
-1.08737398081658));
#32697=CARTESIAN_POINT('Ctrl Pts',(-0.664050756097956,0.547619885902201,
-1.0769400182141));
#32698=CARTESIAN_POINT('Ctrl Pts',(-0.843710064534722,0.1703285686858,-1.06650605561162));
#32699=CARTESIAN_POINT('Ctrl Pts',(-0.824493606532926,-0.247114364257445,
-1.05607209300914));
#32700=CARTESIAN_POINT('Ctrl Pts',(-0.610938989097404,-0.606308301358732,
-1.04563813040666));
#32701=CARTESIAN_POINT('Ctrl Pts',(-0.253378917416559,-0.822590597055703,
-1.03520416780418));
#32702=CARTESIAN_POINT('Ctrl Pts',(0.163904238864601,-0.84498008571162,
-1.0247702052017));
#32703=CARTESIAN_POINT('Ctrl Pts',(0.542553985631648,-0.6682000644996,-1.01433624259922));
#32704=CARTESIAN_POINT('Ctrl Pts',(0.793318474366499,-0.333918884843967,
-1.00390227999674));
#32705=CARTESIAN_POINT('Ctrl Pts',(0.857090434493622,0.0790700529203285,
-0.993468317394256));
#32706=CARTESIAN_POINT('Ctrl Pts',(0.718838074709768,0.473421467484897,
-0.983034354791778));
#32707=CARTESIAN_POINT('Ctrl Pts',(0.411148847508511,0.756182975740501,
-0.972600392189296));
#32708=CARTESIAN_POINT('Ctrl Pts',(0.00654795967898853,0.860705056353458,
-0.962166429586816));
#32709=CARTESIAN_POINT('Ctrl Pts',(-0.399596337541002,0.762350860037237,
-0.951732466984335));
#32710=CARTESIAN_POINT('Ctrl Pts',(-0.711552024815771,0.484303401711296,
-0.941298504381855));
#32711=CARTESIAN_POINT('Ctrl Pts',(-0.855788209334578,0.09210107787063,
-0.930864541779373));
#32712=CARTESIAN_POINT('Ctrl Pts',(-0.798307068972085,-0.321810335264399,
-0.920430579176894));
#32713=CARTESIAN_POINT('Ctrl Pts',(-0.552657447613633,-0.659868027505261,
-0.909996616574413));
#32714=CARTESIAN_POINT('Ctrl Pts',(-0.176741270855785,-0.842388622486455,
-0.899562653971931));
#32715=CARTESIAN_POINT('Ctrl Pts',(0.240834484993162,-0.826350300415453,
-0.889128691369452));
#32716=CARTESIAN_POINT('Ctrl Pts',(0.60164328872928,-0.61553344446227,-0.878694728766969));
#32717=CARTESIAN_POINT('Ctrl Pts',(0.820639113642216,-0.259629569396937,
-0.868260766164492));
#32718=CARTESIAN_POINT('Ctrl Pts',(0.846202585105402,0.15747143581102,-0.857826803562008));
#32719=CARTESIAN_POINT('Ctrl Pts',(0.6723081526093,0.537454943296297,-0.847392840959531));
#32720=CARTESIAN_POINT('Ctrl Pts',(0.339944368562428,0.79075526834847,-0.836958878357048));
#32721=CARTESIAN_POINT('Ctrl Pts',(-0.0725474987715713,0.857667143220318,
-0.826524915754568));
#32722=CARTESIAN_POINT('Ctrl Pts',(-0.467939238669326,0.722418810006905,
-0.816090953152087));
#32723=CARTESIAN_POINT('Ctrl Pts',(-0.753033301188214,0.416889572236416,
-0.805656990549607));
#32724=CARTESIAN_POINT('Ctrl Pts',(-0.860630335790178,0.0130955433541108,
-0.795223027947126));
#32725=CARTESIAN_POINT('Ctrl Pts',(-0.765368709962158,-0.393785228200412,
-0.784789065344646));
#32726=CARTESIAN_POINT('Ctrl Pts',(-0.489702484411021,-0.707847119722667,
-0.774355102742164));
#32727=CARTESIAN_POINT('Ctrl Pts',(-0.0986087798765718,-0.855062791068153,
-0.763921140139686));
#32728=CARTESIAN_POINT('Ctrl Pts',(0.315727941038429,-0.800732124611992,
-0.753487177537203));
#32729=CARTESIAN_POINT('Ctrl Pts',(0.655644618276346,-0.557661369168842,
-0.743053214934723));
#32730=CARTESIAN_POINT('Ctrl Pts',(0.841019695653653,-0.183144586763131,
-0.732619252332243));
#32731=CARTESIAN_POINT('Ctrl Pts',(0.828158524829479,0.234541096378151,
-0.722185289729762));
#32732=CARTESIAN_POINT('Ctrl Pts',(0.620092604667446,0.596943238318976,
-0.711751327127282));
#32733=CARTESIAN_POINT('Ctrl Pts',(0.265865028456182,0.818640247472598,
-0.7013173645248));
#32734=CARTESIAN_POINT('Ctrl Pts',(-0.151029434204362,0.847376054737159,
-0.690883401922321));
#32735=CARTESIAN_POINT('Ctrl Pts',(-0.532324839483263,0.676377360211827,
-0.680449439319839));
#32736=CARTESIAN_POINT('Ctrl Pts',(-0.788146276020444,0.345950163655273,
-0.670015476717359));
#32737=CARTESIAN_POINT('Ctrl Pts',(-0.858194226395883,-0.0660207385506592,
-0.659581514114878));
#32738=CARTESIAN_POINT('Ctrl Pts',(-0.725957730226144,-0.46242993205772,
-0.649147551512398));
#32739=CARTESIAN_POINT('Ctrl Pts',(-0.422606172736652,-0.749840043544544,
-0.638713588909917));
#32740=CARTESIAN_POINT('Ctrl Pts',(-0.0196423676588426,-0.860505807958758,
-0.628279626307437));
#32741=CARTESIAN_POINT('Ctrl Pts',(0.387951328122605,-0.768342264323596,
-0.617845663704956));
#32742=CARTESIAN_POINT('Ctrl Pts',(0.70410124896126,-0.495073226249608,
-0.607411701102476));
#32743=CARTESIAN_POINT('Ctrl Pts',(0.854287886574333,-0.105110774853774,
-0.596977738499994));
#32744=CARTESIAN_POINT('Ctrl Pts',(0.803110838659391,0.309627274260219,
-0.586543775897515));
#32745=CARTESIAN_POINT('Ctrl Pts',(0.562633016495577,0.65138326420556,-0.576109813295033));
#32746=CARTESIAN_POINT('Ctrl Pts',(0.189537303358733,0.839602095503281,
-0.565675850692553));
#32747=CARTESIAN_POINT('Ctrl Pts',(-0.228234133909468,0.829918820280995,
-0.555241888090073));
#32748=CARTESIAN_POINT('Ctrl Pts',(-0.592208640319154,0.624615877535418,
-0.544807925487591));
#32749=CARTESIAN_POINT('Ctrl Pts',(-0.816594003197396,0.272085100804978,
-0.534373962885111));
#32750=CARTESIAN_POINT('Ctrl Pts',(-0.84850048319779,-0.14457869189863,
-0.523940000282631));
#32751=CARTESIAN_POINT('Ctrl Pts',(-0.680407423050025,-0.527163927821724,
-0.513506037680149));
#32752=CARTESIAN_POINT('Ctrl Pts',(-0.351935937175801,-0.785491670396441,
-0.503072075077669));
#32753=CARTESIAN_POINT('Ctrl Pts',(0.0594901574353558,-0.8586716423094,
-0.492638112475189));
#32754=CARTESIAN_POINT('Ctrl Pts',(0.456893862706706,-0.729454636258448,
-0.482204149872708));
#32755=CARTESIAN_POINT('Ctrl Pts',(0.746603389545211,-0.428298315263564,
-0.471770187270228));
#32756=CARTESIAN_POINT('Ctrl Pts',(0.860331479084652,-0.0261880551782389,
-0.461336224667747));
#32757=CARTESIAN_POINT('Ctrl Pts',(0.771271351529101,0.382094975691203,
-0.450902262065267));
#32758=CARTESIAN_POINT('Ctrl Pts',(0.500415316145753,0.700314628938165,
-0.440468299462785));
#32759=CARTESIAN_POINT('Ctrl Pts',(0.111606686634156,0.853463540894646,
-0.430034336860305));
#32760=CARTESIAN_POINT('Ctrl Pts',(-0.3035086880665,0.805443073349304,-0.419600374257825));
#32761=CARTESIAN_POINT('Ctrl Pts',(-0.647084211881655,0.567572101914117,
-0.409166411655343));
#32762=CARTESIAN_POINT('Ctrl Pts',(-0.838135904094766,0.195919050644438,
-0.398732449052864));
#32763=CARTESIAN_POINT('Ctrl Pts',(-0.831631084885775,-0.22191396258519,
-0.388298486450382));
#32764=CARTESIAN_POINT('Ctrl Pts',(-0.62910300128993,-0.587439768745234,
-0.377864523847903));
#32765=CARTESIAN_POINT('Ctrl Pts',(-0.278289426459872,-0.814500499241931,
-0.367430561245421));
#32766=CARTESIAN_POINT('Ctrl Pts',(0.138119582224299,-0.849575805405708,
-0.356996598642941));
#32767=CARTESIAN_POINT('Ctrl Pts',(0.521972506994863,-0.684398107902212,
-0.346562636040461));
#32768=CARTESIAN_POINT('Ctrl Pts',(0.782791605110725,-0.357901342672141,
-0.336128673437979));
#32769=CARTESIAN_POINT('Ctrl Pts',(0.859099363328006,0.05295613331726,-0.3256947108355));
#32770=CARTESIAN_POINT('Ctrl Pts',(0.73290932572912,0.451331351130267,-0.315260748233018));
#32771=CARTESIAN_POINT('Ctrl Pts',(0.433965670377812,0.743323526275438,
-0.304826785630539));
#32772=CARTESIAN_POINT('Ctrl Pts',(0.0327322271087253,0.860107359715668,
-0.294392823028057));
#32773=CARTESIAN_POINT('Ctrl Pts',(-0.376216509881926,0.774155801158889,
-0.283958860425577));
#32774=CARTESIAN_POINT('Ctrl Pts',(-0.696487478713732,0.505728446701738,
-0.273524897823096));
#32775=CARTESIAN_POINT('Ctrl Pts',(-0.85258980190849,0.118096135791905,
-0.263090935220616));
#32776=CARTESIAN_POINT('Ctrl Pts',(-0.807728693369426,-0.297372529726131,
-0.252656972618135));
#32777=CARTESIAN_POINT('Ctrl Pts',(-0.57247834023973,-0.642747723547624,
-0.242223010015654));
#32778=CARTESIAN_POINT('Ctrl Pts',(-0.202289457983844,-0.836621179874877,
-0.231789047413174));
#32779=CARTESIAN_POINT('Ctrl Pts',(0.21558094562892,-0.83329527143972,-0.221355084810693));
#32780=CARTESIAN_POINT('Ctrl Pts',(0.582636904604278,-0.633553614274392,
-0.210921122208213));
#32781=CARTESIAN_POINT('Ctrl Pts',(0.812359846915985,-0.284477846719709,
-0.200487159605732));
#32782=CARTESIAN_POINT('Ctrl Pts',(0.850601978482959,0.131652872725006,
-0.190053197003252));
#32783=CARTESIAN_POINT('Ctrl Pts',(0.68834914577673,0.516750103768234,-0.179619234400771));
#32784=CARTESIAN_POINT('Ctrl Pts',(0.363846109644706,0.780047756745796,
-0.16918527179829));
#32785=CARTESIAN_POINT('Ctrl Pts',(-0.0464191912805425,0.859474377041381,
-0.158751309195809));
#32786=CARTESIAN_POINT('Ctrl Pts',(-0.445742429839058,0.736327471811288,
-0.148317346593329));
#32787=CARTESIAN_POINT('Ctrl Pts',(-0.740001219981202,0.439596343345502,
-0.137883383990848));
#32788=CARTESIAN_POINT('Ctrl Pts',(-0.859832243554816,0.0392975248057583,
-0.127449421388368));
#32789=CARTESIAN_POINT('Ctrl Pts',(-0.776998800479081,-0.370364750731827,
-0.117015458785887));
#32790=CARTESIAN_POINT('Ctrl Pts',(-0.599661587021631,-0.58511176084467,
-0.110059483717567));
#32791=CARTESIAN_POINT('Ctrl Pts',(-0.490897892427245,-0.665357183556688,
-0.106581496183406));
#32792=CARTESIAN_POINT('Ctrl Pts',(0.825266255435535,-3.02102691136588E-15,
-1.13578682154469));
#32793=CARTESIAN_POINT('Ctrl Pts',(0.825266255435536,0.134902373133398,
-1.13230883401052));
#32794=CARTESIAN_POINT('Ctrl Pts',(0.75787537350136,0.40458248431603,-1.12535285894221));
#32795=CARTESIAN_POINT('Ctrl Pts',(0.477939823171875,0.713858104336506,
-1.11491889633972));
#32796=CARTESIAN_POINT('Ctrl Pts',(0.0854337254619215,0.854817337751033,
-1.10448493373724));
#32797=CARTESIAN_POINT('Ctrl Pts',(-0.327250953856659,0.794314572438199,
-1.09405097113476));
#32798=CARTESIAN_POINT('Ctrl Pts',(-0.662778785930793,0.546570976276213,
-1.08361700853228));
#32799=CARTESIAN_POINT('Ctrl Pts',(-0.842093957705064,0.170002286889038,
-1.0731830459298));
#32800=CARTESIAN_POINT('Ctrl Pts',(-0.822914310253025,-0.246641011830834,
-1.06274908332732));
#32801=CARTESIAN_POINT('Ctrl Pts',(-0.609768750387387,-0.605146938555681,
-1.05231512072484));
#32802=CARTESIAN_POINT('Ctrl Pts',(-0.252893576591472,-0.821014942444097,
-1.04188115812236));
#32803=CARTESIAN_POINT('Ctrl Pts',(0.163590284471113,-0.843361548903803,
-1.03144719551988));
#32804=CARTESIAN_POINT('Ctrl Pts',(0.541514736972467,-0.666920143216008,
-1.0210132329174));
#32805=CARTESIAN_POINT('Ctrl Pts',(0.791798892653785,-0.333279271931911,
-1.01057927031492));
#32806=CARTESIAN_POINT('Ctrl Pts',(0.855448699150101,0.0789185963993257,
-1.00014530771244));
#32807=CARTESIAN_POINT('Ctrl Pts',(0.717461158327155,0.47251464038409,-0.989711345109957));
#32808=CARTESIAN_POINT('Ctrl Pts',(0.41036130215142,0.754734526176119,-0.979277382507476));
#32809=CARTESIAN_POINT('Ctrl Pts',(0.00653541722714587,0.859056397277897,
-0.968843419904996));
#32810=CARTESIAN_POINT('Ctrl Pts',(-0.398830920732015,0.76089059600768,
-0.958409457302514));
#32811=CARTESIAN_POINT('Ctrl Pts',(-0.710189064673796,0.483375730628082,
-0.947975494700035));
#32812=CARTESIAN_POINT('Ctrl Pts',(-0.854148968382192,0.0919246605583472,
-0.937541532097554));
#32813=CARTESIAN_POINT('Ctrl Pts',(-0.796777931708911,-0.321193915602005,
-0.927107569495074));
#32814=CARTESIAN_POINT('Ctrl Pts',(-0.551598846068353,-0.658604066769503,
-0.916673606892593));
#32815=CARTESIAN_POINT('Ctrl Pts',(-0.176402727363294,-0.840775048108438,
-0.906239644290112));
#32816=CARTESIAN_POINT('Ctrl Pts',(0.240373172548915,-0.824767447042348,
-0.895805681687632));
#32817=CARTESIAN_POINT('Ctrl Pts',(0.600490856028098,-0.614354405514617,
-0.88537171908515));
#32818=CARTESIAN_POINT('Ctrl Pts',(0.819067199905029,-0.259132255437638,
-0.874937756482672));
#32819=CARTESIAN_POINT('Ctrl Pts',(0.844581705176757,0.157169803206536,
-0.864503793880189));
#32820=CARTESIAN_POINT('Ctrl Pts',(0.6710203631253,0.536425461768513,-0.85406983127771));
#32821=CARTESIAN_POINT('Ctrl Pts',(0.339293213610224,0.789240596370972,
-0.843635868675228));
#32822=CARTESIAN_POINT('Ctrl Pts',(-0.072408535848624,0.856024303216786,
-0.833201906072748));
#32823=CARTESIAN_POINT('Ctrl Pts',(-0.467042912738471,0.721035034809535,
-0.822767943470268));
#32824=CARTESIAN_POINT('Ctrl Pts',(-0.751590884697194,0.4160910306673,-0.812333980867786));
#32825=CARTESIAN_POINT('Ctrl Pts',(-0.858981819865243,0.0130704591677099,
-0.801900018265307));
#32826=CARTESIAN_POINT('Ctrl Pts',(-0.763902665303551,-0.393030942425559,
-0.791466055662826));
#32827=CARTESIAN_POINT('Ctrl Pts',(-0.488764471526209,-0.706491256234296,
-0.781032093060345));
#32828=CARTESIAN_POINT('Ctrl Pts',(-0.0984198972202151,-0.853424939636155,
-0.770598130457865));
#32829=CARTESIAN_POINT('Ctrl Pts',(0.315123172048649,-0.799198342215373,
-0.760164167855384));
#32830=CARTESIAN_POINT('Ctrl Pts',(0.654388747376404,-0.556593182736683,
-0.749730205252903));
#32831=CARTESIAN_POINT('Ctrl Pts',(0.839408743420373,-0.182793777878888,
-0.739296242650423));
#32832=CARTESIAN_POINT('Ctrl Pts',(0.826572207847869,0.234091838762714,
-0.728862280047942));
#32833=CARTESIAN_POINT('Ctrl Pts',(0.618904832762113,0.595799808447022,
-0.718428317445461));
#32834=CARTESIAN_POINT('Ctrl Pts',(0.265355770630763,0.817072162513667,
-0.707994354842981));
#32835=CARTESIAN_POINT('Ctrl Pts',(-0.150740141093178,0.845752927056724,
-0.697560392240501));
#32836=CARTESIAN_POINT('Ctrl Pts',(-0.531305184541261,0.675081776262243,
-0.687126429638019));
#32837=CARTESIAN_POINT('Ctrl Pts',(-0.786636601502631,0.345287504752486,
-0.676692467035539));
#32838=CARTESIAN_POINT('Ctrl Pts',(-0.856550376777682,-0.065894277473992,
-0.666258504433058));
#32839=CARTESIAN_POINT('Ctrl Pts',(-0.724567176315434,-0.461544159066155,
-0.655824541830578));
#32840=CARTESIAN_POINT('Ctrl Pts',(-0.421796681161976,-0.748403743658829,
-0.645390579228098));
#32841=CARTESIAN_POINT('Ctrl Pts',(-0.01960474319391,-0.858857530563777,
-0.634956616625617));
#32842=CARTESIAN_POINT('Ctrl Pts',(0.387208217037725,-0.766870523895836,
-0.624522654023136));
#32843=CARTESIAN_POINT('Ctrl Pts',(0.702752560594826,-0.49412492584287,
-0.614088691420655));
#32844=CARTESIAN_POINT('Ctrl Pts',(0.85265151945255,-0.104909437788343,
-0.603654728818175));
#32845=CARTESIAN_POINT('Ctrl Pts',(0.801572499895393,0.309034190945368,
-0.593220766215694));
#32846=CARTESIAN_POINT('Ctrl Pts',(0.561555306997066,0.650135555822967,
-0.582786803613213));
#32847=CARTESIAN_POINT('Ctrl Pts',(0.189174249385427,0.837993858647703,
-0.572352841010733));
#32848=CARTESIAN_POINT('Ctrl Pts',(-0.227796957123202,0.828329131497389,
-0.561918878408252));
#32849=CARTESIAN_POINT('Ctrl Pts',(-0.591074279451483,0.623419441413817,
-0.551484915805771));
#32850=CARTESIAN_POINT('Ctrl Pts',(-0.815029837768296,0.271563928586243,
-0.541050953203291));
#32851=CARTESIAN_POINT('Ctrl Pts',(-0.846875201702707,-0.144301755023308,
-0.53061699060081));
#32852=CARTESIAN_POINT('Ctrl Pts',(-0.679104119615673,-0.52615415847718,
-0.520183027998331));
#32853=CARTESIAN_POINT('Ctrl Pts',(-0.351261812673254,-0.783987080709439,
-0.509749065395849));
#32854=CARTESIAN_POINT('Ctrl Pts',(0.0593762055237968,-0.857026878212932,
-0.499315102793369));
#32855=CARTESIAN_POINT('Ctrl Pts',(0.456018693917791,-0.728057384111526,
-0.488881140190888));
#32856=CARTESIAN_POINT('Ctrl Pts',(0.745173289389437,-0.427477920531967,
-0.478447177588408));
#32857=CARTESIAN_POINT('Ctrl Pts',(0.858683535612277,-0.0261378926122579,
-0.468013214985927));
#32858=CARTESIAN_POINT('Ctrl Pts',(0.769794000507915,0.381363082303218,
-0.457579252383447));
#32859=CARTESIAN_POINT('Ctrl Pts',(0.499456783099169,0.698973193747863,
-0.447145289780966));
#32860=CARTESIAN_POINT('Ctrl Pts',(0.111392906811862,0.851828752786434,
-0.436711327178486));
#32861=CARTESIAN_POINT('Ctrl Pts',(-0.302927324750768,0.803900267247975,
-0.426277364576005));
#32862=CARTESIAN_POINT('Ctrl Pts',(-0.645844738226477,0.56648493172078,
-0.415843401973524));
#32863=CARTESIAN_POINT('Ctrl Pts',(-0.836530475692225,0.195543772593505,
-0.405409439371044));
#32864=CARTESIAN_POINT('Ctrl Pts',(-0.830038116302073,-0.221488891929322,
-0.394975476768563));
#32865=CARTESIAN_POINT('Ctrl Pts',(-0.627897970194763,-0.58631454253204,
-0.384541514166082));
#32866=CARTESIAN_POINT('Ctrl Pts',(-0.277756370010263,-0.812940343867362,
-0.374107551563602));
#32867=CARTESIAN_POINT('Ctrl Pts',(0.137855017612411,-0.847948464157851,
-0.363673588961121));
#32868=CARTESIAN_POINT('Ctrl Pts',(0.520972681687152,-0.6830871604105,-0.353239626358641));
#32869=CARTESIAN_POINT('Ctrl Pts',(0.781292187331713,-0.357215791584557,
-0.34280566375616));
#32870=CARTESIAN_POINT('Ctrl Pts',(0.857453779941941,0.0528546971663474,
-0.33237170115368));
#32871=CARTESIAN_POINT('Ctrl Pts',(0.731505456212057,0.450466837192338,
-0.321937738551198));
#32872=CARTESIAN_POINT('Ctrl Pts',(0.4331344199664,0.741899708618019,-0.311503775948718));
#32873=CARTESIAN_POINT('Ctrl Pts',(0.0326695293498048,0.858459845534159,
-0.301069813346237));
#32874=CARTESIAN_POINT('Ctrl Pts',(-0.375495876558354,0.772672925054673,
-0.290635850743757));
#32875=CARTESIAN_POINT('Ctrl Pts',(-0.695153374314705,0.504759736470026,
-0.280201888141276));
#32876=CARTESIAN_POINT('Ctrl Pts',(-0.850956687463707,0.117869925623525,
-0.269767925538796));
#32877=CARTESIAN_POINT('Ctrl Pts',(-0.806181509144913,-0.296802920130984,
-0.259333962936315));
#32878=CARTESIAN_POINT('Ctrl Pts',(-0.571381772416905,-0.641516556204871,
-0.248900000333835));
#32879=CARTESIAN_POINT('Ctrl Pts',(-0.201901977286727,-0.835018653129937,
-0.238466037731354));
#32880=CARTESIAN_POINT('Ctrl Pts',(0.215168005139201,-0.831699114674314,
-0.228032075128873));
#32881=CARTESIAN_POINT('Ctrl Pts',(0.581520879277012,-0.632340059072374,
-0.217598112526393));
#32882=CARTESIAN_POINT('Ctrl Pts',(0.810803789707567,-0.283932934675704,
-0.207164149923912));
#32883=CARTESIAN_POINT('Ctrl Pts',(0.848972675949112,0.131400691338025,
-0.196730187321432));
#32884=CARTESIAN_POINT('Ctrl Pts',(0.687030621675961,0.515760288909193,
-0.186296224718951));
#32885=CARTESIAN_POINT('Ctrl Pts',(0.363149188196709,0.778553580855519,
-0.17586226211647));
#32886=CARTESIAN_POINT('Ctrl Pts',(-0.0463303092822819,0.85782810261103,
-0.16542829951399));
#32887=CARTESIAN_POINT('Ctrl Pts',(-0.444888556851272,0.734917001280118,
-0.154994336911509));
#32888=CARTESIAN_POINT('Ctrl Pts',(-0.738583893176416,0.438754413204515,
-0.144560374309029));
#32889=CARTESIAN_POINT('Ctrl Pts',(-0.858185002917792,0.0392220405825488,
-0.134126411706548));
#32890=CARTESIAN_POINT('Ctrl Pts',(-0.775511018752148,-0.369654877107235,
-0.123692449104067));
#32891=CARTESIAN_POINT('Ctrl Pts',(-0.598512098358569,-0.583991704355496,
-0.116736474035747));
#32892=CARTESIAN_POINT('Ctrl Pts',(-0.489957628934667,-0.66408276156614,
-0.113258486501587));
#32893=CARTESIAN_POINT('Ctrl Pts',(0.82035433218061,-3.00304598431118E-15,
-1.14076763757253));
#32894=CARTESIAN_POINT('Ctrl Pts',(0.82035433218061,0.134101768298553,-1.13728965003837));
#32895=CARTESIAN_POINT('Ctrl Pts',(0.75336476651959,0.402173049067151,-1.13033367497005));
#32896=CARTESIAN_POINT('Ctrl Pts',(0.475095200548896,0.709610076749492,
-1.11989971236757));
#32897=CARTESIAN_POINT('Ctrl Pts',(0.0849252644561683,0.849729327752103,
-1.10946574976509));
#32898=CARTESIAN_POINT('Ctrl Pts',(-0.325303245075438,0.789587177339035,
-1.09903178716261));
#32899=CARTESIAN_POINT('Ctrl Pts',(-0.658834080958526,0.543317828833921,
-1.08859782456013));
#32900=CARTESIAN_POINT('Ctrl Pts',(-0.83708201976552,0.168990519247407,
-1.07816386195765));
#32901=CARTESIAN_POINT('Ctrl Pts',(-0.818016521001051,-0.24517308681731,
-1.06772989935517));
#32902=CARTESIAN_POINT('Ctrl Pts',(-0.60613955422243,-0.6015452379551,-1.05729593675269));
#32903=CARTESIAN_POINT('Ctrl Pts',(-0.251388414543861,-0.816128465044897,
-1.04686197415021));
#32904=CARTESIAN_POINT('Ctrl Pts',(0.162616634294624,-0.838342060921672,
-1.03642801154773));
#32905=CARTESIAN_POINT('Ctrl Pts',(0.538291771678319,-0.662950796574503,
-1.02599404894524));
#32906=CARTESIAN_POINT('Ctrl Pts',(0.787086296167865,-0.331295673135838,
-1.01556008634276));
#32907=CARTESIAN_POINT('Ctrl Pts',(0.850357274403784,0.0784488915092827,
-1.00512612374028));
#32908=CARTESIAN_POINT('Ctrl Pts',(0.713191002178239,0.469702347171163,
-0.994692161137803));
#32909=CARTESIAN_POINT('Ctrl Pts',(0.407918930452032,0.750242527821311,
-0.984258198535323));
#32910=CARTESIAN_POINT('Ctrl Pts',(0.00649651999368601,0.853943500409919,
-0.973824235932842));
#32911=CARTESIAN_POINT('Ctrl Pts',(-0.396457175080163,0.756361958283295,
-0.963390273330361));
#32912=CARTESIAN_POINT('Ctrl Pts',(-0.705962190288662,0.480498794630969,
-0.952956310727882));
#32913=CARTESIAN_POINT('Ctrl Pts',(-0.849065279296998,0.091377547096046,
-0.942522348125399));
#32914=CARTESIAN_POINT('Ctrl Pts',(-0.792035701226649,-0.319282246717188,
-0.93208838552292));
#32915=CARTESIAN_POINT('Ctrl Pts',(-0.548315862494257,-0.654684213877513,
-0.92165442292044));
#32916=CARTESIAN_POINT('Ctrl Pts',(-0.175352820786369,-0.835770957377394,
-0.911220460317958));
#32917=CARTESIAN_POINT('Ctrl Pts',(0.238942529278509,-0.819858629701545,
-0.900786497715479));
#32918=CARTESIAN_POINT('Ctrl Pts',(0.596916878978052,-0.610697915954459,
-0.890352535112996));
#32919=CARTESIAN_POINT('Ctrl Pts',(0.814192309062806,-0.257589962620873,
-0.879918572510518));
#32920=CARTESIAN_POINT('Ctrl Pts',(0.83955495813993,0.156234366365254,-0.869484609908036));
#32921=CARTESIAN_POINT('Ctrl Pts',(0.667026611423941,0.53323278652594,-0.859050647305556));
#32922=CARTESIAN_POINT('Ctrl Pts',(0.337273822063288,0.784543226294379,
-0.848616684703075));
#32923=CARTESIAN_POINT('Ctrl Pts',(-0.0719775776704071,0.850929452590405,
-0.838182722100595));
#32924=CARTESIAN_POINT('Ctrl Pts',(-0.464263185728891,0.716743607819753,
-0.827748759498114));
#32925=CARTESIAN_POINT('Ctrl Pts',(-0.747117596643004,0.413614556996799,
-0.817314796895633));
#32926=CARTESIAN_POINT('Ctrl Pts',(-0.853869366811587,0.0129926669405188,
-0.806880834293152));
#32927=CARTESIAN_POINT('Ctrl Pts',(-0.759356100494368,-0.390691716850215,
-0.796446871690672));
#32928=CARTESIAN_POINT('Ctrl Pts',(-0.485855463026629,-0.70228639031422,
-0.786012909088191));
#32929=CARTESIAN_POINT('Ctrl Pts',(-0.0978341256794825,-0.848345559796203,
-0.775578946485711));
#32930=CARTESIAN_POINT('Ctrl Pts',(0.313247634771888,-0.794441706032111,
-0.765144983883231));
#32931=CARTESIAN_POINT('Ctrl Pts',(0.650493983049113,-0.55328047407287,
-0.754711021280748));
#32932=CARTESIAN_POINT('Ctrl Pts',(0.834412784606905,-0.181705833307426,
-0.74427705867827));
#32933=CARTESIAN_POINT('Ctrl Pts',(0.821652649004654,0.232698580479195,
-0.733843096075788));
#32934=CARTESIAN_POINT('Ctrl Pts',(0.615221260154403,0.592253751383161,
-0.723409133473309));
#32935=CARTESIAN_POINT('Ctrl Pts',(0.263776436949313,0.812209145653827,
-0.712975170870827));
#32936=CARTESIAN_POINT('Ctrl Pts',(-0.149842972053255,0.84071920918916,
-0.702541208268347));
#32937=CARTESIAN_POINT('Ctrl Pts',(-0.528142983956435,0.671063852007383,
-0.692107245665866));
#32938=CARTESIAN_POINT('Ctrl Pts',(-0.781954729776755,0.343232436627368,
-0.681673283063385));
#32939=CARTESIAN_POINT('Ctrl Pts',(-0.851452395088087,-0.0655020905937811,
-0.671239320460905));
#32940=CARTESIAN_POINT('Ctrl Pts',(-0.720254726869516,-0.458797159315003,
-0.660805357858424));
#32941=CARTESIAN_POINT('Ctrl Pts',(-0.419286248832958,-0.743949424701023,
-0.650371395255944));
#32942=CARTESIAN_POINT('Ctrl Pts',(-0.0194880604808538,-0.85374581725013,
-0.639937432653463));
#32943=CARTESIAN_POINT('Ctrl Pts',(0.384903646922485,-0.762306295106611,
-0.629503470050983));
#32944=CARTESIAN_POINT('Ctrl Pts',(0.698569946491375,-0.491184013209342,
-0.619069507448501));
#32945=CARTESIAN_POINT('Ctrl Pts',(0.847576742823385,-0.10428504206404,
-0.608635544846022));
#32946=CARTESIAN_POINT('Ctrl Pts',(0.796801733297027,0.307194893818648,
-0.59820158224354));
#32947=CARTESIAN_POINT('Ctrl Pts',(0.558213064963931,0.646266105468152,
-0.58776761964106));
#32948=CARTESIAN_POINT('Ctrl Pts',(0.188048329783199,0.83300632088787,-0.577333657038579));
#32949=CARTESIAN_POINT('Ctrl Pts',(-0.226441164460161,0.823399115867465,
-0.566899694436099));
#32950=CARTESIAN_POINT('Ctrl Pts',(-0.587556347598871,0.61970899894198,
-0.556465731833618));
#32951=CARTESIAN_POINT('Ctrl Pts',(-0.810178976333798,0.269947645442809,
-0.546031769231138));
#32952=CARTESIAN_POINT('Ctrl Pts',(-0.841834804326556,-0.143442905707693,
-0.535597806628657));
#32953=CARTESIAN_POINT('Ctrl Pts',(-0.675062255341265,-0.523022615559749,
-0.525163844026176));
#32954=CARTESIAN_POINT('Ctrl Pts',(-0.349171186905277,-0.779320978293641,
-0.514729881423695));
#32955=CARTESIAN_POINT('Ctrl Pts',(0.0590228126390761,-0.851926060501479,
-0.504295918821215));
#32956=CARTESIAN_POINT('Ctrl Pts',(0.453304580405342,-0.723724161788821,
-0.493861956218735));
#32957=CARTESIAN_POINT('Ctrl Pts',(0.740738197317945,-0.424933674833568,
-0.483427993616254));
#32958=CARTESIAN_POINT('Ctrl Pts',(0.853572857874703,-0.0259823261662502,
-0.472994031013773));
#32959=CARTESIAN_POINT('Ctrl Pts',(0.765212371889514,0.379093301023122,
-0.462560068411293));
#32960=CARTESIAN_POINT('Ctrl Pts',(0.496484136534512,0.694813073526274,
-0.452126105808812));
#32961=CARTESIAN_POINT('Ctrl Pts',(0.110729923040362,0.846758873066443,
-0.441692143206332));
#32962=CARTESIAN_POINT('Ctrl Pts',(-0.301124374221852,0.799115646338571,
-0.431258180603851));
#32963=CARTESIAN_POINT('Ctrl Pts',(-0.642000825785283,0.563113349747737,
-0.42082421800137));
#32964=CARTESIAN_POINT('Ctrl Pts',(-0.831551647635552,0.194379943122157,
-0.410390255398891));
#32965=CARTESIAN_POINT('Ctrl Pts',(-0.825097929205883,-0.220170643352121,
-0.399956292796408));
#32966=CARTESIAN_POINT('Ctrl Pts',(-0.624160872597553,-0.582824939487969,
-0.389522330193929));
#32967=CARTESIAN_POINT('Ctrl Pts',(-0.276103230945767,-0.808101918597743,
-0.379088367591447));
#32968=CARTESIAN_POINT('Ctrl Pts',(0.137034537726095,-0.842901678981727,
-0.368654404988968));
#32969=CARTESIAN_POINT('Ctrl Pts',(0.517871977672865,-0.679021590036208,
-0.358220442386487));
#32970=CARTESIAN_POINT('Ctrl Pts',(0.776642124271996,-0.355089729166509,
-0.347786479784006));
#32971=CARTESIAN_POINT('Ctrl Pts',(0.852350421415523,0.0525401187286379,
-0.337352517181526));
#32972=CARTESIAN_POINT('Ctrl Pts',(0.727151711791375,0.447785766997164,
-0.326918554579045));
#32973=CARTESIAN_POINT('Ctrl Pts',(0.430556508150092,0.737484100106964,
-0.316484591976565));
#32974=CARTESIAN_POINT('Ctrl Pts',(0.0324750881634892,0.853350499154803,
-0.306050629374083));
#32975=CARTESIAN_POINT('Ctrl Pts',(-0.373261015454173,0.768074161753151,
-0.295616666771603));
#32976=CARTESIAN_POINT('Ctrl Pts',(-0.691015988779456,0.501755528036834,
-0.285182704169122));
#32977=CARTESIAN_POINT('Ctrl Pts',(-0.8458919979872,0.117168392128866,-0.274748741566642));
#32978=CARTESIAN_POINT('Ctrl Pts',(-0.801383310988866,-0.295036420454529,
-0.264314778964161));
#32979=CARTESIAN_POINT('Ctrl Pts',(-0.567981045319896,-0.637698404316481,
-0.253880816361681));
#32980=CARTESIAN_POINT('Ctrl Pts',(-0.200700305914004,-0.830048822575997,
-0.2434468537592));
#32981=CARTESIAN_POINT('Ctrl Pts',(0.213887378143144,-0.826749042700629,
-0.23301289115672));
#32982=CARTESIAN_POINT('Ctrl Pts',(0.578059804635798,-0.628576521295641,
-0.222578928554239));
#32983=CARTESIAN_POINT('Ctrl Pts',(0.805978085266885,-0.282243037988439,
-0.212144965951758));
#32984=CARTESIAN_POINT('Ctrl Pts',(0.843919785925288,0.130618633522326,
-0.201711003349278));
#32985=CARTESIAN_POINT('Ctrl Pts',(0.682941598426257,0.512690593115557,
-0.191277040746797));
#32986=CARTESIAN_POINT('Ctrl Pts',(0.360987776933422,0.773919846182338,
-0.180843078144316));
#32987=CARTESIAN_POINT('Ctrl Pts',(-0.0460544942459823,0.852722459491376,
-0.170409115541836));
#32988=CARTESIAN_POINT('Ctrl Pts',(-0.442240821284995,0.73054306366155,
-0.159975152939355));
#32989=CARTESIAN_POINT('Ctrl Pts',(-0.734187755498598,0.436142832866621,
-0.149541190336875));
#32990=CARTESIAN_POINT('Ctrl Pts',(-0.853077819122258,0.038989038595815,
-0.139107227734394));
#32991=CARTESIAN_POINT('Ctrl Pts',(-0.770894241208365,-0.367455713931438,
-0.128673265131913));
#32992=CARTESIAN_POINT('Ctrl Pts',(-0.594951669076762,-0.580514449476557,
-0.121717290063593));
#32993=CARTESIAN_POINT('Ctrl Pts',(-0.48704143763805,-0.660130190455607,
-0.118239302529433));
#32994=CARTESIAN_POINT('Ctrl Pts',(0.816972063808647,-2.99066461804804E-15,
-1.1425283350431));
#32995=CARTESIAN_POINT('Ctrl Pts',(0.816972063808648,0.133547259366551,
-1.13905034750894));
#32996=CARTESIAN_POINT('Ctrl Pts',(0.750258545288663,0.400515882139597,
-1.13209437244062));
#32997=CARTESIAN_POINT('Ctrl Pts',(0.473136385937636,0.70668384175515,-1.12166040983814));
#32998=CARTESIAN_POINT('Ctrl Pts',(0.0845750992767496,0.846226087845691,
-1.11122644723566));
#32999=CARTESIAN_POINT('Ctrl Pts',(-0.323961995775536,0.786331547179378,
-1.10079248463318));
#33000=CARTESIAN_POINT('Ctrl Pts',(-0.656117677249231,0.541077762637851,
-1.0903585220307));
#33001=CARTESIAN_POINT('Ctrl Pts',(-0.833630685095572,0.168293731192072,
-1.07992455942822));
#33002=CARTESIAN_POINT('Ctrl Pts',(-0.814643797129343,-0.244162209445383,
-1.06949059682573));
#33003=CARTESIAN_POINT('Ctrl Pts',(-0.603640408739919,-0.59906504366349,
-1.05905663422325));
#33004=CARTESIAN_POINT('Ctrl Pts',(-0.250351927233723,-0.812763520669616,
-1.04862267162077));
#33005=CARTESIAN_POINT('Ctrl Pts',(0.161946157548482,-0.83488553496122,
-1.03818870901829));
#33006=CARTESIAN_POINT('Ctrl Pts',(0.536072366553592,-0.660217414778481,
-1.02775474641581));
#33007=CARTESIAN_POINT('Ctrl Pts',(0.783841098330601,-0.329929724332764,
-1.01732078381333));
#33008=CARTESIAN_POINT('Ctrl Pts',(0.846851206973997,0.0781254429130721,
-1.00688682121085));
#33009=CARTESIAN_POINT('Ctrl Pts',(0.710250478470445,0.467765739743977,
-0.99645285860837));
#33010=CARTESIAN_POINT('Ctrl Pts',(0.406237059412559,0.747149238803469,
-0.98601889600589));
#33011=CARTESIAN_POINT('Ctrl Pts',(0.00646973450489124,0.850422646762807,
-0.975584933403409));
#33012=CARTESIAN_POINT('Ctrl Pts',(-0.394822561461415,0.753243438481206,
-0.965150970800928));
#33013=CARTESIAN_POINT('Ctrl Pts',(-0.70305147134073,0.478517673019022,
-0.954717008198448));
#33014=CARTESIAN_POINT('Ctrl Pts',(-0.845564538846855,0.0910007927061355,
-0.944283045595966));
#33015=CARTESIAN_POINT('Ctrl Pts',(-0.788770096702248,-0.317965829356403,
-0.933849082993488));
#33016=CARTESIAN_POINT('Ctrl Pts',(-0.546055127582366,-0.651984916701293,
-0.923415120391005));
#33017=CARTESIAN_POINT('Ctrl Pts',(-0.174629831956392,-0.832325030110572,
-0.912981157788527));
#33018=CARTESIAN_POINT('Ctrl Pts',(0.237957356762351,-0.816478309791072,
-0.902547195186044));
#33019=CARTESIAN_POINT('Ctrl Pts',(0.594455759539154,-0.608179976581174,
-0.892113232583563));
#33020=CARTESIAN_POINT('Ctrl Pts',(0.810835351688311,-0.256527905763963,
-0.881679269981084));
#33021=CARTESIAN_POINT('Ctrl Pts',(0.836093429239885,0.155590203920442,
-0.871245307378603));
#33022=CARTESIAN_POINT('Ctrl Pts',(0.664276425899861,0.531034239923244,
-0.860811344776122));
#33023=CARTESIAN_POINT('Ctrl Pts',(0.335883224496111,0.78130851363521,-0.850377382173643));
#33024=CARTESIAN_POINT('Ctrl Pts',(-0.0716808103619117,0.847421026056225,
-0.83994341957116));
#33025=CARTESIAN_POINT('Ctrl Pts',(-0.462349004389065,0.71378843652532,
-0.829509456968681));
#33026=CARTESIAN_POINT('Ctrl Pts',(-0.744037191807753,0.411909202596062,
-0.819075494366199));
#33027=CARTESIAN_POINT('Ctrl Pts',(-0.850348818857665,0.0129390974967706,
-0.808641531763719));
#33028=CARTESIAN_POINT('Ctrl Pts',(-0.756225235669137,-0.389080874515506,
-0.798207569161239));
#33029=CARTESIAN_POINT('Ctrl Pts',(-0.483852255600829,-0.699390826881936,
-0.787773606558758));
#33030=CARTESIAN_POINT('Ctrl Pts',(-0.0974307504743614,-0.844847786786836,
-0.777339643956278));
#33031=CARTESIAN_POINT('Ctrl Pts',(0.31195609842859,-0.791166181424495,
-0.766905681353797));
#33032=CARTESIAN_POINT('Ctrl Pts',(0.647811962414489,-0.550999269808316,
-0.756471718751317));
#33033=CARTESIAN_POINT('Ctrl Pts',(0.830972457156651,-0.180956650675363,
-0.746037756148836));
#33034=CARTESIAN_POINT('Ctrl Pts',(0.818264932259306,0.231739152089763,
-0.735603793546355));
#33035=CARTESIAN_POINT('Ctrl Pts',(0.61268467079679,0.589811858262647,-0.725169830943875));
#33036=CARTESIAN_POINT('Ctrl Pts',(0.262688872936024,0.808860364965553,
-0.714735868341393));
#33037=CARTESIAN_POINT('Ctrl Pts',(-0.149225161660734,0.837252880021286,
-0.704301905738914));
#33038=CARTESIAN_POINT('Ctrl Pts',(-0.525965422875296,0.668297020729717,
-0.693867943136432));
#33039=CARTESIAN_POINT('Ctrl Pts',(-0.778730689623806,0.341817271381425,
-0.683433980533953));
#33040=CARTESIAN_POINT('Ctrl Pts',(-0.847941812434698,-0.0652320220563909,
-0.673000017931471));
#33041=CARTESIAN_POINT('Ctrl Pts',(-0.717285079048034,-0.456905514687298,
-0.662566055328991));
#33042=CARTESIAN_POINT('Ctrl Pts',(-0.417557509750833,-0.740882082404002,
-0.652132092726511));
#33043=CARTESIAN_POINT('Ctrl Pts',(-0.0194077101906125,-0.850225778697497,
-0.64169813012403));
#33044=CARTESIAN_POINT('Ctrl Pts',(0.383316669102108,-0.759163266475053,
-0.631264167521549));
#33045=CARTESIAN_POINT('Ctrl Pts',(0.695689706150894,-0.489158835893097,
-0.620830204919068));
#33046=CARTESIAN_POINT('Ctrl Pts',(0.844082139686513,-0.103855069394059,
-0.610396242316588));
#33047=CARTESIAN_POINT('Ctrl Pts',(0.793516478173853,0.305928313242129,
-0.599962279714107));
#33048=CARTESIAN_POINT('Ctrl Pts',(0.555911523369753,0.643601516593404,
-0.589528317111627));
#33049=CARTESIAN_POINT('Ctrl Pts',(0.187272996707217,0.829571792360918,
-0.579094354509145));
#33050=CARTESIAN_POINT('Ctrl Pts',(-0.225507535723485,0.820004198348112,
-0.568660391906667));
#33051=CARTESIAN_POINT('Ctrl Pts',(-0.585133822119268,0.617153906403178,
-0.558226429304184));
#33052=CARTESIAN_POINT('Ctrl Pts',(-0.806838566139564,0.26883463721489,
-0.547792466701705));
#33053=CARTESIAN_POINT('Ctrl Pts',(-0.838363875501719,-0.142851483122668,
-0.537358504099224));
#33054=CARTESIAN_POINT('Ctrl Pts',(-0.672278938438019,-0.520866166024689,
-0.526924541496743));
#33055=CARTESIAN_POINT('Ctrl Pts',(-0.347731535882056,-0.776107797235484,
-0.516490578894263));
#33056=CARTESIAN_POINT('Ctrl Pts',(0.0587794585027788,-0.848413524900876,
-0.506056616291782));
#33057=CARTESIAN_POINT('Ctrl Pts',(0.451435581967082,-0.720740209306132,
-0.495622653689302));
#33058=CARTESIAN_POINT('Ctrl Pts',(0.737684095078984,-0.423181651119364,
-0.485188691086821));
#33059=CARTESIAN_POINT('Ctrl Pts',(0.8500535324426,-0.0258751996797192,
-0.474754728484341));
#33060=CARTESIAN_POINT('Ctrl Pts',(0.762057361351743,0.377530279562069,
-0.46432076588186));
#33061=CARTESIAN_POINT('Ctrl Pts',(0.494437106533239,0.691948322969061,
-0.453886803279379));
#33062=CARTESIAN_POINT('Ctrl Pts',(0.110273377789823,0.843267642049257,
-0.443452840676899));
#33063=CARTESIAN_POINT('Ctrl Pts',(-0.299882822714386,0.795820850831186,
-0.433018878074418));
#33064=CARTESIAN_POINT('Ctrl Pts',(-0.639353822881232,0.560791604023703,
-0.422584915471937));
#33065=CARTESIAN_POINT('Ctrl Pts',(-0.828123116802314,0.193578504473992,
-0.412150952869457));
#33066=CARTESIAN_POINT('Ctrl Pts',(-0.821696007390509,-0.219262868301153,
-0.401716990266975));
#33067=CARTESIAN_POINT('Ctrl Pts',(-0.621587424751339,-0.580421921850917,
-0.391283027664496));
#33068=CARTESIAN_POINT('Ctrl Pts',(-0.274964842917688,-0.804770072220882,
-0.380849065062014));
#33069=CARTESIAN_POINT('Ctrl Pts',(0.13646953717677,-0.839426351377121,
-0.370415102459534));
#33070=CARTESIAN_POINT('Ctrl Pts',(0.515736764486322,-0.676221948589213,
-0.359981139857054));
#33071=CARTESIAN_POINT('Ctrl Pts',(0.773439988269239,-0.353625675685122,
-0.349547177254573));
#33072=CARTESIAN_POINT('Ctrl Pts',(0.848836136151768,0.052323493078395,
-0.339113214652093));
#33073=CARTESIAN_POINT('Ctrl Pts',(0.724153627343063,0.445939522912988,
-0.328679252049611));
#33074=CARTESIAN_POINT('Ctrl Pts',(0.428781301197021,0.734443414683683,
-0.318245289447132));
#33075=CARTESIAN_POINT('Ctrl Pts',(0.0323411916877329,0.849832090513251,
-0.30781132684465));
#33076=CARTESIAN_POINT('Ctrl Pts',(-0.37172204082515,0.764907351918341,
-0.297377364242171));
#33077=CARTESIAN_POINT('Ctrl Pts',(-0.688166893772679,0.499686763789961,
-0.286943401639689));
#33078=CARTESIAN_POINT('Ctrl Pts',(-0.842404341196427,0.116685300780257,
-0.276509439037209));
#33079=CARTESIAN_POINT('Ctrl Pts',(-0.798079165673276,-0.293819969988382,
-0.266075476434728));
#33080=CARTESIAN_POINT('Ctrl Pts',(-0.56563923004628,-0.635069140343264,
-0.255641513832248));
#33081=CARTESIAN_POINT('Ctrl Pts',(-0.199872807661205,-0.826626488317452,
-0.245207551229767));
#33082=CARTESIAN_POINT('Ctrl Pts',(0.213005508499054,-0.823340312573245,
-0.234773588627286));
#33083=CARTESIAN_POINT('Ctrl Pts',(0.575676435516449,-0.625984868845308,
-0.224339626024806));
#33084=CARTESIAN_POINT('Ctrl Pts',(0.802654992386147,-0.281079332570895,
-0.213905663422325));
#33085=CARTESIAN_POINT('Ctrl Pts',(0.840440266860438,0.130080080884023,
-0.203471700819845));
#33086=CARTESIAN_POINT('Ctrl Pts',(0.680125782303056,0.510576753259704,
-0.193037738217364));
#33087=CARTESIAN_POINT('Ctrl Pts',(0.359499429618306,0.770728914207567,
-0.182603775614884));
#33088=CARTESIAN_POINT('Ctrl Pts',(-0.0458646565737043,0.849206679729667,
-0.172169813012403));
#33089=CARTESIAN_POINT('Ctrl Pts',(-0.440417346097005,0.727530918967195,
-0.161735850409922));
#33090=CARTESIAN_POINT('Ctrl Pts',(-0.731160844709421,0.434344745947389,
-0.151301887807442));
#33091=CARTESIAN_POINT('Ctrl Pts',(-0.849560168473914,0.0388279800983712,
-0.140867925204961));
#33092=CARTESIAN_POINT('Ctrl Pts',(-0.767716584589541,-0.365940025647496,
-0.13043396260248));
#33093=CARTESIAN_POINT('Ctrl Pts',(-0.59249742112771,-0.578121984952217,
-0.12347798753416));
#33094=CARTESIAN_POINT('Ctrl Pts',(-0.485033396983252,-0.657408515958416,
-0.12));
#33095=CARTESIAN_POINT('',(-0.814921455736581,-0.139942643537172,-0.12));
#33096=CARTESIAN_POINT('',(-0.485033396983251,-0.657408515958417,-0.12));
#33097=CARTESIAN_POINT('Ctrl Pts',(-0.81492145573658,-0.139942643537173,
-0.12));
#33098=CARTESIAN_POINT('Ctrl Pts',(-0.797805299826961,-0.239614354303276,
-0.12));
#33099=CARTESIAN_POINT('Ctrl Pts',(-0.761989157288878,-0.335286098400442,
-0.12));
#33100=CARTESIAN_POINT('Ctrl Pts',(-0.676216606680943,-0.475719941382464,
-0.12));
#33101=CARTESIAN_POINT('Ctrl Pts',(-0.636663795100042,-0.525852834710436,
-0.12));
#33102=CARTESIAN_POINT('Ctrl Pts',(-0.553238444854268,-0.608184477072056,
-0.12));
#33103=CARTESIAN_POINT('Ctrl Pts',(-0.516370109403214,-0.63662333474392,
-0.12));
#33104=CARTESIAN_POINT('Ctrl Pts',(-0.485033396983252,-0.657408515958416,
-0.12));
#33105=CARTESIAN_POINT('',(0.826819918308061,8.40321746433153E-9,-1.12624999033503));
#33106=CARTESIAN_POINT('Ctrl Pts',(0.82685,-3.02682447659827E-15,-1.12625));
#33107=CARTESIAN_POINT('Ctrl Pts',(0.82685,0.135161967341268,-1.12277201246584));
#33108=CARTESIAN_POINT('Ctrl Pts',(0.793089927145679,0.270260225604108,
-1.11929402493168));
#33109=CARTESIAN_POINT('Ctrl Pts',(0.729464420950725,0.389454322909825,
-1.11581603739752));
#33110=CARTESIAN_POINT('Ctrl Pts',(0.66583891475577,0.508648420215542,-1.11233804986336));
#33111=CARTESIAN_POINT('Ctrl Pts',(0.572347975220182,0.611938356564135,
-1.1088600623292));
#33112=CARTESIAN_POINT('Ctrl Pts',(0.460059281045226,0.687121564557402,
-1.10538207479504));
#33113=CARTESIAN_POINT('Ctrl Pts',(0.34777058687027,0.762304772550668,-1.10190408726088));
#33114=CARTESIAN_POINT('Ctrl Pts',(0.216684138055947,0.809381252188609,
-1.09842609972672));
#33115=CARTESIAN_POINT('Ctrl Pts',(0.0822281335574654,0.822816371973694,
-1.09494811219256));
#33116=CARTESIAN_POINT('Ctrl Pts',(-0.0522278709410159,0.836251491758778,
-1.0914701246584));
#33117=CARTESIAN_POINT('Ctrl Pts',(-0.190053431123656,0.816045251691006,
-1.08799213712424));
#33118=CARTESIAN_POINT('Ctrl Pts',(-0.31499483556927,0.764572277302742,
-1.08451414959008));
#33119=CARTESIAN_POINT('Ctrl Pts',(-0.439936240014884,0.713099302914477,
-1.08103616205592));
#33120=CARTESIAN_POINT('Ctrl Pts',(-0.551993488723474,0.630359594205718,
-1.07755817452176));
#33121=CARTESIAN_POINT('Ctrl Pts',(-0.637965330037046,0.526107851543765,
-1.0740801869876));
#33122=CARTESIAN_POINT('Ctrl Pts',(-0.723937171350618,0.421856108881812,
-1.07060219945344));
#33123=CARTESIAN_POINT('Ctrl Pts',(-0.783823605269174,0.296092332266663,
-1.06712421191928));
#33124=CARTESIAN_POINT('Ctrl Pts',(-0.810564079439898,0.1636366258683,-1.06364622438512));
#33125=CARTESIAN_POINT('Ctrl Pts',(-0.837304553610622,0.0311809194699361,
-1.06016823685096));
#33126=CARTESIAN_POINT('Ctrl Pts',(-0.830899068033515,-0.107966716711643,
-1.0566902493168));
#33127=CARTESIAN_POINT('Ctrl Pts',(-0.792103889995617,-0.237406190245859,
-1.05321226178264));
#33128=CARTESIAN_POINT('Ctrl Pts',(-0.75330871195772,-0.366845663780076,
-1.04973427424848));
#33129=CARTESIAN_POINT('Ctrl Pts',(-0.682123841459031,-0.48657697466693,
-1.04625628671432));
#33130=CARTESIAN_POINT('Ctrl Pts',(-0.5869380627173,-0.582489677808408,
-1.04277829918015));
#33131=CARTESIAN_POINT('Ctrl Pts',(-0.491752283975569,-0.678402380949886,
-1.03930031164599));
#33132=CARTESIAN_POINT('Ctrl Pts',(-0.372565596990794,-0.750496476345988,
-1.03582232411183));
#33133=CARTESIAN_POINT('Ctrl Pts',(-0.243425062820331,-0.790275105642179,
-1.03234433657767));
#33134=CARTESIAN_POINT('Ctrl Pts',(-0.114284528649868,-0.83005373493837,
-1.02886634904351));
#33135=CARTESIAN_POINT('Ctrl Pts',(0.0248098527062832,-0.837516898134649,
-1.02538836150935));
#33136=CARTESIAN_POINT('Ctrl Pts',(0.157465332643303,-0.811785143597848,
-1.02191037397519));
#33137=CARTESIAN_POINT('Ctrl Pts',(0.290120812580322,-0.786053389061048,
-1.01843238644103));
#33138=CARTESIAN_POINT('Ctrl Pts',(0.416337391098209,-0.727126716791168,
-1.01495439890687));
#33139=CARTESIAN_POINT('Ctrl Pts',(0.52123976058448,-0.641949852425352,
-1.01147641137271));
#33140=CARTESIAN_POINT('Ctrl Pts',(0.626142130070751,-0.556772988059536,
-1.00799842383855));
#33141=CARTESIAN_POINT('Ctrl Pts',(0.709730290525405,-0.445345931597784,
-1.00452043630439));
#33142=CARTESIAN_POINT('Ctrl Pts',(0.762153030458448,-0.320800915734334,
-1.00104244877023));
#33143=CARTESIAN_POINT('Ctrl Pts',(0.814575770391491,-0.196255899870884,
-0.997564461236072));
#33144=CARTESIAN_POINT('Ctrl Pts',(0.835833089802923,-0.0585929246057353,
-0.994086473701912));
#33145=CARTESIAN_POINT('Ctrl Pts',(0.823419690225198,0.0759637968315887,
-0.990608486167752));
#33146=CARTESIAN_POINT('Ctrl Pts',(0.811006290647473,0.210520518268912,
-0.987130498633591));
#33147=CARTESIAN_POINT('Ctrl Pts',(0.764922172080592,0.34197098587841,-0.983652511099432));
#33148=CARTESIAN_POINT('Ctrl Pts',(0.690598576442014,0.454823136345075,
-0.980174523565272));
#33149=CARTESIAN_POINT('Ctrl Pts',(0.616274980803435,0.567675286811741,
-0.976696536031112));
#33150=CARTESIAN_POINT('Ctrl Pts',(0.513711908093158,0.661929120135573,
-0.973218548496951));
#33151=CARTESIAN_POINT('Ctrl Pts',(0.394996892421945,0.726476383047986,
-0.969740560962791));
#33152=CARTESIAN_POINT('Ctrl Pts',(0.276281876750733,0.791023645960399,
-0.96626257342863));
#33153=CARTESIAN_POINT('Ctrl Pts',(0.141414918118584,0.825864338461393,
-0.962784585894471));
#33154=CARTESIAN_POINT('Ctrl Pts',(0.00629072459520486,0.826892319144936,
-0.95930659836031));
#33155=CARTESIAN_POINT('Ctrl Pts',(-0.128833468928174,0.827920299828479,
-0.95582861082615));
#33156=CARTESIAN_POINT('Ctrl Pts',(-0.264214897342785,0.79513556869457,
-0.952350623291989));
#33157=CARTESIAN_POINT('Ctrl Pts',(-0.383898224562581,0.732401961438677,
-0.948872635757829));
#33158=CARTESIAN_POINT('Ctrl Pts',(-0.503581551782376,0.669668354182784,
-0.945394648223669));
#33159=CARTESIAN_POINT('Ctrl Pts',(-0.607566777807355,0.576985870804906,
-0.941916660689509));
#33160=CARTESIAN_POINT('Ctrl Pts',(-0.683598754197441,0.465277577070771,
-0.938438673155349));
#33161=CARTESIAN_POINT('Ctrl Pts',(-0.759630730587527,0.353569283336635,
-0.934960685621189));
#33162=CARTESIAN_POINT('Ctrl Pts',(-0.807709457342717,0.222835179246241,
-0.931482698087028));
#33163=CARTESIAN_POINT('Ctrl Pts',(-0.822168630942393,0.0884828937125682,
-0.928004710552868));
#33164=CARTESIAN_POINT('Ctrl Pts',(-0.83662780454207,-0.0458693918211047,
-0.924526723018708));
#33165=CARTESIAN_POINT('Ctrl Pts',(-0.817467424986232,-0.183839858798057,
-0.921048735484548));
#33166=CARTESIAN_POINT('Ctrl Pts',(-0.766945632855927,-0.309168039331662,
-0.917570747950388));
#33167=CARTESIAN_POINT('Ctrl Pts',(-0.716423840725621,-0.434496219865267,
-0.914092760416228));
#33168=CARTESIAN_POINT('Ctrl Pts',(-0.634540636020849,-0.547182113955525,
-0.910614772882067));
#33169=CARTESIAN_POINT('Ctrl Pts',(-0.530946339389745,-0.633945159267193,
-0.907136785347907));
#33170=CARTESIAN_POINT('Ctrl Pts',(-0.42735204275864,-0.720708204578862,
-0.903658797813747));
#33171=CARTESIAN_POINT('Ctrl Pts',(-0.302046654201204,-0.781548401111942,
-0.900180810279587));
#33172=CARTESIAN_POINT('Ctrl Pts',(-0.169798002666679,-0.809295445778767,
-0.896702822745426));
#33173=CARTESIAN_POINT('Ctrl Pts',(-0.0375493511321535,-0.837042490445593,
-0.893224835211266));
#33174=CARTESIAN_POINT('Ctrl Pts',(0.101642563379461,-0.831696383246165,
-0.889746847677106));
#33175=CARTESIAN_POINT('Ctrl Pts',(0.231373319484613,-0.793887188023754,
-0.886268860142946));
#33176=CARTESIAN_POINT('Ctrl Pts',(0.361104075589764,-0.756077992801343,
-0.882790872608786));
#33177=CARTESIAN_POINT('Ctrl Pts',(0.481373673288452,-0.68580570955595,
-0.879312885074626));
#33178=CARTESIAN_POINT('Ctrl Pts',(0.578007775213605,-0.59135225717159,
-0.875834897540465));
#33179=CARTESIAN_POINT('Ctrl Pts',(0.67464187713876,-0.49689880478723,-0.872356910006305));
#33180=CARTESIAN_POINT('Ctrl Pts',(0.74764048329038,-0.378264183263903,
-0.868878922472145));
#33181=CARTESIAN_POINT('Ctrl Pts',(0.788400364817746,-0.249430040350934,
-0.865400934937985));
#33182=CARTESIAN_POINT('Ctrl Pts',(0.829160246345112,-0.120595897437964,
-0.861922947403825));
#33183=CARTESIAN_POINT('Ctrl Pts',(0.837681403248224,0.0184377668646483,
-0.858444959869665));
#33184=CARTESIAN_POINT('Ctrl Pts',(0.812959577138439,0.151285181729251,
-0.854966972335504));
#33185=CARTESIAN_POINT('Ctrl Pts',(0.788237751028653,0.284132596593853,
-0.851488984801344));
#33186=CARTESIAN_POINT('Ctrl Pts',(0.73027294190597,0.410793762020446,-0.848010997267183));
#33187=CARTESIAN_POINT('Ctrl Pts',(0.645896574970356,0.516341064330821,
-0.844533009733023));
#33188=CARTESIAN_POINT('Ctrl Pts',(0.561520208034741,0.621888366641197,
-0.841055022198863));
#33189=CARTESIAN_POINT('Ctrl Pts',(0.450732283286195,0.706321805835355,
-0.837577034664703));
#33190=CARTESIAN_POINT('Ctrl Pts',(0.326589678383616,0.759690504248876,
-0.834099047130543));
#33191=CARTESIAN_POINT('Ctrl Pts',(0.202447073481038,0.813059202662397,
-0.830621059596383));
#33192=CARTESIAN_POINT('Ctrl Pts',(0.0649497884244267,0.835363160295282,
-0.827143072062222));
#33193=CARTESIAN_POINT('Ctrl Pts',(-0.0696974754768556,0.823973750907556,
-0.823665084528062));
#33194=CARTESIAN_POINT('Ctrl Pts',(-0.204344739378138,0.81258434151983,
-0.820187096993902));
#33195=CARTESIAN_POINT('Ctrl Pts',(-0.336141982124091,0.767501565111493,
-0.816709109459742));
#33196=CARTESIAN_POINT('Ctrl Pts',(-0.449556279182337,0.694038638780559,
-0.813231121925582));
#33197=CARTESIAN_POINT('Ctrl Pts',(-0.562970576240583,0.620575712449625,
-0.809753134391421));
#33198=CARTESIAN_POINT('Ctrl Pts',(-0.658001927611122,0.518732636196093,
-0.806275146857261));
#33199=CARTESIAN_POINT('Ctrl Pts',(-0.723450441867888,0.400512095240222,
-0.802797159323101));
#33200=CARTESIAN_POINT('Ctrl Pts',(-0.788898956124655,0.282291554284351,
-0.799319171788941));
#33201=CARTESIAN_POINT('Ctrl Pts',(-0.824764633267649,0.147693548626141,
-0.795841184254781));
#33202=CARTESIAN_POINT('Ctrl Pts',(-0.826820534669346,0.012581085871065,
-0.79236319672062));
#33203=CARTESIAN_POINT('Ctrl Pts',(-0.828876436071042,-0.122531376884011,
-0.78888520918646));
#33204=CARTESIAN_POINT('Ctrl Pts',(-0.79712256173144,-0.258158296735951,
-0.7854072216523));
#33205=CARTESIAN_POINT('Ctrl Pts',(-0.735301254991326,-0.378315403705378,
-0.78192923411814));
#33206=CARTESIAN_POINT('Ctrl Pts',(-0.673479948251211,-0.498472510674805,
-0.77845124658398));
#33207=CARTESIAN_POINT('Ctrl Pts',(-0.581591209110582,-0.603159804761718,
-0.77497325904982));
#33208=CARTESIAN_POINT('Ctrl Pts',(-0.470464557373384,-0.68003939630587,
-0.771495271515659));
#33209=CARTESIAN_POINT('Ctrl Pts',(-0.359337905636187,-0.756918987850021,
-0.768017283981499));
#33210=CARTESIAN_POINT('Ctrl Pts',(-0.228973341302421,-0.805990876851411,
-0.764539296447338));
#33211=CARTESIAN_POINT('Ctrl Pts',(-0.0947349410194661,-0.821471710543111,
-0.761061308913178));
#33212=CARTESIAN_POINT('Ctrl Pts',(0.0395034592634902,-0.83695254423481,
-0.757583321379018));
#33213=CARTESIAN_POINT('Ctrl Pts',(0.177615695495635,-0.818842322616818,
-0.754105333844858));
#33214=CARTESIAN_POINT('Ctrl Pts',(0.3033245914807,-0.769275420428634,-0.750627346310698));
#33215=CARTESIAN_POINT('Ctrl Pts',(0.429033487465763,-0.719708518240451,
-0.747149358776538));
#33216=CARTESIAN_POINT('Ctrl Pts',(0.542339043203749,-0.638684935482076,
-0.743671371242377));
#33217=CARTESIAN_POINT('Ctrl Pts',(0.62988766639119,-0.535753682209321,
-0.740193383708217));
#33218=CARTESIAN_POINT('Ctrl Pts',(0.717436289578632,-0.432822428936566,
-0.736715396174057));
#33219=CARTESIAN_POINT('Ctrl Pts',(0.779227980215528,-0.307983505149432,
-0.733237408639897));
#33220=CARTESIAN_POINT('Ctrl Pts',(0.807980297126493,-0.175949764785204,
-0.729759421105737));
#33221=CARTESIAN_POINT('Ctrl Pts',(0.836732614037458,-0.0439160244209771,
-0.726281433571577));
#33222=CARTESIAN_POINT('Ctrl Pts',(0.83244555722249,0.0953125325203408,
-0.722803446037417));
#33223=CARTESIAN_POINT('Ctrl Pts',(0.795624376477292,0.225327166199963,
-0.719325458503256));
#33224=CARTESIAN_POINT('Ctrl Pts',(0.758803195732095,0.355341799879584,
-0.715847470969096));
#33225=CARTESIAN_POINT('Ctrl Pts',(0.689447891056669,0.476142510297508,
-0.712369483434936));
#33226=CARTESIAN_POINT('Ctrl Pts',(0.59573231109141,0.573492365942453,-0.708891495900776));
#33227=CARTESIAN_POINT('Ctrl Pts',(0.502016731126151,0.670842221587399,
-0.705413508366616));
#33228=CARTESIAN_POINT('Ctrl Pts',(0.383940875871057,0.744741222459364,
-0.701935520832455));
#33229=CARTESIAN_POINT('Ctrl Pts',(0.255420539849086,0.786480023964873,
-0.698457533298295));
#33230=CARTESIAN_POINT('Ctrl Pts',(0.126900203827114,0.828218825470382,
-0.694979545764135));
#33231=CARTESIAN_POINT('Ctrl Pts',(-0.0120646129617348,0.837797427609435,
-0.691501558229975));
#33232=CARTESIAN_POINT('Ctrl Pts',(-0.145096253695276,0.814086947098516,
-0.688023570695815));
#33233=CARTESIAN_POINT('Ctrl Pts',(-0.278127894428818,0.790376466587597,
-0.684545583161654));
#33234=CARTESIAN_POINT('Ctrl Pts',(-0.405226359107052,0.733376903426706,
-0.681067595627494));
#33235=CARTESIAN_POINT('Ctrl Pts',(-0.511412496278359,0.649805924044189,
-0.677589608093334));
#33236=CARTESIAN_POINT('Ctrl Pts',(-0.617598633449666,0.566234944661672,
-0.674111620559174));
#33237=CARTESIAN_POINT('Ctrl Pts',(-0.702872443114046,0.456092549057529,
-0.670633633025014));
#33238=CARTESIAN_POINT('Ctrl Pts',(-0.757184005997863,0.332359536245936,
-0.667155645490853));
#33239=CARTESIAN_POINT('Ctrl Pts',(-0.81149556888168,0.208626523434343,
-0.663677657956693));
#33240=CARTESIAN_POINT('Ctrl Pts',(-0.834844884984934,0.0713028934153015,
-0.660199670422533));
#33241=CARTESIAN_POINT('Ctrl Pts',(-0.824480127658202,-0.0634271185637466,
-0.656721682888372));
#33242=CARTESIAN_POINT('Ctrl Pts',(-0.814115370331471,-0.198157130542796,
-0.653243695354212));
#33243=CARTESIAN_POINT('Ctrl Pts',(-0.770036539574754,-0.330293524481848,
-0.649765707820052));
#33244=CARTESIAN_POINT('Ctrl Pts',(-0.697438532772425,-0.444263405286585,
-0.646287720285892));
#33245=CARTESIAN_POINT('Ctrl Pts',(-0.624840525970098,-0.55823328609132,
-0.642809732751732));
#33246=CARTESIAN_POINT('Ctrl Pts',(-0.523723343122158,-0.654036653761739,
-0.639331745217572));
#33247=CARTESIAN_POINT('Ctrl Pts',(-0.406004119499086,-0.720382631122071,
-0.635853757683412));
#33248=CARTESIAN_POINT('Ctrl Pts',(-0.288284895876013,-0.786728608482403,
-0.632375770149252));
#33249=CARTESIAN_POINT('Ctrl Pts',(-0.153963631477806,-0.823617195532651,
-0.628897782615091));
#33250=CARTESIAN_POINT('Ctrl Pts',(-0.0188707186517489,-0.82670089890489,
-0.625419795080931));
#33251=CARTESIAN_POINT('Ctrl Pts',(0.116222194174309,-0.829784602277128,
-0.621941807546771));
#33252=CARTESIAN_POINT('Ctrl Pts',(0.252086755428217,-0.799063421971358,
-0.61846382001261));
#33253=CARTESIAN_POINT('Ctrl Pts',(0.372710687974431,-0.738157993482569,
-0.61498583247845));
#33254=CARTESIAN_POINT('Ctrl Pts',(0.493334620520646,-0.677252564993779,
-0.61150784494429));
#33255=CARTESIAN_POINT('Ctrl Pts',(0.598717924359166,-0.58616288832197,
-0.60802985741013));
#33256=CARTESIAN_POINT('Ctrl Pts',(0.676440681809118,-0.47562431000339,
-0.604551869875969));
#33257=CARTESIAN_POINT('Ctrl Pts',(0.754163439259069,-0.365085731684811,
-0.601073882341809));
#33258=CARTESIAN_POINT('Ctrl Pts',(0.804225650320452,-0.235098251719462,
-0.597595894807649));
#33259=CARTESIAN_POINT('Ctrl Pts',(0.820727248116851,-0.100981505589522,
-0.594117907273489));
#33260=CARTESIAN_POINT('Ctrl Pts',(0.837228845913249,0.0331352405404172,
-0.590639919739329));
#33261=CARTESIAN_POINT('Ctrl Pts',(0.820169830444663,0.171381252834947,
-0.587161932205169));
#33262=CARTESIAN_POINT('Ctrl Pts',(0.771560686864994,0.297463588960067,
-0.583683944671009));
#33263=CARTESIAN_POINT('Ctrl Pts',(0.722951543285326,0.423545925085188,
-0.580205957136848));
#33264=CARTESIAN_POINT('Ctrl Pts',(0.642792271594576,0.5374645850409,-0.576727969602688));
#33265=CARTESIAN_POINT('Ctrl Pts',(0.540530018726793,0.625793719309964,
-0.573249982068528));
#33266=CARTESIAN_POINT('Ctrl Pts',(0.43826776585901,0.714122853579028,-0.569771994534367));
#33267=CARTESIAN_POINT('Ctrl Pts',(0.313902531814194,0.776862462161444,
-0.566294007000207));
#33268=CARTESIAN_POINT('Ctrl Pts',(0.182091343967062,0.80661838729653,-0.562816019466047));
#33269=CARTESIAN_POINT('Ctrl Pts',(0.0502801561199304,0.836374312431615,
-0.559338031931886));
#33270=CARTESIAN_POINT('Ctrl Pts',(-0.0889769855295178,0.833146554119371,
-0.555860044397727));
#33271=CARTESIAN_POINT('Ctrl Pts',(-0.219267972300287,0.797315518848032,
-0.552382056863567));
#33272=CARTESIAN_POINT('Ctrl Pts',(-0.349558959071054,0.761484483576693,
-0.548904069329407));
#33273=CARTESIAN_POINT('Ctrl Pts',(-0.470883790963143,0.69305017134626,
-0.545426081795246));
#33274=CARTESIAN_POINT('Ctrl Pts',(-0.56894376628606,0.600077887508629,
-0.541948094261086));
#33275=CARTESIAN_POINT('Ctrl Pts',(-0.667003741608978,0.507105603670996,
-0.538470106726926));
#33276=CARTESIAN_POINT('Ctrl Pts',(-0.741798860362724,0.389595348226163,
-0.534992119192766));
#33277=CARTESIAN_POINT('Ctrl Pts',(-0.784514166249512,0.261396257101012,
-0.531514131658606));
#33278=CARTESIAN_POINT('Ctrl Pts',(-0.8272294721363,0.133197165975861,-0.528036144124446));
#33279=CARTESIAN_POINT('Ctrl Pts',(-0.837864965156129,-0.0056907608296099,
-0.524558156590285));
#33280=CARTESIAN_POINT('Ctrl Pts',(-0.815167202467579,-0.138898928339155,
-0.521080169056125));
#33281=CARTESIAN_POINT('Ctrl Pts',(-0.792469439779029,-0.2721070958487,
-0.517602181521964));
#33282=CARTESIAN_POINT('Ctrl Pts',(-0.7364384213821,-0.399635504062319,
-0.514124193987804));
#33283=CARTESIAN_POINT('Ctrl Pts',(-0.653677666152339,-0.506454330661924,
-0.510646206453644));
#33284=CARTESIAN_POINT('Ctrl Pts',(-0.570916910922577,-0.61327315726153,
-0.507168218919484));
#33285=CARTESIAN_POINT('Ctrl Pts',(-0.461426418859984,-0.699382402247121,
-0.503690231385324));
#33286=CARTESIAN_POINT('Ctrl Pts',(-0.338110159082283,-0.754633686365735,
-0.500212243851163));
#33287=CARTESIAN_POINT('Ctrl Pts',(-0.214793899304584,-0.809884970484349,
-0.496734256317003));
#33288=CARTESIAN_POINT('Ctrl Pts',(-0.0776518718117775,-0.834278293735987,
-0.493256268782843));
#33289=CARTESIAN_POINT('Ctrl Pts',(0.0571530908599799,-0.824938788321738,
-0.489778281248683));
#33290=CARTESIAN_POINT('Ctrl Pts',(0.191958053531737,-0.815599282907488,
-0.486300293714522));
#33291=CARTESIAN_POINT('Ctrl Pts',(0.324425951382446,-0.772526948827351,
-0.482822306180362));
#33292=CARTESIAN_POINT('Ctrl Pts',(0.438944820023654,-0.700798063101624,
-0.479344318646202));
#33293=CARTESIAN_POINT('Ctrl Pts',(0.553463688664857,-0.6290691773759,-0.475866331112042));
#33294=CARTESIAN_POINT('Ctrl Pts',(0.650033528096561,-0.528683740004589,
-0.472388343577882));
#33295=CARTESIAN_POINT('Ctrl Pts',(0.717273128843357,-0.411472646614386,
-0.468910356043722));
#33296=CARTESIAN_POINT('Ctrl Pts',(0.784512729590156,-0.294261553224178,
-0.465432368509562));
#33297=CARTESIAN_POINT('Ctrl Pts',(0.822422091652043,-0.160224803815075,
-0.461954380975402));
#33298=CARTESIAN_POINT('Ctrl Pts',(0.826533418528118,-0.0251592593056256,
-0.458476393441242));
#33299=CARTESIAN_POINT('Ctrl Pts',(0.830644745404194,0.109906285203826,
-0.454998405907081));
#33300=CARTESIAN_POINT('Ctrl Pts',(0.800958037094456,0.246000624813626,
-0.451520418372921));
#33301=CARTESIAN_POINT('Ctrl Pts',(0.740972011706928,0.367084401928998,
-0.44804243083876));
#33302=CARTESIAN_POINT('Ctrl Pts',(0.680985986319401,0.488168179044368,
-0.4445644433046));
#33303=CARTESIAN_POINT('Ctrl Pts',(0.590700643854085,0.594241393665312,
-0.44108645577044));
#33304=CARTESIAN_POINT('Ctrl Pts',(0.480756536280454,0.672802818882485,
-0.43760846823628));
#33305=CARTESIAN_POINT('Ctrl Pts',(0.370812428706824,0.751364244099657,
-0.43413048070212));
#33306=CARTESIAN_POINT('Ctrl Pts',(0.241209556024878,0.802413879913057,
-0.43065249316796));
#33307=CARTESIAN_POINT('Ctrl Pts',(0.107222225940717,0.819935286798217,
-0.427174505633799));
#33308=CARTESIAN_POINT('Ctrl Pts',(-0.026765104143441,0.837456693683376,
-0.423696518099639));
#33309=CARTESIAN_POINT('Ctrl Pts',(-0.165136891629814,0.821449871640294,
-0.420218530565479));
#33310=CARTESIAN_POINT('Ctrl Pts',(-0.291585370986883,0.773801299882005,
-0.416740543031319));
#33311=CARTESIAN_POINT('Ctrl Pts',(-0.418033850343953,0.726152728123715,
-0.413262555497159));
#33312=CARTESIAN_POINT('Ctrl Pts',(-0.532559021571719,0.646862406650216,
-0.409784567962998));
#33313=CARTESIAN_POINT('Ctrl Pts',(-0.621663554948784,0.545275072528494,
-0.406306580428838));
#33314=CARTESIAN_POINT('Ctrl Pts',(-0.710768088325849,0.443687738406773,
-0.402828592894678));
#33315=CARTESIAN_POINT('Ctrl Pts',(-0.774451983852214,0.31980339163683,
-0.399350605360518));
#33316=CARTESIAN_POINT('Ctrl Pts',(-0.805209795112537,0.188222384767201,
-0.395872617826358));
#33317=CARTESIAN_POINT('Ctrl Pts',(-0.835967606372859,0.0566413778975711,
-0.392394630292197));
#33318=CARTESIAN_POINT('Ctrl Pts',(-0.833799333367139,-0.0826362890717455,
-0.388916642758037));
#33319=CARTESIAN_POINT('Ctrl Pts',(-0.798960517260377,-0.213196088453219,
-0.385438655223877));
#33320=CARTESIAN_POINT('Ctrl Pts',(-0.764121701153614,-0.343755887834692,
-0.381960667689717));
#33321=CARTESIAN_POINT('Ctrl Pts',(-0.69661234194581,-0.465597819628322,
-0.378482680155557));
#33322=CARTESIAN_POINT('Ctrl Pts',(-0.604388734927787,-0.564362239491933,
-0.375004692621396));
#33323=CARTESIAN_POINT('Ctrl Pts',(-0.512165127909764,-0.663126659355544,
-0.371526705087236));
#33324=CARTESIAN_POINT('Ctrl Pts',(-0.395227273081522,-0.738813567289136,
-0.368048717553076));
#33325=CARTESIAN_POINT('Ctrl Pts',(-0.267356846266645,-0.782502905444176,
-0.364570730018916));
#33326=CARTESIAN_POINT('Ctrl Pts',(-0.139486419451767,-0.826192243599216,
-0.361092742484755));
#33327=CARTESIAN_POINT('Ctrl Pts',(-0.00068342065025373,-0.837884011975705,
-0.357614754950595));
#33328=CARTESIAN_POINT('Ctrl Pts',(0.132693564325645,-0.816200280725187,
-0.354136767416435));
#33329=CARTESIAN_POINT('Ctrl Pts',(0.266070549301539,-0.794516549474669,
-0.350658779882275));
#33330=CARTESIAN_POINT('Ctrl Pts',(0.394021520451819,-0.739457318597146,
-0.347180792348115));
#33331=CARTESIAN_POINT('Ctrl Pts',(0.501466854431064,-0.657511577224771,
-0.343702804813955));
#33332=CARTESIAN_POINT('Ctrl Pts',(0.608912188410314,-0.575565835852392,
-0.340224817279795));
#33333=CARTESIAN_POINT('Ctrl Pts',(0.695851885218527,-0.466733583985158,
-0.336746829745634));
#33334=CARTESIAN_POINT('Ctrl Pts',(0.752039692950406,-0.343841214072583,
-0.333268842211474));
#33335=CARTESIAN_POINT('Ctrl Pts',(0.808227500682283,-0.22094884416001,
-0.329790854677314));
#33336=CARTESIAN_POINT('Ctrl Pts',(0.833663419337829,-0.0839963562020974,
-0.326312867143154));
#33337=CARTESIAN_POINT('Ctrl Pts',(0.825349706352788,0.0508757554542803,
-0.322834879608993));
#33338=CARTESIAN_POINT('Ctrl Pts',(0.817035993367747,0.185747867110658,
-0.319356892074833));
#33339=CARTESIAN_POINT('Ctrl Pts',(0.77497264874212,0.318539602465501,-0.315878904540673));
#33340=CARTESIAN_POINT('Ctrl Pts',(0.704117035339799,0.433600831232199,
-0.312400917006513));
#33341=CARTESIAN_POINT('Ctrl Pts',(0.633261421937478,0.548662059998898,
-0.308922929472353));
#33342=CARTESIAN_POINT('Ctrl Pts',(0.533613539758462,0.645992782177453,
-0.305444941938192));
#33343=CARTESIAN_POINT('Ctrl Pts',(0.416917360096601,0.714122114932397,
-0.301966954404032));
#33344=CARTESIAN_POINT('Ctrl Pts',(0.300221180434741,0.782251447687341,
-0.298488966869872));
#33345=CARTESIAN_POINT('Ctrl Pts',(0.166476703290036,0.821179391018675,
-0.295010979335712));
#33346=CARTESIAN_POINT('Ctrl Pts',(0.0314463438949348,0.826318103348088,
-0.291532991801552));
#33347=CARTESIAN_POINT('Ctrl Pts',(-0.103584015500168,0.831456815677501,
-0.288055004267391));
#33348=CARTESIAN_POINT('Ctrl Pts',(-0.239900257145666,0.802806297004992,
-0.284577016733231));
#33349=CARTESIAN_POINT('Ctrl Pts',(-0.361436871197806,0.743743146577004,
-0.281099029199071));
#33350=CARTESIAN_POINT('Ctrl Pts',(-0.482973485249941,0.684679996149019,
-0.277621041664911));
#33351=CARTESIAN_POINT('Ctrl Pts',(-0.589730471708718,0.595204213965558,
-0.27414305413075));
#33352=CARTESIAN_POINT('Ctrl Pts',(-0.669126018040221,0.485860939630323,
-0.27066506659659));
#33353=CARTESIAN_POINT('Ctrl Pts',(-0.748521564371728,0.376517665295085,
-0.26718707906243));
#33354=CARTESIAN_POINT('Ctrl Pts',(-0.800555670575959,0.247306898808072,
-0.26370909152827));
#33355=CARTESIAN_POINT('Ctrl Pts',(-0.819095872468406,0.113456740014413,
-0.26023110399411));
#33356=CARTESIAN_POINT('Ctrl Pts',(-0.837636074360853,-0.0203934187792456,
-0.25675311645995));
#33357=CARTESIAN_POINT('Ctrl Pts',(-0.822682371941516,-0.158882969879551,
-0.25327512892579));
#33358=CARTESIAN_POINT('Ctrl Pts',(-0.775997129713515,-0.28569027602439,
-0.249797141391629));
#33359=CARTESIAN_POINT('Ctrl Pts',(-0.729311887485514,-0.412497582169228,
-0.246319153857469));
#33360=CARTESIAN_POINT('Ctrl Pts',(-0.650895105448849,-0.5276226433586,
-0.242841166323309));
#33361=CARTESIAN_POINT('Ctrl Pts',(-0.549988569180364,-0.61749741574404,
-0.239363178789149));
#33362=CARTESIAN_POINT('Ctrl Pts',(-0.449082032911878,-0.70737218812948,
-0.235885191254988));
#33363=CARTESIAN_POINT('Ctrl Pts',(-0.325685742411572,-0.771996671710988,
-0.232407203720828));
#33364=CARTESIAN_POINT('Ctrl Pts',(-0.194342531999381,-0.803754595401515,
-0.228929216186668));
#33365=CARTESIAN_POINT('Ctrl Pts',(-0.062999321587187,-0.835512519092041,
-0.225451228652508));
#33366=CARTESIAN_POINT('Ctrl Pts',(0.0762908087368925,-0.834403882891585,
-0.221973241118347));
#33367=CARTESIAN_POINT('Ctrl Pts',(0.20711186536151,-0.800559289665402,
-0.218495253584187));
#33368=CARTESIAN_POINT('Ctrl Pts',(0.337932921986123,-0.766714696439221,
-0.215017266050027));
#33369=CARTESIAN_POINT('Ctrl Pts',(0.460284904911274,-0.700134146187317,
-0.211539278515867));
#33370=CARTESIAN_POINT('Ctrl Pts',(0.559748052092242,-0.608664578014513,
-0.208061290981707));
#33371=CARTESIAN_POINT('Ctrl Pts',(0.659211199273213,-0.517195009841706,
-0.204583303447547));
#33372=CARTESIAN_POINT('Ctrl Pts',(0.73578551071,-0.400836423747998,-0.201105315913387));
#33373=CARTESIAN_POINT('Ctrl Pts',(0.780446355236759,-0.273302013173154,
-0.197627328379226));
#33374=CARTESIAN_POINT('Ctrl Pts',(0.825107199763518,-0.145767602598309,
-0.194149340845066));
#33375=CARTESIAN_POINT('Ctrl Pts',(0.837854577380248,-0.00705736754232866,
-0.190671353310906));
#33376=CARTESIAN_POINT('Ctrl Pts',(0.817186127412104,0.126480620590223,
-0.187193365776746));
#33377=CARTESIAN_POINT('Ctrl Pts',(0.79651767744396,0.260018608722774,-0.183715378242586));
#33378=CARTESIAN_POINT('Ctrl Pts',(0.742433399890941,0.388384349931897,
-0.180237390708425));
#33379=CARTESIAN_POINT('Ctrl Pts',(0.661307424905583,0.496450160114778,
-0.176759403174265));
#33380=CARTESIAN_POINT('Ctrl Pts',(0.580181449920225,0.604515970297661,
-0.173281415640105));
#33381=CARTESIAN_POINT('Ctrl Pts',(0.472013777502527,0.692281849454302,
-0.169803428105944));
#33382=CARTESIAN_POINT('Ctrl Pts',(0.349552390106817,0.749402561227557,
-0.166325440571784));
#33383=CARTESIAN_POINT('Ctrl Pts',(0.227091002711111,0.80652327300081,-0.162847453037624));
#33384=CARTESIAN_POINT('Ctrl Pts',(0.0903359003373931,0.832998817390679,
-0.159369465503464));
#33385=CARTESIAN_POINT('Ctrl Pts',(-0.0445955159864317,0.825712101000813,
-0.155891477969304));
#33386=CARTESIAN_POINT('Ctrl Pts',(-0.179526932310259,0.818425384610948,
-0.152413490435144));
#33387=CARTESIAN_POINT('Ctrl Pts',(-0.312634662584192,0.777376407441347,
-0.148935502900983));
#33388=CARTESIAN_POINT('Ctrl Pts',(-0.428231669765076,0.707396742051747,
-0.145457515366823));
#33389=CARTESIAN_POINT('Ctrl Pts',(-0.543828676945959,0.637417076662149,
-0.141979527832663));
#33390=CARTESIAN_POINT('Ctrl Pts',(-0.641914961033792,0.538506723052553,
-0.138501540298503));
#33391=CARTESIAN_POINT('Ctrl Pts',(-0.710929916311705,0.422335058963057,
-0.135023552764343));
#33392=CARTESIAN_POINT('Ctrl Pts',(-0.779944871589619,0.30616339487356,
-0.131545565230183));
#33393=CARTESIAN_POINT('Ctrl Pts',(-0.819888498057611,0.172730420304163,
-0.128067577696022));
#33394=CARTESIAN_POINT('Ctrl Pts',(-0.826054786734804,0.0377369297661925,
-0.124589590161862));
#33395=CARTESIAN_POINT('Ctrl Pts',(-0.828767153927046,-0.0216426961432587,
-0.123059726774575));
#33396=CARTESIAN_POINT('Ctrl Pts',(-0.824944083444905,-0.081324259846495,
-0.121529863387287));
#33397=CARTESIAN_POINT('Ctrl Pts',(-0.814862045042685,-0.139933199781797,
-0.12));
#33398=CARTESIAN_POINT('',(0.589301091561375,0.565833523687252,-1.12625));
#33399=CARTESIAN_POINT('Ctrl Pts',(0.589301091561376,0.565833523687252,
-1.12625));
#33400=CARTESIAN_POINT('Ctrl Pts',(0.616667481029594,0.540044898914141,
-1.12625));
#33401=CARTESIAN_POINT('Ctrl Pts',(0.648190221269374,0.505777024736575,
-1.12625));
#33402=CARTESIAN_POINT('Ctrl Pts',(0.716478059012939,0.410513493212782,
-1.12625));
#33403=CARTESIAN_POINT('Ctrl Pts',(0.746976021141474,0.354408470381556,
-1.12625));
#33404=CARTESIAN_POINT('Ctrl Pts',(0.807743006623441,0.201482947924198,
-1.12625));
#33405=CARTESIAN_POINT('Ctrl Pts',(0.82685,0.101130131372722,-1.12625));
#33406=CARTESIAN_POINT('Ctrl Pts',(0.82685,-2.41473507855972E-15,-1.12625));
#33407=CARTESIAN_POINT('Ctrl Pts',(0.589258732516949,0.565791827419059,
-1.12625));
#33408=CARTESIAN_POINT('Ctrl Pts',(0.548574338866325,0.608188043340019,
-1.12472013661271));
#33409=CARTESIAN_POINT('Ctrl Pts',(0.400588145741329,0.732737761006617,
-1.11971228569126));
#33410=CARTESIAN_POINT('Ctrl Pts',(0.0845750992767496,0.846226087845691,
-1.11122644723566));
#33411=CARTESIAN_POINT('Ctrl Pts',(-0.323961995775536,0.786331547179378,
-1.10079248463318));
#33412=CARTESIAN_POINT('Ctrl Pts',(-0.656117677249231,0.541077762637851,
-1.0903585220307));
#33413=CARTESIAN_POINT('Ctrl Pts',(-0.833630685095572,0.168293731192072,
-1.07992455942822));
#33414=CARTESIAN_POINT('Ctrl Pts',(-0.814643797129343,-0.244162209445383,
-1.06949059682573));
#33415=CARTESIAN_POINT('Ctrl Pts',(-0.603640408739919,-0.59906504366349,
-1.05905663422325));
#33416=CARTESIAN_POINT('Ctrl Pts',(-0.250351927233723,-0.812763520669616,
-1.04862267162077));
#33417=CARTESIAN_POINT('Ctrl Pts',(0.161946157548482,-0.83488553496122,
-1.03818870901829));
#33418=CARTESIAN_POINT('Ctrl Pts',(0.536072366553592,-0.660217414778481,
-1.02775474641581));
#33419=CARTESIAN_POINT('Ctrl Pts',(0.783841098330601,-0.329929724332764,
-1.01732078381333));
#33420=CARTESIAN_POINT('Ctrl Pts',(0.846851206973997,0.0781254429130721,
-1.00688682121085));
#33421=CARTESIAN_POINT('Ctrl Pts',(0.710250478470445,0.467765739743977,
-0.99645285860837));
#33422=CARTESIAN_POINT('Ctrl Pts',(0.406237059412559,0.747149238803469,
-0.98601889600589));
#33423=CARTESIAN_POINT('Ctrl Pts',(0.00646973450489124,0.850422646762807,
-0.975584933403409));
#33424=CARTESIAN_POINT('Ctrl Pts',(-0.394822561461415,0.753243438481206,
-0.965150970800928));
#33425=CARTESIAN_POINT('Ctrl Pts',(-0.70305147134073,0.478517673019022,
-0.954717008198448));
#33426=CARTESIAN_POINT('Ctrl Pts',(-0.845564538846855,0.0910007927061355,
-0.944283045595966));
#33427=CARTESIAN_POINT('Ctrl Pts',(-0.788770096702248,-0.317965829356403,
-0.933849082993488));
#33428=CARTESIAN_POINT('Ctrl Pts',(-0.546055127582366,-0.651984916701293,
-0.923415120391005));
#33429=CARTESIAN_POINT('Ctrl Pts',(-0.174629831956392,-0.832325030110572,
-0.912981157788527));
#33430=CARTESIAN_POINT('Ctrl Pts',(0.237957356762351,-0.816478309791072,
-0.902547195186044));
#33431=CARTESIAN_POINT('Ctrl Pts',(0.594455759539154,-0.608179976581174,
-0.892113232583563));
#33432=CARTESIAN_POINT('Ctrl Pts',(0.810835351688311,-0.256527905763963,
-0.881679269981084));
#33433=CARTESIAN_POINT('Ctrl Pts',(0.836093429239885,0.155590203920442,
-0.871245307378603));
#33434=CARTESIAN_POINT('Ctrl Pts',(0.664276425899861,0.531034239923244,
-0.860811344776122));
#33435=CARTESIAN_POINT('Ctrl Pts',(0.335883224496111,0.78130851363521,-0.850377382173643));
#33436=CARTESIAN_POINT('Ctrl Pts',(-0.0716808103619117,0.847421026056225,
-0.83994341957116));
#33437=CARTESIAN_POINT('Ctrl Pts',(-0.462349004389065,0.71378843652532,
-0.829509456968681));
#33438=CARTESIAN_POINT('Ctrl Pts',(-0.744037191807753,0.411909202596062,
-0.819075494366199));
#33439=CARTESIAN_POINT('Ctrl Pts',(-0.850348818857665,0.0129390974967706,
-0.808641531763719));
#33440=CARTESIAN_POINT('Ctrl Pts',(-0.756225235669137,-0.389080874515506,
-0.798207569161239));
#33441=CARTESIAN_POINT('Ctrl Pts',(-0.483852255600829,-0.699390826881936,
-0.787773606558758));
#33442=CARTESIAN_POINT('Ctrl Pts',(-0.0974307504743614,-0.844847786786836,
-0.777339643956278));
#33443=CARTESIAN_POINT('Ctrl Pts',(0.31195609842859,-0.791166181424495,
-0.766905681353797));
#33444=CARTESIAN_POINT('Ctrl Pts',(0.647811962414489,-0.550999269808316,
-0.756471718751317));
#33445=CARTESIAN_POINT('Ctrl Pts',(0.830972457156651,-0.180956650675363,
-0.746037756148836));
#33446=CARTESIAN_POINT('Ctrl Pts',(0.818264932259306,0.231739152089763,
-0.735603793546355));
#33447=CARTESIAN_POINT('Ctrl Pts',(0.61268467079679,0.589811858262647,-0.725169830943875));
#33448=CARTESIAN_POINT('Ctrl Pts',(0.262688872936024,0.808860364965553,
-0.714735868341393));
#33449=CARTESIAN_POINT('Ctrl Pts',(-0.149225161660734,0.837252880021286,
-0.704301905738914));
#33450=CARTESIAN_POINT('Ctrl Pts',(-0.525965422875296,0.668297020729717,
-0.693867943136432));
#33451=CARTESIAN_POINT('Ctrl Pts',(-0.778730689623806,0.341817271381425,
-0.683433980533953));
#33452=CARTESIAN_POINT('Ctrl Pts',(-0.847941812434698,-0.0652320220563909,
-0.673000017931471));
#33453=CARTESIAN_POINT('Ctrl Pts',(-0.717285079048034,-0.456905514687298,
-0.662566055328991));
#33454=CARTESIAN_POINT('Ctrl Pts',(-0.417557509750833,-0.740882082404002,
-0.652132092726511));
#33455=CARTESIAN_POINT('Ctrl Pts',(-0.0194077101906125,-0.850225778697497,
-0.64169813012403));
#33456=CARTESIAN_POINT('Ctrl Pts',(0.383316669102108,-0.759163266475053,
-0.631264167521549));
#33457=CARTESIAN_POINT('Ctrl Pts',(0.695689706150894,-0.489158835893097,
-0.620830204919068));
#33458=CARTESIAN_POINT('Ctrl Pts',(0.844082139686513,-0.103855069394059,
-0.610396242316588));
#33459=CARTESIAN_POINT('Ctrl Pts',(0.793516478173853,0.305928313242129,
-0.599962279714107));
#33460=CARTESIAN_POINT('Ctrl Pts',(0.555911523369753,0.643601516593404,
-0.589528317111627));
#33461=CARTESIAN_POINT('Ctrl Pts',(0.187272996707217,0.829571792360918,
-0.579094354509145));
#33462=CARTESIAN_POINT('Ctrl Pts',(-0.225507535723485,0.820004198348112,
-0.568660391906667));
#33463=CARTESIAN_POINT('Ctrl Pts',(-0.585133822119268,0.617153906403178,
-0.558226429304184));
#33464=CARTESIAN_POINT('Ctrl Pts',(-0.806838566139564,0.26883463721489,
-0.547792466701705));
#33465=CARTESIAN_POINT('Ctrl Pts',(-0.838363875501719,-0.142851483122668,
-0.537358504099224));
#33466=CARTESIAN_POINT('Ctrl Pts',(-0.672278938438019,-0.520866166024689,
-0.526924541496743));
#33467=CARTESIAN_POINT('Ctrl Pts',(-0.347731535882056,-0.776107797235484,
-0.516490578894263));
#33468=CARTESIAN_POINT('Ctrl Pts',(0.0587794585027788,-0.848413524900876,
-0.506056616291782));
#33469=CARTESIAN_POINT('Ctrl Pts',(0.451435581967082,-0.720740209306132,
-0.495622653689302));
#33470=CARTESIAN_POINT('Ctrl Pts',(0.737684095078984,-0.423181651119364,
-0.485188691086821));
#33471=CARTESIAN_POINT('Ctrl Pts',(0.8500535324426,-0.0258751996797192,
-0.474754728484341));
#33472=CARTESIAN_POINT('Ctrl Pts',(0.762057361351743,0.377530279562069,
-0.46432076588186));
#33473=CARTESIAN_POINT('Ctrl Pts',(0.494437106533239,0.691948322969061,
-0.453886803279379));
#33474=CARTESIAN_POINT('Ctrl Pts',(0.110273377789823,0.843267642049257,
-0.443452840676899));
#33475=CARTESIAN_POINT('Ctrl Pts',(-0.299882822714386,0.795820850831186,
-0.433018878074418));
#33476=CARTESIAN_POINT('Ctrl Pts',(-0.639353822881232,0.560791604023703,
-0.422584915471937));
#33477=CARTESIAN_POINT('Ctrl Pts',(-0.828123116802314,0.193578504473992,
-0.412150952869457));
#33478=CARTESIAN_POINT('Ctrl Pts',(-0.821696007390509,-0.219262868301153,
-0.401716990266975));
#33479=CARTESIAN_POINT('Ctrl Pts',(-0.621587424751339,-0.580421921850917,
-0.391283027664496));
#33480=CARTESIAN_POINT('Ctrl Pts',(-0.274964842917688,-0.804770072220882,
-0.380849065062014));
#33481=CARTESIAN_POINT('Ctrl Pts',(0.13646953717677,-0.839426351377121,
-0.370415102459534));
#33482=CARTESIAN_POINT('Ctrl Pts',(0.515736764486322,-0.676221948589213,
-0.359981139857054));
#33483=CARTESIAN_POINT('Ctrl Pts',(0.773439988269239,-0.353625675685122,
-0.349547177254573));
#33484=CARTESIAN_POINT('Ctrl Pts',(0.848836136151768,0.052323493078395,
-0.339113214652093));
#33485=CARTESIAN_POINT('Ctrl Pts',(0.724153627343063,0.445939522912988,
-0.328679252049611));
#33486=CARTESIAN_POINT('Ctrl Pts',(0.428781301197021,0.734443414683683,
-0.318245289447132));
#33487=CARTESIAN_POINT('Ctrl Pts',(0.0323411916877329,0.849832090513251,
-0.30781132684465));
#33488=CARTESIAN_POINT('Ctrl Pts',(-0.37172204082515,0.764907351918341,
-0.297377364242171));
#33489=CARTESIAN_POINT('Ctrl Pts',(-0.688166893772679,0.499686763789961,
-0.286943401639689));
#33490=CARTESIAN_POINT('Ctrl Pts',(-0.842404341196427,0.116685300780257,
-0.276509439037209));
#33491=CARTESIAN_POINT('Ctrl Pts',(-0.798079165673276,-0.293819969988382,
-0.266075476434728));
#33492=CARTESIAN_POINT('Ctrl Pts',(-0.56563923004628,-0.635069140343264,
-0.255641513832248));
#33493=CARTESIAN_POINT('Ctrl Pts',(-0.199872807661205,-0.826626488317452,
-0.245207551229767));
#33494=CARTESIAN_POINT('Ctrl Pts',(0.213005508499054,-0.823340312573245,
-0.234773588627286));
#33495=CARTESIAN_POINT('Ctrl Pts',(0.575676435516449,-0.625984868845308,
-0.224339626024806));
#33496=CARTESIAN_POINT('Ctrl Pts',(0.802654992386147,-0.281079332570895,
-0.213905663422325));
#33497=CARTESIAN_POINT('Ctrl Pts',(0.840440266860438,0.130080080884023,
-0.203471700819845));
#33498=CARTESIAN_POINT('Ctrl Pts',(0.680125782303056,0.510576753259704,
-0.193037738217364));
#33499=CARTESIAN_POINT('Ctrl Pts',(0.359499429618306,0.770728914207567,
-0.182603775614884));
#33500=CARTESIAN_POINT('Ctrl Pts',(-0.0458646565737043,0.849206679729667,
-0.172169813012403));
#33501=CARTESIAN_POINT('Ctrl Pts',(-0.440417346097005,0.727530918967195,
-0.161735850409922));
#33502=CARTESIAN_POINT('Ctrl Pts',(-0.731160844709421,0.434344745947389,
-0.151301887807442));
#33503=CARTESIAN_POINT('Ctrl Pts',(-0.849560168473914,0.0388279800983712,
-0.140867925204961));
#33504=CARTESIAN_POINT('Ctrl Pts',(-0.767716584589541,-0.365940025647496,
-0.13043396260248));
#33505=CARTESIAN_POINT('Ctrl Pts',(-0.59249742112771,-0.578121984952217,
-0.12347798753416));
#33506=CARTESIAN_POINT('Ctrl Pts',(-0.485033396983252,-0.657408515958416,
-0.12));
#33507=CARTESIAN_POINT('Ctrl Pts',(0.546314451000132,0.524558727749236,
-1.15727273924394));
#33508=CARTESIAN_POINT('Ctrl Pts',(0.45933042519086,0.615150357993716,-1.15374460067508));
#33509=CARTESIAN_POINT('Ctrl Pts',(0.239517155169429,0.752140157504836,
-1.14668832353737));
#33510=CARTESIAN_POINT('Ctrl Pts',(-0.148496413265637,0.775239352992086,
-1.1361039078308));
#33511=CARTESIAN_POINT('Ctrl Pts',(-0.50041587773332,0.61042793059028,-1.12551949212423));
#33512=CARTESIAN_POINT('Ctrl Pts',(-0.731074678445066,0.297631408040497,
-1.11493507641766));
#33513=CARTESIAN_POINT('Ctrl Pts',(-0.784486575071109,-0.0873109114175124,
-1.10435066071109));
#33514=CARTESIAN_POINT('Ctrl Pts',(-0.647739858405562,-0.451090008407746,
-1.09376624500451));
#33515=CARTESIAN_POINT('Ctrl Pts',(-0.353965525798943,-0.705517309450159,
-1.08318182929794));
#33516=CARTESIAN_POINT('Ctrl Pts',(0.0256119661671953,-0.788917676587972,
-1.07259741359137));
#33517=CARTESIAN_POINT('Ctrl Pts',(0.398982356900775,-0.68107280850569,
-1.0620129978848));
#33518=CARTESIAN_POINT('Ctrl Pts',(0.675632891112325,-0.408126282767527,
-1.05142858217823));
#33519=CARTESIAN_POINT('Ctrl Pts',(0.788500750688368,-0.036244024752235,
-1.04084416647166));
#33520=CARTESIAN_POINT('Ctrl Pts',(0.710224521156416,0.344424265850668,
-1.03025975076509));
#33521=CARTESIAN_POINT('Ctrl Pts',(0.459779801870052,0.641599200064964,
-1.01967533505852));
#33522=CARTESIAN_POINT('Ctrl Pts',(0.0978778173933265,0.783241287520997,
-1.00909091935195));
#33523=CARTESIAN_POINT('Ctrl Pts',(-0.287751124101883,0.735014472176636,
-0.998506503645377));
#33524=CARTESIAN_POINT('Ctrl Pts',(-0.603625085401646,0.508609617298404,
-0.987922087938806));
#33525=CARTESIAN_POINT('Ctrl Pts',(-0.773171671953705,0.158910506780705,
-0.977337672232235));
#33526=CARTESIAN_POINT('Ctrl Pts',(-0.755290373416536,-0.229310787602247,
-0.966753256525666));
#33527=CARTESIAN_POINT('Ctrl Pts',(-0.554315867123394,-0.561943861908008,
-0.956168840819094));
#33528=CARTESIAN_POINT('Ctrl Pts',(-0.218967255152568,-0.758353694545466,
-0.945584425112523));
#33529=CARTESIAN_POINT('Ctrl Pts',(0.169462156609871,-0.770927728297872,
-0.935000009405953));
#33530=CARTESIAN_POINT('Ctrl Pts',(0.516811513855877,-0.596617837396195,
-0.924415593699381));
#33531=CARTESIAN_POINT('Ctrl Pts',(0.738878357065634,-0.277679236275885,
-0.913831177992811));
#33532=CARTESIAN_POINT('Ctrl Pts',(0.781830502198585,0.108572789396221,
-0.90324676228624));
#33533=CARTESIAN_POINT('Ctrl Pts',(0.635255734092279,0.468505215644773,
-0.892662346579668));
#33534=CARTESIAN_POINT('Ctrl Pts',(0.334685876135463,0.714865266390365,
-0.882077930873099));
#33535=CARTESIAN_POINT('Ctrl Pts',(-0.0470166324849965,0.78793173628669,
-0.871493515166526));
#33536=CARTESIAN_POINT('Ctrl Pts',(-0.417321635893158,0.669992266368472,
-0.860909099459958));
#33537=CARTESIAN_POINT('Ctrl Pts',(-0.686461896723765,0.389637073600391,
-0.850324683753385));
#33538=CARTESIAN_POINT('Ctrl Pts',(-0.789193960383511,0.0148282727314076,
-0.839740268046816));
#33539=CARTESIAN_POINT('Ctrl Pts',(-0.700614103026784,-0.363575113859105,
-0.829155852340243));
#33540=CARTESIAN_POINT('Ctrl Pts',(-0.442195350963467,-0.653842684721737,
-0.818571436633674));
#33541=CARTESIAN_POINT('Ctrl Pts',(-0.0765821114814572,-0.785609422664233,
-0.807987020927103));
#33542=CARTESIAN_POINT('Ctrl Pts',(0.30759572884442,-0.726933182881659,
-0.797402605220531));
#33543=CARTESIAN_POINT('Ctrl Pts',(0.617207958261565,-0.492037926420709,
-0.786818189513962));
#33544=CARTESIAN_POINT('Ctrl Pts',(0.777200137236411,-0.137865628267143,
-0.776233773807389));
#33545=CARTESIAN_POINT('Ctrl Pts',(0.748787869734938,0.249727273071264,
-0.76564935810082));
#33546=CARTESIAN_POINT('Ctrl Pts',(0.538858696398576,0.576782706132405,
-0.755064942394247));
#33547=CARTESIAN_POINT('Ctrl Pts',(0.198302456030384,0.764017748949664,
-0.744480526687679));
#33548=CARTESIAN_POINT('Ctrl Pts',(-0.190325140315885,0.76604394504593,
-0.733896110981106));
#33549=CARTESIAN_POINT('Ctrl Pts',(-0.532815196286454,0.582370115462685,
-0.723311695274537));
#33550=CARTESIAN_POINT('Ctrl Pts',(-0.746143216224096,0.257521427575564,
-0.712727279567965));
#33551=CARTESIAN_POINT('Ctrl Pts',(-0.778595432221924,-0.129754143290103,
-0.702142863861395));
#33552=CARTESIAN_POINT('Ctrl Pts',(-0.622304962251661,-0.48557545112449,
-0.691558448154824));
#33553=CARTESIAN_POINT('Ctrl Pts',(-0.315158855058534,-0.723686313851511,
-0.680974032448253));
#33554=CARTESIAN_POINT('Ctrl Pts',(0.0683862731776844,-0.786365247463709,
-0.670389616741682));
#33555=CARTESIAN_POINT('Ctrl Pts',(0.435353589178261,-0.65841798059242,
-0.659805201035111));
#33556=CARTESIAN_POINT('Ctrl Pts',(0.696784958823666,-0.37086076354192,
-0.649220785328541));
#33557=CARTESIAN_POINT('Ctrl Pts',(0.789305673168616,0.00659841508485431,
-0.638636369621969));
#33558=CARTESIAN_POINT('Ctrl Pts',(0.690487385718299,0.382458043374308,
-0.628051953915399));
#33559=CARTESIAN_POINT('Ctrl Pts',(0.424285064899531,0.665604363327791,
-0.617467538208828));
#33560=CARTESIAN_POINT('Ctrl Pts',(0.0552299665647796,0.787398650983761,
-0.606883122502258));
#33561=CARTESIAN_POINT('Ctrl Pts',(-0.32721366682163,0.71831622633972,-0.596298706795686));
#33562=CARTESIAN_POINT('Ctrl Pts',(-0.630336020111219,0.475103658718963,
-0.585714291089116));
#33563=CARTESIAN_POINT('Ctrl Pts',(-0.780655892709756,0.116719158475916,
-0.575129875382544));
#33564=CARTESIAN_POINT('Ctrl Pts',(-0.74173359420234,-0.269959737756342,
-0.564545459675975));
#33565=CARTESIAN_POINT('Ctrl Pts',(-0.523004447299988,-0.591196526446348,
-0.553961043969403));
#33566=CARTESIAN_POINT('Ctrl Pts',(-0.177491530455713,-0.769118808373767,
-0.543376628262832));
#33567=CARTESIAN_POINT('Ctrl Pts',(0.211047875895698,-0.760595673704307,
-0.532792212556262));
#33568=CARTESIAN_POINT('Ctrl Pts',(0.548426253918519,-0.567693252373757,
-0.522207796849691));
#33569=CARTESIAN_POINT('Ctrl Pts',(0.752858251913652,-0.237173854594718,
-0.511623381143121));
#33570=CARTESIAN_POINT('Ctrl Pts',(0.774786625126501,0.150839882998086,
-0.501038965436549));
#33571=CARTESIAN_POINT('Ctrl Pts',(0.608895621771471,0.502287872206101,
-0.490454549729978));
#33572=CARTESIAN_POINT('Ctrl Pts',(0.295399597411619,0.731974086035049,
-0.479870134023408));
#33573=CARTESIAN_POINT('Ctrl Pts',(-0.0897055208909264,0.784219296051476,
-0.469285718316836));
#33574=CARTESIAN_POINT('Ctrl Pts',(-0.453064735918975,0.646358514947008,
-0.458701302610267));
#33575=CARTESIAN_POINT('Ctrl Pts',(-0.706594568913721,0.351811170884782,
-0.448116886903694));
#33576=CARTESIAN_POINT('Ctrl Pts',(-0.788835756602106,-0.0280202406126237,
-0.437532471197125));
#33577=CARTESIAN_POINT('Ctrl Pts',(-0.679851857001817,-0.401059144402229,
-0.426948055490553));
#33578=CARTESIAN_POINT('Ctrl Pts',(-0.40606212854654,-0.676875566510091,
-0.416363639783983));
#33579=CARTESIAN_POINT('Ctrl Pts',(-0.0338371233843339,-0.788607655212058,
-0.405779224077412));
#33580=CARTESIAN_POINT('Ctrl Pts',(0.346590485190772,-0.709169951669667,
-0.395194808370841));
#33581=CARTESIAN_POINT('Ctrl Pts',(0.642999595336511,-0.45781929315021,
-0.38461039266427));
#33582=CARTESIAN_POINT('Ctrl Pts',(0.783536392737088,-0.0954866798141,-0.374025976957699));
#33583=CARTESIAN_POINT('Ctrl Pts',(0.734132744595485,0.28999327252795,-0.363441561251129));
#33584=CARTESIAN_POINT('Ctrl Pts',(0.506764802819446,0.605174701533931,
-0.352857145544558));
#33585=CARTESIAN_POINT('Ctrl Pts',(0.156549813679539,0.773653113881336,
-0.342272729837987));
#33586=CARTESIAN_POINT('Ctrl Pts',(-0.231615093084909,0.754586929064556,
-0.331688314131416));
#33587=CARTESIAN_POINT('Ctrl Pts',(-0.563633182964224,0.552598063281501,
-0.321103898424845));
#33588=CARTESIAN_POINT('Ctrl Pts',(-0.759018516340419,0.216651511277543,
-0.310519482718275));
#33589=CARTESIAN_POINT('Ctrl Pts',(-0.770406886705711,-0.171814470849813,
-0.299935067011703));
#33590=CARTESIAN_POINT('Ctrl Pts',(-0.595037595541406,-0.51863016343718,
-0.289350651305133));
#33591=CARTESIAN_POINT('Ctrl Pts',(-0.275422660164455,-0.739722476337532,
-0.278766235598562));
#33592=CARTESIAN_POINT('Ctrl Pts',(0.110958659106209,-0.781495462293021,
-0.268181819891991));
#33593=CARTESIAN_POINT('Ctrl Pts',(0.470442038027584,-0.633822758023187,
-0.25759740418542));
#33594=CARTESIAN_POINT('Ctrl Pts',(0.715883472822076,-0.332502328862273,
-0.24701298847885));
#33595=CARTESIAN_POINT('Ctrl Pts',(0.787784607225334,0.0494214101901685,
-0.236428572772279));
#33596=CARTESIAN_POINT('Ctrl Pts',(0.668715255345631,0.419364726111373,
-0.225844157065708));
#33597=CARTESIAN_POINT('Ctrl Pts',(0.387540164029798,0.687647957073736,
-0.215259741359137));
#33598=CARTESIAN_POINT('Ctrl Pts',(0.0124189653017137,0.789235606485634,
-0.204675325652566));
#33599=CARTESIAN_POINT('Ctrl Pts',(-0.36571115764945,0.699500976810335,
-0.194090909945996));
#33600=CARTESIAN_POINT('Ctrl Pts',(-0.655190820886875,0.440197805626221,
-0.183506494239425));
#33601=CARTESIAN_POINT('Ctrl Pts',(-0.785836630350134,0.0741833682121673,
-0.172922078532854));
#33602=CARTESIAN_POINT('Ctrl Pts',(-0.725996588748235,-0.309812190918388,
-0.162337662826283));
#33603=CARTESIAN_POINT('Ctrl Pts',(-0.490140575868305,-0.618708756217194,
-0.151753247119712));
#33604=CARTESIAN_POINT('Ctrl Pts',(-0.135514917188149,-0.777613622822952,
-0.141168831413142));
#33605=CARTESIAN_POINT('Ctrl Pts',(0.252058240770721,-0.748030699511341,
-0.130584415706571));
#33606=CARTESIAN_POINT('Ctrl Pts',(0.469550542503074,-0.607385125337196,
-0.123528138568857));
#33607=CARTESIAN_POINT('Ctrl Pts',(0.555007866453731,-0.51535192480862,
-0.12));
#33608=CARTESIAN_POINT('Ctrl Pts',(0.560643331187213,0.538316993061908,
-1.14693182616263));
#33609=CARTESIAN_POINT('Ctrl Pts',(0.471377865299377,0.631284684590047,
-1.14340368759377));
#33610=CARTESIAN_POINT('Ctrl Pts',(0.245799274584155,0.771867488863268,
-1.13634741045605));
#33611=CARTESIAN_POINT('Ctrl Pts',(-0.152391216542393,0.795572536170745,
-1.12576299474948));
#33612=CARTESIAN_POINT('Ctrl Pts',(-0.513540917978231,0.626438396109293,
-1.11517857904291));
#33613=CARTESIAN_POINT('Ctrl Pts',(-0.750249498836639,0.30543776347905,
-1.10459416333634));
#33614=CARTESIAN_POINT('Ctrl Pts',(-0.80506229684085,-0.0896009251384309,
-1.09400974762977));
#33615=CARTESIAN_POINT('Ctrl Pts',(-0.664728951054492,-0.46292131668127,
-1.0834253319232));
#33616=CARTESIAN_POINT('Ctrl Pts',(-0.363249427405876,-0.724021804395361,
-1.07284091621663));
#33617=CARTESIAN_POINT('Ctrl Pts',(0.0262837236026674,-0.809609618462482,
-1.06225650051006));
#33618=CARTESIAN_POINT('Ctrl Pts',(0.409446971882722,-0.698936166602645,
-1.05167208480349));
#33619=CARTESIAN_POINT('Ctrl Pts',(0.69335356961438,-0.41883072706013,-1.04108766909692));
#33620=CARTESIAN_POINT('Ctrl Pts',(0.809181757319902,-0.0371946426376338,
-1.03050325339035));
#33621=CARTESIAN_POINT('Ctrl Pts',(0.728852478097601,0.353457916763366,
-1.01991883768378));
#33622=CARTESIAN_POINT('Ctrl Pts',(0.47183902834919,0.658427233899741,-1.00933442197721));
#33623=CARTESIAN_POINT('Ctrl Pts',(0.100444982724272,0.803784347558888,
-0.998750006270634));
#33624=CARTESIAN_POINT('Ctrl Pts',(-0.295298336835145,0.754292626522195,
-0.988165590564065));
#33625=CARTESIAN_POINT('Ctrl Pts',(-0.619457124094387,0.521949565115864,
-0.977581174857492));
#33626=CARTESIAN_POINT('Ctrl Pts',(-0.793450623446179,0.163078453661775,
-0.966996759150923));
#33627=CARTESIAN_POINT('Ctrl Pts',(-0.775100329472668,-0.235325211703865,
-0.956412343444351));
#33628=CARTESIAN_POINT('Ctrl Pts',(-0.568854610572828,-0.576682674425972,
-0.945827927737781));
#33629=CARTESIAN_POINT('Ctrl Pts',(-0.224710386344195,-0.778243996199906,
-0.93524351203121));
#33630=CARTESIAN_POINT('Ctrl Pts',(0.173906854958709,-0.791147825041526,
-0.924659096324638));
#33631=CARTESIAN_POINT('Ctrl Pts',(0.530366583189642,-0.612266088131418,
-0.914074680618069));
#33632=CARTESIAN_POINT('Ctrl Pts',(0.75825785440794,-0.284962280866329,
-0.903490264911497));
#33633=CARTESIAN_POINT('Ctrl Pts',(0.802336559785201,0.111420465286886,
-0.892905849204926));
#33634=CARTESIAN_POINT('Ctrl Pts',(0.651917389820589,0.480793294588515,
-0.882321433498356));
#33635=CARTESIAN_POINT('Ctrl Pts',(0.343464105982164,0.733614942027283,
-0.871737017791784));
#33636=CARTESIAN_POINT('Ctrl Pts',(-0.0482497971806109,0.808597818657717,
-0.861152602085213));
#33637=CARTESIAN_POINT('Ctrl Pts',(-0.428267258344188,0.687565001070053,
-0.850568186378644));
#33638=CARTESIAN_POINT('Ctrl Pts',(-0.704466601254543,0.399856578015558,
-0.839983770672072));
#33639=CARTESIAN_POINT('Ctrl Pts',(-0.809893148702622,0.0152171925979075,
-0.829399354965503));
#33640=CARTESIAN_POINT('Ctrl Pts',(-0.718989995374629,-0.373111058288095,
-0.81881493925893));
#33641=CARTESIAN_POINT('Ctrl Pts',(-0.453793367804575,-0.670991843916457,
-0.80823052355236));
#33642=CARTESIAN_POINT('Ctrl Pts',(-0.0785907273946608,-0.806214594778186,
-0.797646107845789));
#33643=CARTESIAN_POINT('Ctrl Pts',(0.315663431129433,-0.745999379030153,
-0.787061692139219));
#33644=CARTESIAN_POINT('Ctrl Pts',(0.633396252142959,-0.504943227538546,
-0.776477276432648));
#33645=CARTESIAN_POINT('Ctrl Pts',(0.797584748383812,-0.141481604497939,
-0.765892860726077));
#33646=CARTESIAN_POINT('Ctrl Pts',(0.768427276401428,0.256277186163867,
-0.755308445019506));
#33647=CARTESIAN_POINT('Ctrl Pts',(0.552992025078289,0.591910715788788,
-0.744724029312936));
#33648=CARTESIAN_POINT('Ctrl Pts',(0.20350358539473,0.784056608923918,-0.734139613606364));
#33649=CARTESIAN_POINT('Ctrl Pts',(-0.195317038529785,0.786135948628314,
-0.723555197899794));
#33650=CARTESIAN_POINT('Ctrl Pts',(-0.546790014443777,0.597644673171574,
-0.712970782193222));
#33651=CARTESIAN_POINT('Ctrl Pts',(-0.765713258217504,0.264275767817858,
-0.702386366486653));
#33652=CARTESIAN_POINT('Ctrl Pts',(-0.799016639535941,-0.133157369343483,
-0.691801950780081));
#33653=CARTESIAN_POINT('Ctrl Pts',(-0.638626941704349,-0.498311252727784,
-0.681217535073511));
#33654=CARTESIAN_POINT('Ctrl Pts',(-0.323424925022022,-0.742667350258704,
-0.670633119366939));
#33655=CARTESIAN_POINT('Ctrl Pts',(0.0701799264720645,-0.806990243550787,
-0.660048703660369));
#33656=CARTESIAN_POINT('Ctrl Pts',(0.446772158478287,-0.675687141859632,
-0.649464287953797));
#33657=CARTESIAN_POINT('Ctrl Pts',(0.715060419362678,-0.380587797921394,
-0.638879872247227));
#33658=CARTESIAN_POINT('Ctrl Pts',(0.810007791520257,0.00677148006419363,
-0.628295456540657));
#33659=CARTESIAN_POINT('Ctrl Pts',(0.708597671841128,0.392489254282354,
-0.617711040834085));
#33660=CARTESIAN_POINT('Ctrl Pts',(0.435413326011759,0.683062010945683,
-0.607126625127515));
#33661=CARTESIAN_POINT('Ctrl Pts',(0.056678552763067,0.808050751452202,
-0.596542209420944));
#33662=CARTESIAN_POINT('Ctrl Pts',(-0.335795913582409,0.73715641466865,
-0.585957793714373));
#33663=CARTESIAN_POINT('Ctrl Pts',(-0.646868640277571,0.487564803376157,
-0.575373378007802));
#33664=CARTESIAN_POINT('Ctrl Pts',(-0.801131142327443,0.119780499493487,
-0.564788962301232));
#33665=CARTESIAN_POINT('Ctrl Pts',(-0.761187979460869,-0.277040313294047,
-0.554204546594661));
#33666=CARTESIAN_POINT('Ctrl Pts',(-0.536721946533173,-0.606702585601401,
-0.54362013088809));
#33667=CARTESIAN_POINT('Ctrl Pts',(-0.182146825349461,-0.78929146028631,
-0.533035715181518));
#33668=CARTESIAN_POINT('Ctrl Pts',(0.216583295509642,-0.780544778582221,
-0.522451299474949));
#33669=CARTESIAN_POINT('Ctrl Pts',(0.562810523032143,-0.58258286142837,
-0.511866883768377));
#33670=CARTESIAN_POINT('Ctrl Pts',(0.772604417642524,-0.243394513301027,
-0.501282468061807));
#33671=CARTESIAN_POINT('Ctrl Pts',(0.795107934038735,0.154796151419974,
-0.490698052355236));
#33672=CARTESIAN_POINT('Ctrl Pts',(0.624865897488743,0.5154620116181,-0.480113636648665));
#33673=CARTESIAN_POINT('Ctrl Pts',(0.303147416329596,0.751172496327223,
-0.469529220942095));
#33674=CARTESIAN_POINT('Ctrl Pts',(-0.0920583410636534,0.804788007556265,
-0.458944805235523));
#33675=CARTESIAN_POINT('Ctrl Pts',(-0.464947837868942,0.663311377353669,
-0.448360389528953));
#33676=CARTESIAN_POINT('Ctrl Pts',(-0.725127318505594,0.36103856750015,
-0.437775973822382));
#33677=CARTESIAN_POINT('Ctrl Pts',(-0.809525549857519,-0.0287551629084119,
-0.427191558115811));
#33678=CARTESIAN_POINT('Ctrl Pts',(-0.697683191659193,-0.411578229917086,
-0.41660714240924));
#33679=CARTESIAN_POINT('Ctrl Pts',(-0.416712433655261,-0.694628838231771,
-0.40602272670267));
#33680=CARTESIAN_POINT('Ctrl Pts',(-0.0347246124228582,-0.809291465763771,
-0.395438310996098));
#33681=CARTESIAN_POINT('Ctrl Pts',(0.355680952278343,-0.727770249082904,
-0.384853895289528));
#33682=CARTESIAN_POINT('Ctrl Pts',(0.659864359109556,-0.469827098887135,
-0.374269479582957));
#33683=CARTESIAN_POINT('Ctrl Pts',(0.804087192872788,-0.0979911297549973,
-0.363685063876386));
#33684=CARTESIAN_POINT('Ctrl Pts',(0.753387772756398,0.297599292924272,
-0.353100648169815));
#33685=CARTESIAN_POINT('Ctrl Pts',(0.520056364353901,0.621047383969216,
-0.342516232463245));
#33686=CARTESIAN_POINT('Ctrl Pts',(0.160655843676399,0.793944692760265,
-0.331931816756674));
#33687=CARTESIAN_POINT('Ctrl Pts',(-0.237689955121337,0.774378434995818,
-0.321347401050103));
#33688=CARTESIAN_POINT('Ctrl Pts',(-0.578416303442498,0.567091751716574,
-0.310762985343532));
#33689=CARTESIAN_POINT('Ctrl Pts',(-0.778926255117066,0.222333904525174,
-0.300178569636962));
#33690=CARTESIAN_POINT('Ctrl Pts',(-0.790613322678069,-0.17632086631987,
-0.28959415393039));
#33691=CARTESIAN_POINT('Ctrl Pts',(-0.610644399274519,-0.532232932794082,
-0.27900973822382));
#33692=CARTESIAN_POINT('Ctrl Pts',(-0.282646518678684,-0.759124113463783,
-0.268425322517249));
#33693=CARTESIAN_POINT('Ctrl Pts',(0.113868912219852,-0.801992732364212,
-0.257840906810678));
#33694=CARTESIAN_POINT('Ctrl Pts',(0.482780916462016,-0.650446829275436,
-0.247256491104107));
#33695=CARTESIAN_POINT('Ctrl Pts',(0.734659854247096,-0.341223288052482,
-0.236672075397537));
#33696=CARTESIAN_POINT('Ctrl Pts',(0.808446830656353,0.0507176480326692,
-0.226087659690966));
#33697=CARTESIAN_POINT('Ctrl Pts',(0.686254496263712,0.43036393527404,-0.215503243984395));
#33698=CARTESIAN_POINT('Ctrl Pts',(0.397704670145094,0.705683769909664,
-0.204918828277824));
#33699=CARTESIAN_POINT('Ctrl Pts',(0.0127446932145117,0.809935887109747,
-0.194334412571253));
#33700=CARTESIAN_POINT('Ctrl Pts',(-0.375303126800996,0.717847673788811,
-0.183749996864682));
#33701=CARTESIAN_POINT('Ctrl Pts',(-0.672375339354173,0.4517434303189,-0.173165581158112));
#33702=CARTESIAN_POINT('Ctrl Pts',(-0.80644776172748,0.0761290692512678,
-0.162581165451541));
#33703=CARTESIAN_POINT('Ctrl Pts',(-0.745038219657612,-0.31793802715801,
-0.15199674974497));
#33704=CARTESIAN_POINT('Ctrl Pts',(-0.50299611277308,-0.63493641342506,
-0.141412334038399));
#33705=CARTESIAN_POINT('Ctrl Pts',(-0.139069238345857,-0.798009078979886,
-0.130827918331829));
#33706=CARTESIAN_POINT('Ctrl Pts',(0.258669291101823,-0.767650246916566,
-0.120243502625257));
#33707=CARTESIAN_POINT('Ctrl Pts',(0.481866038556653,-0.623315783353728,
-0.113187225487544));
#33708=CARTESIAN_POINT('Ctrl Pts',(0.569564759844972,-0.528868711654082,
-0.109659086918687));
#33709=CARTESIAN_POINT('Ctrl Pts',(0.574972211374295,0.552075258374579,
-1.13659091308131));
#33710=CARTESIAN_POINT('Ctrl Pts',(0.483425305407893,0.647419011186379,
-1.13306277451246));
#33711=CARTESIAN_POINT('Ctrl Pts',(0.252081393998882,0.791594820221698,
-1.12600649737474));
#33712=CARTESIAN_POINT('Ctrl Pts',(-0.156286019819149,0.815905719349405,
-1.11542208166817));
#33713=CARTESIAN_POINT('Ctrl Pts',(-0.526665958223143,0.642448861628305,
-1.1048376659616));
#33714=CARTESIAN_POINT('Ctrl Pts',(-0.769424319228211,0.313244118917604,
-1.09425325025503));
#33715=CARTESIAN_POINT('Ctrl Pts',(-0.825638018610591,-0.0918909388593487,
-1.08366883454846));
#33716=CARTESIAN_POINT('Ctrl Pts',(-0.681718043703422,-0.474752624954795,
-1.07308441884189));
#33717=CARTESIAN_POINT('Ctrl Pts',(-0.372533329012808,-0.742526299340564,
-1.06250000313532));
#33718=CARTESIAN_POINT('Ctrl Pts',(0.0269554810381386,-0.830301560336992,
-1.05191558742875));
#33719=CARTESIAN_POINT('Ctrl Pts',(0.41991158686467,-0.716799524699601,
-1.04133117172218));
#33720=CARTESIAN_POINT('Ctrl Pts',(0.711074248116434,-0.429535171352733,
-1.0307467560156));
#33721=CARTESIAN_POINT('Ctrl Pts',(0.829862763951439,-0.0381452605230327,
-1.02016234030904));
#33722=CARTESIAN_POINT('Ctrl Pts',(0.747480435038786,0.362491567676063,
-1.00957792460246));
#33723=CARTESIAN_POINT('Ctrl Pts',(0.483898254828326,0.675255267734519,
-0.998993508895893));
#33724=CARTESIAN_POINT('Ctrl Pts',(0.103012148055218,0.82432740759678,-0.988409093189321));
#33725=CARTESIAN_POINT('Ctrl Pts',(-0.302845549568408,0.773570780867754,
-0.977824677482751));
#33726=CARTESIAN_POINT('Ctrl Pts',(-0.635289162787124,0.535289512933325,
-0.967240261776179));
#33727=CARTESIAN_POINT('Ctrl Pts',(-0.813729574938655,0.167246400542845,
-0.956655846069609));
#33728=CARTESIAN_POINT('Ctrl Pts',(-0.794910285528797,-0.241339635805483,
-0.946071430363039));
#33729=CARTESIAN_POINT('Ctrl Pts',(-0.583393354022263,-0.591421486943936,
-0.935487014656467));
#33730=CARTESIAN_POINT('Ctrl Pts',(-0.230453517535821,-0.798134297854346,
-0.924902598949897));
#33731=CARTESIAN_POINT('Ctrl Pts',(0.178351553307548,-0.811367921785181,
-0.914318183243325));
#33732=CARTESIAN_POINT('Ctrl Pts',(0.543921652523408,-0.627914338866641,
-0.903733767536756));
#33733=CARTESIAN_POINT('Ctrl Pts',(0.777637351750247,-0.292245325456773,
-0.893149351830183));
#33734=CARTESIAN_POINT('Ctrl Pts',(0.822842617371817,0.114268141177552,
-0.882564936123615));
#33735=CARTESIAN_POINT('Ctrl Pts',(0.668579045548899,0.493081373532257,
-0.871980520417042));
#33736=CARTESIAN_POINT('Ctrl Pts',(0.352242335828866,0.7523646176642,-0.861396104710472));
#33737=CARTESIAN_POINT('Ctrl Pts',(-0.049482961876225,0.829263901028744,
-0.8508116890039));
#33738=CARTESIAN_POINT('Ctrl Pts',(-0.439212880795219,0.705137735771634,
-0.840227273297331));
#33739=CARTESIAN_POINT('Ctrl Pts',(-0.72247130578532,0.410076082430724,
-0.829642857590758));
#33740=CARTESIAN_POINT('Ctrl Pts',(-0.830592337021733,0.0156061124644078,
-0.819058441884189));
#33741=CARTESIAN_POINT('Ctrl Pts',(-0.737365887722474,-0.382647002717086,
-0.808474026177617));
#33742=CARTESIAN_POINT('Ctrl Pts',(-0.465391384645683,-0.688141003111176,
-0.797889610471047));
#33743=CARTESIAN_POINT('Ctrl Pts',(-0.0805993433078642,-0.82681976689214,
-0.787305194764476));
#33744=CARTESIAN_POINT('Ctrl Pts',(0.323731133414446,-0.765065575178646,
-0.776720779057905));
#33745=CARTESIAN_POINT('Ctrl Pts',(0.649584546024354,-0.517848528656383,
-0.766136363351335));
#33746=CARTESIAN_POINT('Ctrl Pts',(0.817969359531213,-0.145097580728736,
-0.755551947644764));
#33747=CARTESIAN_POINT('Ctrl Pts',(0.788066683067918,0.262827099256472,
-0.744967531938192));
#33748=CARTESIAN_POINT('Ctrl Pts',(0.567125353758003,0.607038725445171,
-0.734383116231623));
#33749=CARTESIAN_POINT('Ctrl Pts',(0.208704714759077,0.804095468898173,
-0.72379870052505));
#33750=CARTESIAN_POINT('Ctrl Pts',(-0.200308936743686,0.806227952210697,
-0.713214284818482));
#33751=CARTESIAN_POINT('Ctrl Pts',(-0.560764832601099,0.612919230880464,
-0.702629869111908));
#33752=CARTESIAN_POINT('Ctrl Pts',(-0.785283300210913,0.271030108060151,
-0.692045453405339));
#33753=CARTESIAN_POINT('Ctrl Pts',(-0.819437846849956,-0.136560595396861,
-0.681461037698768));
#33754=CARTESIAN_POINT('Ctrl Pts',(-0.654948921157037,-0.511047054331079,
-0.670876621992197));
#33755=CARTESIAN_POINT('Ctrl Pts',(-0.33169099498551,-0.761648386665895,
-0.660292206285627));
#33756=CARTESIAN_POINT('Ctrl Pts',(0.0719735797664441,-0.827615239637866,
-0.649707790579055));
#33757=CARTESIAN_POINT('Ctrl Pts',(0.458190727778314,-0.692956303126841,
-0.639123374872485));
#33758=CARTESIAN_POINT('Ctrl Pts',(0.733335879901689,-0.390314832300869,
-0.628538959165914));
#33759=CARTESIAN_POINT('Ctrl Pts',(0.830709909871898,0.00694454504353371,
-0.617954543459343));
#33760=CARTESIAN_POINT('Ctrl Pts',(0.726707957963956,0.4025204651904,-0.607370127752773));
#33761=CARTESIAN_POINT('Ctrl Pts',(0.446541587123989,0.700519658563575,
-0.596785712046201));
#33762=CARTESIAN_POINT('Ctrl Pts',(0.0581271389613537,0.828702851920643,
-0.586201296339631));
#33763=CARTESIAN_POINT('Ctrl Pts',(-0.344378160343187,0.75599660299758,
-0.575616880633059));
#33764=CARTESIAN_POINT('Ctrl Pts',(-0.663401260443925,0.500025948033351,
-0.56503246492649));
#33765=CARTESIAN_POINT('Ctrl Pts',(-0.82160639194513,0.122841840511059,
-0.554448049219918));
#33766=CARTESIAN_POINT('Ctrl Pts',(-0.780642364719398,-0.284120888831752,
-0.543863633513348));
#33767=CARTESIAN_POINT('Ctrl Pts',(-0.550439445766359,-0.622208644756453,
-0.533279217806777));
#33768=CARTESIAN_POINT('Ctrl Pts',(-0.186802120243209,-0.809464112198856,
-0.522694802100206));
#33769=CARTESIAN_POINT('Ctrl Pts',(0.222118715123586,-0.800493883460134,
-0.512110386393635));
#33770=CARTESIAN_POINT('Ctrl Pts',(0.577194792145768,-0.597472470482985,
-0.501525970687065));
#33771=CARTESIAN_POINT('Ctrl Pts',(0.792350583371396,-0.249615172007336,
-0.490941554980494));
#33772=CARTESIAN_POINT('Ctrl Pts',(0.815429242950967,0.158752419841862,
-0.480357139273923));
#33773=CARTESIAN_POINT('Ctrl Pts',(0.640836173206014,0.528636151030098,
-0.469772723567352));
#33774=CARTESIAN_POINT('Ctrl Pts',(0.310895235247574,0.770370906619397,
-0.459188307860781));
#33775=CARTESIAN_POINT('Ctrl Pts',(-0.0944111612363807,0.825356719061054,
-0.44860389215421));
#33776=CARTESIAN_POINT('Ctrl Pts',(-0.476830939818908,0.68026423976033,
-0.43801947644764));
#33777=CARTESIAN_POINT('Ctrl Pts',(-0.743660068097467,0.370265964115517,
-0.427435060741069));
#33778=CARTESIAN_POINT('Ctrl Pts',(-0.830215343112932,-0.0294900852041995,
-0.416850645034497));
#33779=CARTESIAN_POINT('Ctrl Pts',(-0.71551452631657,-0.422097315431943,
-0.406266229327927));
#33780=CARTESIAN_POINT('Ctrl Pts',(-0.427362738763982,-0.71238210995345,
-0.395681813621356));
#33781=CARTESIAN_POINT('Ctrl Pts',(-0.0356121014613823,-0.829975276315481,
-0.385097397914785));
#33782=CARTESIAN_POINT('Ctrl Pts',(0.364771419365913,-0.746370546496145,
-0.374512982208215));
#33783=CARTESIAN_POINT('Ctrl Pts',(0.676729122882603,-0.481834904624058,
-0.363928566501644));
#33784=CARTESIAN_POINT('Ctrl Pts',(0.824637993008486,-0.100495579695895,
-0.353344150795073));
#33785=CARTESIAN_POINT('Ctrl Pts',(0.772642800917313,0.305205313320593,
-0.342759735088502));
#33786=CARTESIAN_POINT('Ctrl Pts',(0.533347925888355,0.636920066404502,
-0.332175319381931));
#33787=CARTESIAN_POINT('Ctrl Pts',(0.164761873673258,0.814236271639193,
-0.321590903675361));
#33788=CARTESIAN_POINT('Ctrl Pts',(-0.243764817157765,0.794169940927082,
-0.311006487968789));
#33789=CARTESIAN_POINT('Ctrl Pts',(-0.593199423920774,0.581585440151646,
-0.300422072262219));
#33790=CARTESIAN_POINT('Ctrl Pts',(-0.798833993893712,0.228016297772806,
-0.289837656555648));
#33791=CARTESIAN_POINT('Ctrl Pts',(-0.810819758650429,-0.180827261789927,
-0.279253240849077));
#33792=CARTESIAN_POINT('Ctrl Pts',(-0.62625120300763,-0.545835702150984,
-0.268668825142506));
#33793=CARTESIAN_POINT('Ctrl Pts',(-0.289870377192915,-0.778525750590034,
-0.258084409435936));
#33794=CARTESIAN_POINT('Ctrl Pts',(0.116779165333497,-0.822490002435403,
-0.247499993729365));
#33795=CARTESIAN_POINT('Ctrl Pts',(0.495119794896445,-0.667070900527686,
-0.236915578022794));
#33796=CARTESIAN_POINT('Ctrl Pts',(0.753436235672117,-0.34994424724269,
-0.226331162316223));
#33797=CARTESIAN_POINT('Ctrl Pts',(0.82910905408737,0.0520138858751696,
-0.215746746609652));
#33798=CARTESIAN_POINT('Ctrl Pts',(0.703793737181796,0.441363144436706,
-0.205162330903082));
#33799=CARTESIAN_POINT('Ctrl Pts',(0.407869176260388,0.723719582745591,
-0.194577915196511));
#33800=CARTESIAN_POINT('Ctrl Pts',(0.0130704211273114,0.830636167733861,
-0.18399349948994));
#33801=CARTESIAN_POINT('Ctrl Pts',(-0.384895095952544,0.736194370767287,
-0.173409083783369));
#33802=CARTESIAN_POINT('Ctrl Pts',(-0.68955985782147,0.463289055011579,
-0.162824668076798));
#33803=CARTESIAN_POINT('Ctrl Pts',(-0.827058893104828,0.0780747702903682,
-0.152240252370227));
#33804=CARTESIAN_POINT('Ctrl Pts',(-0.764079850566988,-0.326063863397633,
-0.141655836663657));
#33805=CARTESIAN_POINT('Ctrl Pts',(-0.515851649677855,-0.651164070632928,
-0.131071420957086));
#33806=CARTESIAN_POINT('Ctrl Pts',(-0.142623559503565,-0.818404535136818,
-0.120487005250515));
#33807=CARTESIAN_POINT('Ctrl Pts',(0.265280341432924,-0.787269794321791,
-0.109902589543944));
#33808=CARTESIAN_POINT('Ctrl Pts',(0.494181534610232,-0.639246441370259,
-0.10284631240623));
#33809=CARTESIAN_POINT('Ctrl Pts',(0.584121653236212,-0.542385498499545,
-0.0993181738373734));
#33810=CARTESIAN_POINT('Ctrl Pts',(0.589301091561376,0.565833523687251,
-1.12625));
#33811=CARTESIAN_POINT('Ctrl Pts',(0.49547274551641,0.663553337782711,-1.12272186143114));
#33812=CARTESIAN_POINT('Ctrl Pts',(0.258363513413608,0.81132215158013,-1.11566558429343));
#33813=CARTESIAN_POINT('Ctrl Pts',(-0.160180823095904,0.836238902528062,
-1.10508116858686));
#33814=CARTESIAN_POINT('Ctrl Pts',(-0.539790998468055,0.658459327147319,
-1.09449675288029));
#33815=CARTESIAN_POINT('Ctrl Pts',(-0.788599139619784,0.321050474356156,
-1.08391233717372));
#33816=CARTESIAN_POINT('Ctrl Pts',(-0.846213740380332,-0.0941809525802668,
-1.07332792146714));
#33817=CARTESIAN_POINT('Ctrl Pts',(-0.698707136352351,-0.486583933228319,
-1.06274350576058));
#33818=CARTESIAN_POINT('Ctrl Pts',(-0.381817230619741,-0.761030794285767,
-1.052159090054));
#33819=CARTESIAN_POINT('Ctrl Pts',(0.0276272384736108,-0.850993502211501,
-1.04157467434743));
#33820=CARTESIAN_POINT('Ctrl Pts',(0.430376201846617,-0.734662882796558,
-1.03099025864086));
#33821=CARTESIAN_POINT('Ctrl Pts',(0.728794926618489,-0.440239615645336,
-1.02040584293429));
#33822=CARTESIAN_POINT('Ctrl Pts',(0.850543770582973,-0.0390958784084322,
-1.00982142722772));
#33823=CARTESIAN_POINT('Ctrl Pts',(0.766108391979972,0.371525218588761,
-0.99923701152115));
#33824=CARTESIAN_POINT('Ctrl Pts',(0.495957481307464,0.692083301569296,
-0.988652595814578));
#33825=CARTESIAN_POINT('Ctrl Pts',(0.105579313386164,0.844870467634671,
-0.978068180108008));
#33826=CARTESIAN_POINT('Ctrl Pts',(-0.31039276230167,0.792848935213314,
-0.967483764401438));
#33827=CARTESIAN_POINT('Ctrl Pts',(-0.651121201479864,0.548629460750785,
-0.956899348694866));
#33828=CARTESIAN_POINT('Ctrl Pts',(-0.834008526431131,0.171414347423915,
-0.946314932988296));
#33829=CARTESIAN_POINT('Ctrl Pts',(-0.814720241584927,-0.247354059907101,
-0.935730517281725));
#33830=CARTESIAN_POINT('Ctrl Pts',(-0.597932097471697,-0.606160299461901,
-0.925146101575155));
#33831=CARTESIAN_POINT('Ctrl Pts',(-0.236196648727449,-0.818024599508785,
-0.914561685868583));
#33832=CARTESIAN_POINT('Ctrl Pts',(0.182796251656386,-0.831588018528835,
-0.903977270162012));
#33833=CARTESIAN_POINT('Ctrl Pts',(0.557476721857173,-0.643562589601863,
-0.893392854455442));
#33834=CARTESIAN_POINT('Ctrl Pts',(0.797016849092553,-0.299528370047217,
-0.88280843874887));
#33835=CARTESIAN_POINT('Ctrl Pts',(0.843348674958434,0.117115817068219,
-0.8722240230423));
#33836=CARTESIAN_POINT('Ctrl Pts',(0.685240701277208,0.505369452475997,
-0.86163960733573));
#33837=CARTESIAN_POINT('Ctrl Pts',(0.361020565675568,0.771114293301119,
-0.851055191629158));
#33838=CARTESIAN_POINT('Ctrl Pts',(-0.0507161265718393,0.84992998339977,
-0.840470775922587));
#33839=CARTESIAN_POINT('Ctrl Pts',(-0.45015850324625,0.722710470473215,
-0.829886360216017));
#33840=CARTESIAN_POINT('Ctrl Pts',(-0.740476010316097,0.420295586845891,
-0.819301944509446));
#33841=CARTESIAN_POINT('Ctrl Pts',(-0.851291525340844,0.0159950323309077,
-0.808717528802875));
#33842=CARTESIAN_POINT('Ctrl Pts',(-0.755741780070319,-0.392182947146075,
-0.798133113096305));
#33843=CARTESIAN_POINT('Ctrl Pts',(-0.476989401486791,-0.705290162305896,
-0.787548697389733));
#33844=CARTESIAN_POINT('Ctrl Pts',(-0.0826079592210675,-0.847424939006093,
-0.776964281683163));
#33845=CARTESIAN_POINT('Ctrl Pts',(0.33179883569946,-0.78413177132714,-0.766379865976592));
#33846=CARTESIAN_POINT('Ctrl Pts',(0.665772839905748,-0.530753829774219,
-0.755795450270021));
#33847=CARTESIAN_POINT('Ctrl Pts',(0.838353970678615,-0.148713556959532,
-0.74521103456345));
#33848=CARTESIAN_POINT('Ctrl Pts',(0.807706089734408,0.269377012349075,
-0.73462661885688));
#33849=CARTESIAN_POINT('Ctrl Pts',(0.581258682437717,0.622166735101554,
-0.724042203150308));
#33850=CARTESIAN_POINT('Ctrl Pts',(0.213905844123423,0.824134328872426,
-0.713457787443738));
#33851=CARTESIAN_POINT('Ctrl Pts',(-0.205300834957585,0.826319955793079,
-0.702873371737167));
#33852=CARTESIAN_POINT('Ctrl Pts',(-0.574739650758423,0.628193788589353,
-0.692288956030596));
#33853=CARTESIAN_POINT('Ctrl Pts',(-0.804853342204321,0.277784448302445,
-0.681704540324025));
#33854=CARTESIAN_POINT('Ctrl Pts',(-0.839859054163973,-0.13996382145024,
-0.671120124617455));
#33855=CARTESIAN_POINT('Ctrl Pts',(-0.671270900609725,-0.523782855934373,
-0.660535708910883));
#33856=CARTESIAN_POINT('Ctrl Pts',(-0.339957064948998,-0.780629423073089,
-0.649951293204314));
#33857=CARTESIAN_POINT('Ctrl Pts',(0.0737672330608236,-0.848240235724943,
-0.639366877497742));
#33858=CARTESIAN_POINT('Ctrl Pts',(0.469609297078341,-0.710225464394054,
-0.628782461791172));
#33859=CARTESIAN_POINT('Ctrl Pts',(0.751611340440699,-0.400041866680343,
-0.618198046084599));
#33860=CARTESIAN_POINT('Ctrl Pts',(0.85141202822354,0.00711761002287252,
-0.607613630378031));
#33861=CARTESIAN_POINT('Ctrl Pts',(0.744818244086785,0.412551676098446,
-0.597029214671458));
#33862=CARTESIAN_POINT('Ctrl Pts',(0.457669848236219,0.717977306181466,
-0.58644479896489));
#33863=CARTESIAN_POINT('Ctrl Pts',(0.0595757251596406,0.849354952389083,
-0.575860383258316));
#33864=CARTESIAN_POINT('Ctrl Pts',(-0.352960407103966,0.77483679132651,
-0.565275967551747));
#33865=CARTESIAN_POINT('Ctrl Pts',(-0.679933880610278,0.512487092690545,
-0.554691551845175));
#33866=CARTESIAN_POINT('Ctrl Pts',(-0.842081641562816,0.12590318152863,
-0.544107136138606));
#33867=CARTESIAN_POINT('Ctrl Pts',(-0.800096749977928,-0.291201464369457,
-0.533522720432034));
#33868=CARTESIAN_POINT('Ctrl Pts',(-0.564156944999544,-0.637714703911506,
-0.522938304725464));
#33869=CARTESIAN_POINT('Ctrl Pts',(-0.191457415136958,-0.829636764111399,
-0.512353889018893));
#33870=CARTESIAN_POINT('Ctrl Pts',(0.22765413473753,-0.820442988338048,
-0.501769473312322));
#33871=CARTESIAN_POINT('Ctrl Pts',(0.591579061259393,-0.6123620795376,-0.491185057605751));
#33872=CARTESIAN_POINT('Ctrl Pts',(0.812096749100267,-0.255835830713644,
-0.48060064189918));
#33873=CARTESIAN_POINT('Ctrl Pts',(0.835750551863201,0.162708688263749,
-0.47001622619261));
#33874=CARTESIAN_POINT('Ctrl Pts',(0.656806448923285,0.541810290442097,
-0.459431810486038));
#33875=CARTESIAN_POINT('Ctrl Pts',(0.318643054165552,0.789569316911571,
-0.448847394779468));
#33876=CARTESIAN_POINT('Ctrl Pts',(-0.0967639814091079,0.845925430565843,
-0.438262979072897));
#33877=CARTESIAN_POINT('Ctrl Pts',(-0.488714041768874,0.697217102166991,
-0.427678563366326));
#33878=CARTESIAN_POINT('Ctrl Pts',(-0.762192817689339,0.379493360730885,
-0.417094147659756));
#33879=CARTESIAN_POINT('Ctrl Pts',(-0.850905136368346,-0.0302250074999876,
-0.406509731953184));
#33880=CARTESIAN_POINT('Ctrl Pts',(-0.733345860973945,-0.4326164009468,
-0.395925316246614));
#33881=CARTESIAN_POINT('Ctrl Pts',(-0.438013043872703,-0.730135381675129,
-0.385340900540043));
#33882=CARTESIAN_POINT('Ctrl Pts',(-0.0364995904999063,-0.850659086867193,
-0.374756484833472));
#33883=CARTESIAN_POINT('Ctrl Pts',(0.373861886453484,-0.764970843909383,
-0.364172069126902));
#33884=CARTESIAN_POINT('Ctrl Pts',(0.693593886655648,-0.493842710360983,
-0.35358765342033));
#33885=CARTESIAN_POINT('Ctrl Pts',(0.845188793144185,-0.103000029636792,
-0.34300323771376));
#33886=CARTESIAN_POINT('Ctrl Pts',(0.791897829078227,0.312811333716915,
-0.332418822007189));
#33887=CARTESIAN_POINT('Ctrl Pts',(0.54663948742281,0.652792748839787,-0.321834406300618));
#33888=CARTESIAN_POINT('Ctrl Pts',(0.168867903670117,0.834527850518123,
-0.311249990594047));
#33889=CARTESIAN_POINT('Ctrl Pts',(-0.249839679194194,0.813961446858345,
-0.300665574887476));
#33890=CARTESIAN_POINT('Ctrl Pts',(-0.607982544399048,0.596079128586719,
-0.290081159180906));
#33891=CARTESIAN_POINT('Ctrl Pts',(-0.818741732670359,0.233698691020436,
-0.279496743474335));
#33892=CARTESIAN_POINT('Ctrl Pts',(-0.831026194622787,-0.185333657259983,
-0.268912327767764));
#33893=CARTESIAN_POINT('Ctrl Pts',(-0.641858006740743,-0.559438471507887,
-0.258327912061193));
#33894=CARTESIAN_POINT('Ctrl Pts',(-0.297094235707144,-0.797927387716284,
-0.247743496354622));
#33895=CARTESIAN_POINT('Ctrl Pts',(0.119689418447141,-0.842987272506595,
-0.237159080648052));
#33896=CARTESIAN_POINT('Ctrl Pts',(0.507458673330876,-0.683694971779935,
-0.226574664941481));
#33897=CARTESIAN_POINT('Ctrl Pts',(0.772212617097137,-0.358665206432899,
-0.21599024923491));
#33898=CARTESIAN_POINT('Ctrl Pts',(0.849771277518388,0.0533101237176703,
-0.205405833528339));
#33899=CARTESIAN_POINT('Ctrl Pts',(0.721332978099877,0.452362353599373,
-0.194821417821768));
#33900=CARTESIAN_POINT('Ctrl Pts',(0.418033682375684,0.741755395581518,
-0.184237002115198));
#33901=CARTESIAN_POINT('Ctrl Pts',(0.0133961490401099,0.851336448357973,
-0.173652586408627));
#33902=CARTESIAN_POINT('Ctrl Pts',(-0.39448706510409,0.754541067745763,
-0.163068170702056));
#33903=CARTESIAN_POINT('Ctrl Pts',(-0.706744376288768,0.474834679704258,
-0.152483754995485));
#33904=CARTESIAN_POINT('Ctrl Pts',(-0.847670024482173,0.0800204713294688,
-0.141899339288914));
#33905=CARTESIAN_POINT('Ctrl Pts',(-0.783121481476366,-0.334189699637256,
-0.131314923582344));
#33906=CARTESIAN_POINT('Ctrl Pts',(-0.528707186582629,-0.667391727840794,
-0.120730507875773));
#33907=CARTESIAN_POINT('Ctrl Pts',(-0.146177880661274,-0.838799991293752,
-0.110146092169202));
#33908=CARTESIAN_POINT('Ctrl Pts',(0.271891391764026,-0.806889341727016,
-0.099561676462631));
#33909=CARTESIAN_POINT('Ctrl Pts',(0.506497030663811,-0.65517709938679,
-0.0925053993249171));
#33910=CARTESIAN_POINT('Ctrl Pts',(0.598678546627452,-0.555902285345007,
-0.0889772607560602));
#33911=CARTESIAN_POINT('',(0.555007866453735,-0.515351924808616,-0.12));
#33912=CARTESIAN_POINT('Ctrl Pts',(-0.485074560134038,-0.657451903693333,
-0.12));
#33913=CARTESIAN_POINT('Ctrl Pts',(-0.453585509292975,-0.678311536271596,
-0.12));
#33914=CARTESIAN_POINT('Ctrl Pts',(-0.420738538427646,-0.69688883557989,
-0.12));
#33915=CARTESIAN_POINT('Ctrl Pts',(-0.386803943986752,-0.713111122122748,
-0.12));
#33916=CARTESIAN_POINT('Ctrl Pts',(-0.352869989073431,-0.729333102942208,
-0.12));
#33917=CARTESIAN_POINT('Ctrl Pts',(-0.317847265092479,-0.743200535648918,
-0.12));
#33918=CARTESIAN_POINT('Ctrl Pts',(-0.281986661943899,-0.754592743143177,
-0.12));
#33919=CARTESIAN_POINT('Ctrl Pts',(-0.25594917278718,-0.762864340747765,
-0.12));
#33920=CARTESIAN_POINT('Ctrl Pts',(-0.229469505296541,-0.769830064822657,
-0.12));
#33921=CARTESIAN_POINT('Ctrl Pts',(-0.202642618162792,-0.775426102639142,
-0.12));
#33922=CARTESIAN_POINT('Ctrl Pts',(-0.195274171502223,-0.776963146648598,
-0.12));
#33923=CARTESIAN_POINT('Ctrl Pts',(-0.187880255104256,-0.778396492223848,
-0.12));
#33924=CARTESIAN_POINT('Ctrl Pts',(-0.180475767737279,-0.77972273894194,
-0.12));
#33925=CARTESIAN_POINT('Ctrl Pts',(-0.166033419323757,-0.782309564502668,
-0.12));
#33926=CARTESIAN_POINT('Ctrl Pts',(-0.151538081912919,-0.784491790556042,
-0.12));
#33927=CARTESIAN_POINT('Ctrl Pts',(-0.137004865545513,-0.786263720842398,
-0.12));
#33928=CARTESIAN_POINT('Ctrl Pts',(-0.100095238310191,-0.790763845570673,
-0.12));
#33929=CARTESIAN_POINT('Ctrl Pts',(-0.062941216534269,-0.792621345331588,
-0.12));
#33930=CARTESIAN_POINT('Ctrl Pts',(-0.0258198641282856,-0.791883010674467,
-0.12));
#33931=CARTESIAN_POINT('Ctrl Pts',(0.0040257252501598,-0.79128938917169,
-0.12));
#33932=CARTESIAN_POINT('Ctrl Pts',(0.033850610796128,-0.789016694488584,
-0.12));
#33933=CARTESIAN_POINT('Ctrl Pts',(0.0635063571245307,-0.78506522308135,
-0.12));
#33934=CARTESIAN_POINT('Ctrl Pts',(0.0773427424554382,-0.783221597889486,
-0.12));
#33935=CARTESIAN_POINT('Ctrl Pts',(0.0911422070143154,-0.78101223318484,
-0.12));
#33936=CARTESIAN_POINT('Ctrl Pts',(0.104888951391214,-0.778435636708654,
-0.12));
#33937=CARTESIAN_POINT('Ctrl Pts',(0.11244272845885,-0.777019807997451,
-0.12));
#33938=CARTESIAN_POINT('Ctrl Pts',(0.119978617799766,-0.775493331514105,
-0.12));
#33939=CARTESIAN_POINT('Ctrl Pts',(0.127482778723967,-0.773858786231397,
-0.12));
#33940=CARTESIAN_POINT('Ctrl Pts',(0.163232326177276,-0.766071872445965,
-0.12));
#33941=CARTESIAN_POINT('Ctrl Pts',(0.19833507148298,-0.755823166544053,
-0.12));
#33942=CARTESIAN_POINT('Ctrl Pts',(0.232522340421131,-0.743135834967468,
-0.12));
#33943=CARTESIAN_POINT('Ctrl Pts',(0.23781323037933,-0.741172318216354,
-0.12));
#33944=CARTESIAN_POINT('Ctrl Pts',(0.24308215822664,-0.739150297994117,
-0.12));
#33945=CARTESIAN_POINT('Ctrl Pts',(0.248328083260998,-0.737069756703629,
-0.12));
#33946=CARTESIAN_POINT('Ctrl Pts',(0.277906408593185,-0.725338951029881,
-0.12));
#33947=CARTESIAN_POINT('Ctrl Pts',(0.306754972760513,-0.711749564176307,
-0.12));
#33948=CARTESIAN_POINT('Ctrl Pts',(0.33471754468048,-0.696396977944507,
-0.12));
#33949=CARTESIAN_POINT('Ctrl Pts',(0.341939489363331,-0.69243183736938,
-0.12));
#33950=CARTESIAN_POINT('Ctrl Pts',(0.349102231022204,-0.688348968693442,
-0.12));
#33951=CARTESIAN_POINT('Ctrl Pts',(0.356202844546331,-0.68414978827903,
-0.12));
#33952=CARTESIAN_POINT('Ctrl Pts',(0.363162967591196,-0.680033691511815,
-0.12));
#33953=CARTESIAN_POINT('Ctrl Pts',(0.370055970561641,-0.675810190933559,
-0.12));
#33954=CARTESIAN_POINT('Ctrl Pts',(0.376876658719866,-0.671483106788984,
-0.12));
#33955=CARTESIAN_POINT('Ctrl Pts',(0.407456234430149,-0.652083246520597,
-0.12));
#33956=CARTESIAN_POINT('Ctrl Pts',(0.436604118223066,-0.630593159063361,
-0.12));
#33957=CARTESIAN_POINT('Ctrl Pts',(0.464102331907716,-0.607172277822429,
-0.12));
#33958=CARTESIAN_POINT('Ctrl Pts',(0.491112633064527,-0.584166963261629,
-0.12));
#33959=CARTESIAN_POINT('Ctrl Pts',(0.516532076728422,-0.559297921849101,
-0.12));
#33960=CARTESIAN_POINT('Ctrl Pts',(0.540116340222347,-0.53268395928398,
-0.12));
#33961=CARTESIAN_POINT('Ctrl Pts',(0.545165350090399,-0.526986339782151,
-0.12));
#33962=CARTESIAN_POINT('Ctrl Pts',(0.550130085793828,-0.521208653508965,
-0.12));
#33963=CARTESIAN_POINT('Ctrl Pts',(0.555007866453731,-0.51535192480862,
-0.12));
#33964=CARTESIAN_POINT('',(-0.45977880844898,0.601851132366392,-1.12625));
#33965=CARTESIAN_POINT('Ctrl Pts',(-0.459817636075324,0.601890711574507,
-1.12625));
#33966=CARTESIAN_POINT('Ctrl Pts',(-0.432503985120159,0.625165263761499,
-1.12625));
#33967=CARTESIAN_POINT('Ctrl Pts',(-0.403593713496176,0.646405611026526,
-1.12625));
#33968=CARTESIAN_POINT('Ctrl Pts',(-0.373360039769516,0.665530294929992,
-1.12625));
#33969=CARTESIAN_POINT('Ctrl Pts',(-0.342830078355216,0.684842399271405,
-1.12625));
#33970=CARTESIAN_POINT('Ctrl Pts',(-0.31094965018966,0.701997871851396,
-1.12625));
#33971=CARTESIAN_POINT('Ctrl Pts',(-0.27796322910615,0.716874587570177,
-1.12625));
#33972=CARTESIAN_POINT('Ctrl Pts',(-0.26649732981665,0.722045652468616,
-1.12625));
#33973=CARTESIAN_POINT('Ctrl Pts',(-0.25489754895223,0.726941007906489,
-1.12625));
#33974=CARTESIAN_POINT('Ctrl Pts',(-0.243173471025965,0.731554211541679,
-1.12625));
#33975=CARTESIAN_POINT('Ctrl Pts',(-0.235772847933684,0.734466217207855,
-1.12625));
#33976=CARTESIAN_POINT('Ctrl Pts',(-0.228323386858712,0.737265362583718,
-1.12625));
#33977=CARTESIAN_POINT('Ctrl Pts',(-0.220840169235029,0.739945834207436,
-1.12625));
#33978=CARTESIAN_POINT('Ctrl Pts',(-0.196274161507377,0.748745322600449,
-1.12625));
#33979=CARTESIAN_POINT('Ctrl Pts',(-0.171310177389595,0.756280719951804,
-1.12625));
#33980=CARTESIAN_POINT('Ctrl Pts',(-0.146041756546094,0.762513765607056,
-1.12625));
#33981=CARTESIAN_POINT('Ctrl Pts',(-0.114363689392252,0.770327900097807,
-1.12625));
#33982=CARTESIAN_POINT('Ctrl Pts',(-0.0822071438969236,0.776096397271709,
-1.12625));
#33983=CARTESIAN_POINT('Ctrl Pts',(-0.0497689197316195,0.779842549380837,
-1.12625));
#33984=CARTESIAN_POINT('Ctrl Pts',(-0.0298100993333156,0.782147508393075,
-1.12625));
#33985=CARTESIAN_POINT('Ctrl Pts',(-0.00974437858918223,0.783686221448921,
-1.12625));
#33986=CARTESIAN_POINT('Ctrl Pts',(0.0103835877242539,0.784457979579485,
-1.12625));
#33987=CARTESIAN_POINT('Ctrl Pts',(0.0199668006279772,0.784825424673551,
-1.12625));
#33988=CARTESIAN_POINT('Ctrl Pts',(0.0295667334937316,0.785018756675132,
-1.12625));
#33989=CARTESIAN_POINT('Ctrl Pts',(0.0391548342290692,0.785038051041727,
-1.12625));
#33990=CARTESIAN_POINT('Ctrl Pts',(0.0764066796325684,0.785113013829603,
-1.12625));
#33991=CARTESIAN_POINT('Ctrl Pts',(0.113553048502875,0.78256936197534,-1.12625));
#33992=CARTESIAN_POINT('Ctrl Pts',(0.150309494086452,0.777450709617537,
-1.12625));
#33993=CARTESIAN_POINT('Ctrl Pts',(0.181105692019783,0.773162073198534,
-1.12625));
#33994=CARTESIAN_POINT('Ctrl Pts',(0.211628935935288,0.767064947824063,
-1.12625));
#33995=CARTESIAN_POINT('Ctrl Pts',(0.241714208481675,0.759156929049669,
-1.12625));
#33996=CARTESIAN_POINT('Ctrl Pts',(0.258311234815943,0.754794342815885,
-1.12625));
#33997=CARTESIAN_POINT('Ctrl Pts',(0.274774951161251,0.7498801751997,-1.12625));
#33998=CARTESIAN_POINT('Ctrl Pts',(0.291082790748263,0.744427662964886,
-1.12625));
#33999=CARTESIAN_POINT('Ctrl Pts',(0.302253486658688,0.740692750329893,
-1.12625));
#34000=CARTESIAN_POINT('Ctrl Pts',(0.313351031746933,0.736705191681684,
-1.12625));
#34001=CARTESIAN_POINT('Ctrl Pts',(0.324367932126046,0.732468638719791,
-1.12625));
#34002=CARTESIAN_POINT('Ctrl Pts',(0.331410788639504,0.729760305740867,
-1.12625));
#34003=CARTESIAN_POINT('Ctrl Pts',(0.338411390393548,0.726953771030822,
-1.12625));
#34004=CARTESIAN_POINT('Ctrl Pts',(0.345367277998784,0.72405101276316,-1.12625));
#34005=CARTESIAN_POINT('Ctrl Pts',(0.379999812823046,0.709598525532694,
-1.12625));
#34006=CARTESIAN_POINT('Ctrl Pts',(0.413530302275784,0.692762730520492,
-1.12625));
#34007=CARTESIAN_POINT('Ctrl Pts',(0.445738862386387,0.673721922806366,
-1.12625));
#34008=CARTESIAN_POINT('Ctrl Pts',(0.478055825617878,0.654617030172785,
-1.12625));
#34009=CARTESIAN_POINT('Ctrl Pts',(0.509043040539765,0.633291742439725,
-1.12625));
#34010=CARTESIAN_POINT('Ctrl Pts',(0.538461112130543,0.609877570946797,
-1.12625));
#34011=CARTESIAN_POINT('Ctrl Pts',(0.555983532412802,0.595931281089083,
-1.12625));
#34012=CARTESIAN_POINT('Ctrl Pts',(0.57294884620594,0.58124300692065,-1.12625));
#34013=CARTESIAN_POINT('Ctrl Pts',(0.589301091561376,0.565833523687251,
-1.12625));
#34014=CARTESIAN_POINT('Ctrl Pts',(-0.45981763607532,0.60189071157451,-1.12625));
#34015=CARTESIAN_POINT('Ctrl Pts',(-0.466706837362044,0.59663400030589,
-1.12600649737474));
#34016=CARTESIAN_POINT('Ctrl Pts',(-0.571995661495496,0.513358547689712,
-1.12223485618063));
#34017=CARTESIAN_POINT('Ctrl Pts',(-0.731074678445066,0.297631408040497,
-1.11493507641766));
#34018=CARTESIAN_POINT('Ctrl Pts',(-0.784486575071109,-0.0873109114175124,
-1.10435066071109));
#34019=CARTESIAN_POINT('Ctrl Pts',(-0.647739858405562,-0.451090008407746,
-1.09376624500451));
#34020=CARTESIAN_POINT('Ctrl Pts',(-0.353965525798943,-0.705517309450159,
-1.08318182929794));
#34021=CARTESIAN_POINT('Ctrl Pts',(0.0256119661671953,-0.788917676587972,
-1.07259741359137));
#34022=CARTESIAN_POINT('Ctrl Pts',(0.398982356900775,-0.68107280850569,
-1.0620129978848));
#34023=CARTESIAN_POINT('Ctrl Pts',(0.675632891112325,-0.408126282767527,
-1.05142858217823));
#34024=CARTESIAN_POINT('Ctrl Pts',(0.788500750688368,-0.036244024752235,
-1.04084416647166));
#34025=CARTESIAN_POINT('Ctrl Pts',(0.710224521156416,0.344424265850668,
-1.03025975076509));
#34026=CARTESIAN_POINT('Ctrl Pts',(0.459779801870052,0.641599200064964,
-1.01967533505852));
#34027=CARTESIAN_POINT('Ctrl Pts',(0.0978778173933265,0.783241287520997,
-1.00909091935195));
#34028=CARTESIAN_POINT('Ctrl Pts',(-0.287751124101883,0.735014472176636,
-0.998506503645377));
#34029=CARTESIAN_POINT('Ctrl Pts',(-0.603625085401646,0.508609617298404,
-0.987922087938806));
#34030=CARTESIAN_POINT('Ctrl Pts',(-0.773171671953705,0.158910506780705,
-0.977337672232235));
#34031=CARTESIAN_POINT('Ctrl Pts',(-0.755290373416536,-0.229310787602247,
-0.966753256525666));
#34032=CARTESIAN_POINT('Ctrl Pts',(-0.554315867123394,-0.561943861908008,
-0.956168840819094));
#34033=CARTESIAN_POINT('Ctrl Pts',(-0.218967255152568,-0.758353694545466,
-0.945584425112523));
#34034=CARTESIAN_POINT('Ctrl Pts',(0.169462156609871,-0.770927728297872,
-0.935000009405953));
#34035=CARTESIAN_POINT('Ctrl Pts',(0.516811513855877,-0.596617837396195,
-0.924415593699381));
#34036=CARTESIAN_POINT('Ctrl Pts',(0.738878357065634,-0.277679236275885,
-0.913831177992811));
#34037=CARTESIAN_POINT('Ctrl Pts',(0.781830502198585,0.108572789396221,
-0.90324676228624));
#34038=CARTESIAN_POINT('Ctrl Pts',(0.635255734092279,0.468505215644773,
-0.892662346579668));
#34039=CARTESIAN_POINT('Ctrl Pts',(0.334685876135463,0.714865266390365,
-0.882077930873099));
#34040=CARTESIAN_POINT('Ctrl Pts',(-0.0470166324849965,0.78793173628669,
-0.871493515166526));
#34041=CARTESIAN_POINT('Ctrl Pts',(-0.417321635893158,0.669992266368472,
-0.860909099459958));
#34042=CARTESIAN_POINT('Ctrl Pts',(-0.686461896723765,0.389637073600391,
-0.850324683753385));
#34043=CARTESIAN_POINT('Ctrl Pts',(-0.789193960383511,0.0148282727314076,
-0.839740268046816));
#34044=CARTESIAN_POINT('Ctrl Pts',(-0.700614103026784,-0.363575113859105,
-0.829155852340243));
#34045=CARTESIAN_POINT('Ctrl Pts',(-0.442195350963467,-0.653842684721737,
-0.818571436633674));
#34046=CARTESIAN_POINT('Ctrl Pts',(-0.0765821114814572,-0.785609422664233,
-0.807987020927103));
#34047=CARTESIAN_POINT('Ctrl Pts',(0.30759572884442,-0.726933182881659,
-0.797402605220531));
#34048=CARTESIAN_POINT('Ctrl Pts',(0.617207958261565,-0.492037926420709,
-0.786818189513962));
#34049=CARTESIAN_POINT('Ctrl Pts',(0.777200137236411,-0.137865628267143,
-0.776233773807389));
#34050=CARTESIAN_POINT('Ctrl Pts',(0.748787869734938,0.249727273071264,
-0.76564935810082));
#34051=CARTESIAN_POINT('Ctrl Pts',(0.538858696398576,0.576782706132405,
-0.755064942394247));
#34052=CARTESIAN_POINT('Ctrl Pts',(0.198302456030384,0.764017748949664,
-0.744480526687679));
#34053=CARTESIAN_POINT('Ctrl Pts',(-0.190325140315885,0.76604394504593,
-0.733896110981106));
#34054=CARTESIAN_POINT('Ctrl Pts',(-0.532815196286454,0.582370115462685,
-0.723311695274537));
#34055=CARTESIAN_POINT('Ctrl Pts',(-0.746143216224096,0.257521427575564,
-0.712727279567965));
#34056=CARTESIAN_POINT('Ctrl Pts',(-0.778595432221924,-0.129754143290103,
-0.702142863861395));
#34057=CARTESIAN_POINT('Ctrl Pts',(-0.622304962251661,-0.48557545112449,
-0.691558448154824));
#34058=CARTESIAN_POINT('Ctrl Pts',(-0.315158855058534,-0.723686313851511,
-0.680974032448253));
#34059=CARTESIAN_POINT('Ctrl Pts',(0.0683862731776844,-0.786365247463709,
-0.670389616741682));
#34060=CARTESIAN_POINT('Ctrl Pts',(0.435353589178261,-0.65841798059242,
-0.659805201035111));
#34061=CARTESIAN_POINT('Ctrl Pts',(0.696784958823666,-0.37086076354192,
-0.649220785328541));
#34062=CARTESIAN_POINT('Ctrl Pts',(0.789305673168616,0.00659841508485431,
-0.638636369621969));
#34063=CARTESIAN_POINT('Ctrl Pts',(0.690487385718299,0.382458043374308,
-0.628051953915399));
#34064=CARTESIAN_POINT('Ctrl Pts',(0.424285064899531,0.665604363327791,
-0.617467538208828));
#34065=CARTESIAN_POINT('Ctrl Pts',(0.0552299665647796,0.787398650983761,
-0.606883122502258));
#34066=CARTESIAN_POINT('Ctrl Pts',(-0.32721366682163,0.71831622633972,-0.596298706795686));
#34067=CARTESIAN_POINT('Ctrl Pts',(-0.630336020111219,0.475103658718963,
-0.585714291089116));
#34068=CARTESIAN_POINT('Ctrl Pts',(-0.780655892709756,0.116719158475916,
-0.575129875382544));
#34069=CARTESIAN_POINT('Ctrl Pts',(-0.74173359420234,-0.269959737756342,
-0.564545459675975));
#34070=CARTESIAN_POINT('Ctrl Pts',(-0.523004447299988,-0.591196526446348,
-0.553961043969403));
#34071=CARTESIAN_POINT('Ctrl Pts',(-0.177491530455713,-0.769118808373767,
-0.543376628262832));
#34072=CARTESIAN_POINT('Ctrl Pts',(0.211047875895698,-0.760595673704307,
-0.532792212556262));
#34073=CARTESIAN_POINT('Ctrl Pts',(0.548426253918519,-0.567693252373757,
-0.522207796849691));
#34074=CARTESIAN_POINT('Ctrl Pts',(0.752858251913652,-0.237173854594718,
-0.511623381143121));
#34075=CARTESIAN_POINT('Ctrl Pts',(0.774786625126501,0.150839882998086,
-0.501038965436549));
#34076=CARTESIAN_POINT('Ctrl Pts',(0.608895621771471,0.502287872206101,
-0.490454549729978));
#34077=CARTESIAN_POINT('Ctrl Pts',(0.295399597411619,0.731974086035049,
-0.479870134023408));
#34078=CARTESIAN_POINT('Ctrl Pts',(-0.0897055208909264,0.784219296051476,
-0.469285718316836));
#34079=CARTESIAN_POINT('Ctrl Pts',(-0.453064735918975,0.646358514947008,
-0.458701302610267));
#34080=CARTESIAN_POINT('Ctrl Pts',(-0.706594568913721,0.351811170884782,
-0.448116886903694));
#34081=CARTESIAN_POINT('Ctrl Pts',(-0.788835756602106,-0.0280202406126237,
-0.437532471197125));
#34082=CARTESIAN_POINT('Ctrl Pts',(-0.679851857001817,-0.401059144402229,
-0.426948055490553));
#34083=CARTESIAN_POINT('Ctrl Pts',(-0.40606212854654,-0.676875566510091,
-0.416363639783983));
#34084=CARTESIAN_POINT('Ctrl Pts',(-0.0338371233843339,-0.788607655212058,
-0.405779224077412));
#34085=CARTESIAN_POINT('Ctrl Pts',(0.346590485190772,-0.709169951669667,
-0.395194808370841));
#34086=CARTESIAN_POINT('Ctrl Pts',(0.642999595336511,-0.45781929315021,
-0.38461039266427));
#34087=CARTESIAN_POINT('Ctrl Pts',(0.783536392737088,-0.0954866798141,-0.374025976957699));
#34088=CARTESIAN_POINT('Ctrl Pts',(0.734132744595485,0.28999327252795,-0.363441561251129));
#34089=CARTESIAN_POINT('Ctrl Pts',(0.506764802819446,0.605174701533931,
-0.352857145544558));
#34090=CARTESIAN_POINT('Ctrl Pts',(0.156549813679539,0.773653113881336,
-0.342272729837987));
#34091=CARTESIAN_POINT('Ctrl Pts',(-0.231615093084909,0.754586929064556,
-0.331688314131416));
#34092=CARTESIAN_POINT('Ctrl Pts',(-0.563633182964224,0.552598063281501,
-0.321103898424845));
#34093=CARTESIAN_POINT('Ctrl Pts',(-0.759018516340419,0.216651511277543,
-0.310519482718275));
#34094=CARTESIAN_POINT('Ctrl Pts',(-0.770406886705711,-0.171814470849813,
-0.299935067011703));
#34095=CARTESIAN_POINT('Ctrl Pts',(-0.595037595541406,-0.51863016343718,
-0.289350651305133));
#34096=CARTESIAN_POINT('Ctrl Pts',(-0.275422660164455,-0.739722476337532,
-0.278766235598562));
#34097=CARTESIAN_POINT('Ctrl Pts',(0.110958659106209,-0.781495462293021,
-0.268181819891991));
#34098=CARTESIAN_POINT('Ctrl Pts',(0.470442038027584,-0.633822758023187,
-0.25759740418542));
#34099=CARTESIAN_POINT('Ctrl Pts',(0.715883472822076,-0.332502328862273,
-0.24701298847885));
#34100=CARTESIAN_POINT('Ctrl Pts',(0.787784607225334,0.0494214101901685,
-0.236428572772279));
#34101=CARTESIAN_POINT('Ctrl Pts',(0.668715255345631,0.419364726111373,
-0.225844157065708));
#34102=CARTESIAN_POINT('Ctrl Pts',(0.387540164029798,0.687647957073736,
-0.215259741359137));
#34103=CARTESIAN_POINT('Ctrl Pts',(0.0124189653017137,0.789235606485634,
-0.204675325652566));
#34104=CARTESIAN_POINT('Ctrl Pts',(-0.36571115764945,0.699500976810335,
-0.194090909945996));
#34105=CARTESIAN_POINT('Ctrl Pts',(-0.655190820886875,0.440197805626221,
-0.183506494239425));
#34106=CARTESIAN_POINT('Ctrl Pts',(-0.785836630350134,0.0741833682121673,
-0.172922078532854));
#34107=CARTESIAN_POINT('Ctrl Pts',(-0.725996588748235,-0.309812190918388,
-0.162337662826283));
#34108=CARTESIAN_POINT('Ctrl Pts',(-0.490140575868305,-0.618708756217194,
-0.151753247119712));
#34109=CARTESIAN_POINT('Ctrl Pts',(-0.135514917188149,-0.777613622822952,
-0.141168831413142));
#34110=CARTESIAN_POINT('Ctrl Pts',(0.252058240770721,-0.748030699511341,
-0.130584415706571));
#34111=CARTESIAN_POINT('Ctrl Pts',(0.469550542503074,-0.607385125337196,
-0.123528138568857));
#34112=CARTESIAN_POINT('Ctrl Pts',(0.555007866453731,-0.51535192480862,
-0.12));
#34113=CARTESIAN_POINT('Ctrl Pts',(-0.453782243834444,0.594001620520161,
-1.1425283350431));
#34114=CARTESIAN_POINT('Ctrl Pts',(-0.550881388338776,0.519823594492225,
-1.13905034750894));
#34115=CARTESIAN_POINT('Ctrl Pts',(-0.707932320584144,0.323031319671974,
-1.13209437244062));
#34116=CARTESIAN_POINT('Ctrl Pts',(-0.776614466270609,-0.0485165662670082,
-1.12166040983814));
#34117=CARTESIAN_POINT('Ctrl Pts',(-0.662248238305507,-0.408538693637011,
-1.11122644723566));
#34118=CARTESIAN_POINT('Ctrl Pts',(-0.391780881856493,-0.672308433025167,
-1.10079248463318));
#34119=CARTESIAN_POINT('Ctrl Pts',(-0.0289685614302378,-0.777586532369439,
-1.0903585220307));
#34120=CARTESIAN_POINT('Ctrl Pts',(0.34067266544482,-0.699591456600571,
-1.07992455942821));
#34121=CARTESIAN_POINT('Ctrl Pts',(0.630013764781801,-0.456690366635246,
-1.06949059682574));
#34122=CARTESIAN_POINT('Ctrl Pts',(0.770854889346008,-0.10614597677494,
-1.05905663422325));
#34123=CARTESIAN_POINT('Ctrl Pts',(0.729998172573568,0.269419497799131,
-1.04862267162077));
#34124=CARTESIAN_POINT('Ctrl Pts',(0.517074073818031,0.581479511865621,
-1.03818870901829));
#34125=CARTESIAN_POINT('Ctrl Pts',(0.182270729955255,0.756479721113076,
-1.02775474641581));
#34126=CARTESIAN_POINT('Ctrl Pts',(-0.195495525574094,0.753170354596226,
-1.01732078381333));
#34127=CARTESIAN_POINT('Ctrl Pts',(-0.527181654493517,0.572331754114923,
-1.00688682121085));
#34128=CARTESIAN_POINT('Ctrl Pts',(-0.734606108414347,0.256589128857389,
-0.99645285860837));
#34129=CARTESIAN_POINT('Ctrl Pts',(-0.768876998658737,-0.119633940618221,
-0.98601889600589));
#34130=CARTESIAN_POINT('Ctrl Pts',(-0.621916351700688,-0.467658178639457,
-0.975584933403408));
#34131=CARTESIAN_POINT('Ctrl Pts',(-0.328364174807739,-0.705450981188055,
-0.965150970800928));
#34132=CARTESIAN_POINT('Ctrl Pts',(0.0425865250681795,-0.776962359283856,
-0.954717008198448));
#34133=CARTESIAN_POINT('Ctrl Pts',(0.403499180542327,-0.665336403825431,
-0.944283045595967));
#34134=CARTESIAN_POINT('Ctrl Pts',(0.669303286159028,-0.39688440440999,
-0.933849082993487));
#34135=CARTESIAN_POINT('Ctrl Pts',(0.777346315469044,-0.0348830195569227,
-0.923415120391006));
#34136=CARTESIAN_POINT('Ctrl Pts',(0.702161510858137,0.335340620697416,
-0.912981157788526));
#34137=CARTESIAN_POINT('Ctrl Pts',(0.461470637519422,0.626521324425118,
-0.902547195186045));
#34138=CARTESIAN_POINT('Ctrl Pts',(0.112006796904714,0.770025062366403,
-0.892113232583564));
#34139=CARTESIAN_POINT('Ctrl Pts',(-0.263858098652974,0.732026654580471,
-0.881679269981083));
#34140=CARTESIAN_POINT('Ctrl Pts',(-0.577529159980994,0.521482682939162,
-0.871245307378604));
#34141=CARTESIAN_POINT('Ctrl Pts',(-0.75507116928701,0.188020340781936,
-0.860811344776122));
#34142=CARTESIAN_POINT('Ctrl Pts',(-0.754635806007903,-0.189760163171063,
-0.850377382173643));
#34143=CARTESIAN_POINT('Ctrl Pts',(-0.576325689361536,-0.522812412838008,
-0.83994341957116));
#34144=CARTESIAN_POINT('Ctrl Pts',(-0.262170190030731,-0.732632862145289,
-0.82950945696868));
#34145=CARTESIAN_POINT('Ctrl Pts',(0.113781287599418,-0.769764858789943,
-0.819075494366201));
#34146=CARTESIAN_POINT('Ctrl Pts',(0.462913446150841,-0.625456042107332,
-0.808641531763718));
#34147=CARTESIAN_POINT('Ctrl Pts',(0.702932553865032,-0.333721356752229,
-0.79820756916124));
#34148=CARTESIAN_POINT('Ctrl Pts',(0.77726385077405,0.0366745895092527,
-0.787773606558758));
#34149=CARTESIAN_POINT('Ctrl Pts',(0.668386751451239,0.398425990267,-0.777339643956278));
#34150=CARTESIAN_POINT('Ctrl Pts',(0.401964611697131,0.666264639748313,
-0.766905681353798));
#34151=CARTESIAN_POINT('Ctrl Pts',(0.040795634331005,0.777058450475451,
-0.756471718751315));
#34152=CARTESIAN_POINT('Ctrl Pts',(-0.329989257542916,0.704692279751986,
-0.746037756148836));
#34153=CARTESIAN_POINT('Ctrl Pts',(-0.622992579377319,0.46622351428963,
-0.735603793546354));
#34154=CARTESIAN_POINT('Ctrl Pts',(-0.769150693862395,0.117861483813719,
-0.725169830943875));
#34155=CARTESIAN_POINT('Ctrl Pts',(-0.734012759466783,-0.258281606344191,
-0.714735868341394));
#34156=CARTESIAN_POINT('Ctrl Pts',(-0.525861117638763,-0.573545293931951,
-0.704301905738913));
#34157=CARTESIAN_POINT('Ctrl Pts',(-0.193759067069451,-0.753618964174968,
-0.693867943136433));
#34158=CARTESIAN_POINT('Ctrl Pts',(0.184013817024176,-0.756057560229359,
-0.683433980533952));
#34159=CARTESIAN_POINT('Ctrl Pts',(0.518412914638575,-0.580286282081279,
-0.673000017931472));
#34160=CARTESIAN_POINT('Ctrl Pts',(0.73061721497504,-0.267736072313561,
-0.66256605532899));
#34161=CARTESIAN_POINT('Ctrl Pts',(0.770608169635336,0.107922046529211,
-0.652132092726511));
#34162=CARTESIAN_POINT('Ctrl Pts',(0.62895953467438,0.458141924492798,-0.64169813012403));
#34163=CARTESIAN_POINT('Ctrl Pts',(0.339059224908714,0.700373444128258,
-0.63126416752155));
#34164=CARTESIAN_POINT('Ctrl Pts',(-0.0307605314660666,0.777520359180197,
-0.620830204919068));
#34165=CARTESIAN_POINT('Ctrl Pts',(-0.393329741412471,0.671398416557692,
-0.610396242316588));
#34166=CARTESIAN_POINT('Ctrl Pts',(-0.663187433844332,0.407021555727391,
-0.599962279714107));
#34167=CARTESIAN_POINT('Ctrl Pts',(-0.7767256138806,0.0467058880397563,
-0.589528317111627));
#34168=CARTESIAN_POINT('Ctrl Pts',(-0.707182265180476,-0.324618796513675,
-0.579094354509146));
#34169=CARTESIAN_POINT('Ctrl Pts',(-0.470949408769067,-0.619427779176751,
-0.568660391906665));
#34170=CARTESIAN_POINT('Ctrl Pts',(-0.123709349589919,-0.768231811408391,
-0.558226429304186));
#34171=CARTESIAN_POINT('Ctrl Pts',(0.252690166207058,-0.735956383991622,
-0.547792466701704));
#34172=CARTESIAN_POINT('Ctrl Pts',(0.569528234436075,-0.530209118571064,
-0.537358504099224));
#34173=CARTESIAN_POINT('Ctrl Pts',(0.752123144005562,-0.199486579716444,
-0.526924541496743));
#34174=CARTESIAN_POINT('Ctrl Pts',(0.757435558261682,0.178256821234392,
-0.516490578894262));
#34175=CARTESIAN_POINT('Ctrl Pts',(0.58421329122536,0.513983413731816,-0.506056616291782));
#34176=CARTESIAN_POINT('Ctrl Pts',(0.273286459598611,0.728559283954182,
-0.495622653689301));
#34177=CARTESIAN_POINT('Ctrl Pts',(-0.102056559562226,0.77140688218741,
-0.485188691086821));
#34178=CARTESIAN_POINT('Ctrl Pts',(-0.453343888260034,0.63242662674262,
-0.47475472848434));
#34179=CARTESIAN_POINT('Ctrl Pts',(-0.697773800873293,0.344377470300547,
-0.46432076588186));
#34180=CARTESIAN_POINT('Ctrl Pts',(-0.777731869256008,-0.0248446931832595,
-0.453886803279379));
#34181=CARTESIAN_POINT('Ctrl Pts',(-0.674371225051026,-0.388210728933218,
-0.443452840676899));
#34182=CARTESIAN_POINT('Ctrl Pts',(-0.412054943730941,-0.660071846530996,
-0.433018878074418));
#34183=CARTESIAN_POINT('Ctrl Pts',(-0.0526134386847218,-0.776347824950465,
-0.422584915471937));
#34184=CARTESIAN_POINT('Ctrl Pts',(0.319229548446936,-0.709631323036316,
-0.412150952869456));
#34185=CARTESIAN_POINT('Ctrl Pts',(0.615827130120359,-0.475648047450979,
-0.401716990266976));
#34186=CARTESIAN_POINT('Ctrl Pts',(0.767268468189365,-0.129550055793601,
-0.391283027664495));
#34187=CARTESIAN_POINT('Ctrl Pts',(0.737857415668762,0.24708410184319,-0.380849065062015));
#34188=CARTESIAN_POINT('Ctrl Pts',(0.534526434095284,0.565478213973463,
-0.370415102459534));
#34189=CARTESIAN_POINT('Ctrl Pts',(0.205202547258304,0.750583795355781,
-0.359981139857054));
#34190=CARTESIAN_POINT('Ctrl Pts',(-0.172489509004567,0.758769720339229,
-0.349547177254573));
#34191=CARTESIAN_POINT('Ctrl Pts',(-0.509524166428113,0.588106489551379,
-0.339113214652093));
#34192=CARTESIAN_POINT('Ctrl Pts',(-0.726459188269098,0.278821030603052,
-0.328679252049611));
#34193=CARTESIAN_POINT('Ctrl Pts',(-0.772160950053184,-0.0961851660426477,
-0.318245289447131));
#34194=CARTESIAN_POINT('Ctrl Pts',(-0.635857117988058,-0.448519615362849,
-0.307811326844651));
#34195=CARTESIAN_POINT('Ctrl Pts',(-0.349675784487423,-0.695133774103561,
-0.29737736424217));
#34196=CARTESIAN_POINT('Ctrl Pts',(0.0189274157531888,-0.777898369643474,
-0.28694340163969));
#34197=CARTESIAN_POINT('Ctrl Pts',(0.383069251609914,-0.67730500314506,
-0.276509439037209));
#34198=CARTESIAN_POINT('Ctrl Pts',(0.656918053157321,-0.417064487823481,
-0.266075476434728));
#34199=CARTESIAN_POINT('Ctrl Pts',(0.775925115315038,-0.0585179376441977,
-0.255641513832248));
#34200=CARTESIAN_POINT('Ctrl Pts',(0.712039292365909,0.313821812003488,
-0.245207551229767));
#34201=CARTESIAN_POINT('Ctrl Pts',(0.480319196218496,0.612190866640263,
-0.234773588627287));
#34202=CARTESIAN_POINT('Ctrl Pts',(0.135383189993241,0.766260668703223,
-0.224339626024806));
#34203=CARTESIAN_POINT('Ctrl Pts',(-0.241463591288354,0.739715845333339,
-0.213905663422325));
#34204=CARTESIAN_POINT('Ctrl Pts',(-0.561395755032469,0.5388126158932,-0.203471700819845));
#34205=CARTESIAN_POINT('Ctrl Pts',(-0.749000440414916,0.210907029399775,
-0.193037738217364));
#34206=CARTESIAN_POINT('Ctrl Pts',(-0.76006108477016,-0.166712982541228,
-0.182603775614884));
#34207=CARTESIAN_POINT('Ctrl Pts',(-0.591963456523644,-0.505033918677001,
-0.172169813012403));
#34208=CARTESIAN_POINT('Ctrl Pts',(-0.284343786563683,-0.724320025643106,
-0.161735850409922));
#34209=CARTESIAN_POINT('Ctrl Pts',(0.09031673140191,-0.772864465068915,
-0.151301887807442));
#34210=CARTESIAN_POINT('Ctrl Pts',(0.44365235923649,-0.639262442637623,
-0.140867925204961));
#34211=CARTESIAN_POINT('Ctrl Pts',(0.692489824641788,-0.354929918130683,
-0.13043396260248));
#34212=CARTESIAN_POINT('Ctrl Pts',(0.749438361810141,-0.109676867461678,
-0.12347798753416));
#34213=CARTESIAN_POINT('Ctrl Pts',(0.747395528060274,0.012496985056547,
-0.12));
#34214=CARTESIAN_POINT('Ctrl Pts',(-0.453782243834444,0.594001620520161,
-1.13966850381659));
#34215=CARTESIAN_POINT('Ctrl Pts',(-0.550881059946454,0.519823845364613,
-1.13619051628243));
#34216=CARTESIAN_POINT('Ctrl Pts',(-0.707932492103511,0.323031139564096,
-1.12923454121411));
#34217=CARTESIAN_POINT('Ctrl Pts',(-0.776614348027596,-0.0485164852858574,
-1.11880057861163));
#34218=CARTESIAN_POINT('Ctrl Pts',(-0.662248261705559,-0.40853871944569,
-1.10836661600915));
#34219=CARTESIAN_POINT('Ctrl Pts',(-0.391780845205783,-0.67230838997676,
-1.09793265340667));
#34220=CARTESIAN_POINT('Ctrl Pts',(-0.0289685722792028,-0.777586516102956,
-1.08749869080419));
#34221=CARTESIAN_POINT('Ctrl Pts',(0.340672659850851,-0.699591427563088,
-1.07706472820171));
#34222=CARTESIAN_POINT('Ctrl Pts',(0.630013740257188,-0.456690353715162,
-1.06663076559923));
#34223=CARTESIAN_POINT('Ctrl Pts',(0.770854864632094,-0.106145971815373,
-1.05619680299675));
#34224=CARTESIAN_POINT('Ctrl Pts',(0.72999814690911,0.269419487936225,-1.04576284039427));
#34225=CARTESIAN_POINT('Ctrl Pts',(0.517074056599653,0.581479492398165,
-1.03532887779179));
#34226=CARTESIAN_POINT('Ctrl Pts',(0.182270723540412,0.75647969515944,-1.02489491518931));
#34227=CARTESIAN_POINT('Ctrl Pts',(-0.195495518808877,0.753170329021126,
-1.01446095258683));
#34228=CARTESIAN_POINT('Ctrl Pts',(-0.527181636582195,0.572331734566925,
-1.00402698998434));
#34229=CARTESIAN_POINT('Ctrl Pts',(-0.734606083355523,0.256589120137115,
-0.993593027381866));
#34230=CARTESIAN_POINT('Ctrl Pts',(-0.768876972472471,-0.119633936553389,
-0.983159064779384));
#34231=CARTESIAN_POINT('Ctrl Pts',(-0.62191633050167,-0.467658162697799,
-0.972725102176903));
#34232=CARTESIAN_POINT('Ctrl Pts',(-0.328364163622079,-0.705450957152499,
-0.962291139574423));
#34233=CARTESIAN_POINT('Ctrl Pts',(0.0425865236188069,-0.776962332806937,
-0.951857176971942));
#34234=CARTESIAN_POINT('Ctrl Pts',(0.403499166791987,-0.665336381154547,
-0.941423214369462));
#34235=CARTESIAN_POINT('Ctrl Pts',(0.669303263352647,-0.396884390885559,
-0.930989251766981));
#34236=CARTESIAN_POINT('Ctrl Pts',(0.777346288980351,-0.0348830183684687,
-0.920555289164501));
#34237=CARTESIAN_POINT('Ctrl Pts',(0.702161486931755,0.335340609270621,
-0.910121326562019));
#34238=CARTESIAN_POINT('Ctrl Pts',(0.461470621794522,0.626521303076042,
-0.89968736395954));
#34239=CARTESIAN_POINT('Ctrl Pts',(0.112006793088058,0.770025036127444,
-0.889253401357058));
#34240=CARTESIAN_POINT('Ctrl Pts',(-0.263858089661894,0.732026629636288,
-0.878819438754579));
#34241=CARTESIAN_POINT('Ctrl Pts',(-0.577529140301394,0.521482665169388,
-0.868385476152096));
#34242=CARTESIAN_POINT('Ctrl Pts',(-0.75507114355759,0.188020334375047,
-0.857951513549617));
#34243=CARTESIAN_POINT('Ctrl Pts',(-0.754635780293312,-0.189760156704889,
-0.847517550947136));
#34244=CARTESIAN_POINT('Ctrl Pts',(-0.576325669722955,-0.522812395022917,
-0.837083588344655));
#34245=CARTESIAN_POINT('Ctrl Pts',(-0.262170181097151,-0.732632837180461,
-0.826649625742175));
#34246=CARTESIAN_POINT('Ctrl Pts',(0.113781283722264,-0.769764832559825,
-0.816215663139694));
#34247=CARTESIAN_POINT('Ctrl Pts',(0.462913430376836,-0.625456020794608,
-0.805781700537214));
#34248=CARTESIAN_POINT('Ctrl Pts',(0.702932529912257,-0.333721345380509,
-0.795347737934733));
#34249=CARTESIAN_POINT('Ctrl Pts',(0.7772638242884,0.0366745882595479,-0.784913775332253));
#34250=CARTESIAN_POINT('Ctrl Pts',(0.668386728675629,0.398425976690438,
-0.774479812729771));
#34251=CARTESIAN_POINT('Ctrl Pts',(0.401964597999989,0.666264617045014,
-0.764045850127292));
#34252=CARTESIAN_POINT('Ctrl Pts',(0.0407956329408734,0.777058423996801,
-0.75361188752481));
#34253=CARTESIAN_POINT('Ctrl Pts',(-0.329989246298369,0.704692255739247,
-0.74317792492233));
#34254=CARTESIAN_POINT('Ctrl Pts',(-0.622992558148538,0.466223498402834,
-0.732743962319849));
#34255=CARTESIAN_POINT('Ctrl Pts',(-0.769150667653204,0.11786147979753,
-0.722309999717369));
#34256=CARTESIAN_POINT('Ctrl Pts',(-0.734012734454935,-0.258281597543118,
-0.711876037114888));
#34257=CARTESIAN_POINT('Ctrl Pts',(-0.525861099719785,-0.573545274388111,
-0.701442074512408));
#34258=CARTESIAN_POINT('Ctrl Pts',(-0.193759060467015,-0.75361893849503,
-0.691008111909926));
#34259=CARTESIAN_POINT('Ctrl Pts',(0.184013810753814,-0.756057534466323,
-0.680574149307447));
#34260=CARTESIAN_POINT('Ctrl Pts',(0.518412896973398,-0.580286262307737,
-0.670140186704965));
#34261=CARTESIAN_POINT('Ctrl Pts',(0.730617190078897,-0.267736063190322,
-0.659706224102486));
#34262=CARTESIAN_POINT('Ctrl Pts',(0.770608143376481,0.107922042851714,
-0.649272261500004));
#34263=CARTESIAN_POINT('Ctrl Pts',(0.628959513242272,0.458141908881385,
-0.638838298897525));
#34264=CARTESIAN_POINT('Ctrl Pts',(0.339059213355103,0.700373420262687,
-0.628404336295043));
#34265=CARTESIAN_POINT('Ctrl Pts',(-0.0307605304178867,0.777520332685805,
-0.617970373692563));
#34266=CARTESIAN_POINT('Ctrl Pts',(-0.393329728009565,0.671398393679458,
-0.607536411090083));
#34267=CARTESIAN_POINT('Ctrl Pts',(-0.663187411245893,0.40702154185793,
-0.597102448487601));
#34268=CARTESIAN_POINT('Ctrl Pts',(-0.77672558741329,0.0467058864482299,
-0.586668485885122));
#34269=CARTESIAN_POINT('Ctrl Pts',(-0.707182241082891,-0.324618785452129,
-0.57623452328264));
#34270=CARTESIAN_POINT('Ctrl Pts',(-0.470949392721232,-0.619427758069444,
-0.56580056068016));
#34271=CARTESIAN_POINT('Ctrl Pts',(-0.123709345374462,-0.768231785230512,
-0.555366598077679));
#34272=CARTESIAN_POINT('Ctrl Pts',(0.252690157596516,-0.735956358913545,
-0.544932635475199));
#34273=CARTESIAN_POINT('Ctrl Pts',(0.569528215029119,-0.530209100503926,
-0.534498672872717));
#34274=CARTESIAN_POINT('Ctrl Pts',(0.752123118376594,-0.19948657291884,
-0.524064710270238));
#34275=CARTESIAN_POINT('Ctrl Pts',(0.757435532451691,0.178256815160203,
-0.513630747667757));
#34276=CARTESIAN_POINT('Ctrl Pts',(0.584213271318003,0.513983396217577,
-0.503196785065276));
#34277=CARTESIAN_POINT('Ctrl Pts',(0.27328645028624,0.728559259128164,-0.492762822462796));
#34278=CARTESIAN_POINT('Ctrl Pts',(-0.102056556084598,0.771406855901339,
-0.482328859860315));
#34279=CARTESIAN_POINT('Ctrl Pts',(-0.453343872812117,0.63242660519237,
-0.471894897257835));
#34280=CARTESIAN_POINT('Ctrl Pts',(-0.697773777096305,0.344377458565714,
-0.461460934655354));
#34281=CARTESIAN_POINT('Ctrl Pts',(-0.77773184275441,-0.0248446923366639,
-0.451026972052874));
#34282=CARTESIAN_POINT('Ctrl Pts',(-0.674371202071493,-0.388210715704746,
-0.440593009450393));
#34283=CARTESIAN_POINT('Ctrl Pts',(-0.412054929689965,-0.66007182403872,
-0.430159046847912));
#34284=CARTESIAN_POINT('Ctrl Pts',(-0.0526134368918924,-0.776347798496031,
-0.419725084245431));
#34285=CARTESIAN_POINT('Ctrl Pts',(0.31922953756903,-0.709631298855274,
-0.409291121642952));
#34286=CARTESIAN_POINT('Ctrl Pts',(0.615827109135746,-0.475648031243042,
-0.39885715904047));
#34287=CARTESIAN_POINT('Ctrl Pts',(0.767268442044312,-0.129550051379108,
-0.38842319643799));
#34288=CARTESIAN_POINT('Ctrl Pts',(0.737857390525905,0.247084093423657,
-0.377989233835509));
#34289=CARTESIAN_POINT('Ctrl Pts',(0.534526415881033,0.565478194704553,
-0.367555271233028));
#34290=CARTESIAN_POINT('Ctrl Pts',(0.205202540265923,0.750583769779188,
-0.357121308630548));
#34291=CARTESIAN_POINT('Ctrl Pts',(-0.172489503126895,0.758769694483932,
-0.346687346028067));
#34292=CARTESIAN_POINT('Ctrl Pts',(-0.509524149065839,0.58810646951105,
-0.336253383425587));
#34293=CARTESIAN_POINT('Ctrl Pts',(-0.726459163514615,0.278821021102697,
-0.325819420823106));
#34294=CARTESIAN_POINT('Ctrl Pts',(-0.772160923741469,-0.0961851627662888,
-0.315385458220626));
#34295=CARTESIAN_POINT('Ctrl Pts',(-0.63585709632081,-0.448519600076963,
-0.304951495618145));
#34296=CARTESIAN_POINT('Ctrl Pts',(-0.34967577257225,-0.695133750421173,
-0.294517533015665));
#34297=CARTESIAN_POINT('Ctrl Pts',(0.0189274151086266,-0.777898343127075,
-0.284083570413184));
#34298=CARTESIAN_POINT('Ctrl Pts',(0.383069238555855,-0.677304980083515,
-0.273649607810703));
#34299=CARTESIAN_POINT('Ctrl Pts',(0.656918030774058,-0.417064473576466,
-0.263215645208223));
#34300=CARTESIAN_POINT('Ctrl Pts',(0.775925088871968,-0.0585179357197007,
-0.252781682605742));
#34301=CARTESIAN_POINT('Ctrl Pts',(0.712039268108796,0.313821801446672,
-0.242347720003262));
#34302=CARTESIAN_POINT('Ctrl Pts',(0.480319179839619,0.612190845510335,
-0.23191375740078));
#34303=CARTESIAN_POINT('Ctrl Pts',(0.135383185403138,0.766260643122266,
-0.2214797947983));
#34304=CARTESIAN_POINT('Ctrl Pts',(-0.241463583105909,0.73971581908474,
-0.21104583219582));
#34305=CARTESIAN_POINT('Ctrl Pts',(-0.561395735813007,0.538812599584091,
-0.200611869593339));
#34306=CARTESIAN_POINT('Ctrl Pts',(-0.749000415068712,0.210907018176796,
-0.190177906990859));
#34307=CARTESIAN_POINT('Ctrl Pts',(-0.760061058523674,-0.166712968918093,
-0.179743944388378));
#34308=CARTESIAN_POINT('Ctrl Pts',(-0.59196343703511,-0.505033917097267,
-0.169309981785897));
#34309=CARTESIAN_POINT('Ctrl Pts',(-0.284343775530136,-0.724319970193124,
-0.158876019183416));
#34310=CARTESIAN_POINT('Ctrl Pts',(0.0903167256720993,-0.772864499431969,
-0.148442056580936));
#34311=CARTESIAN_POINT('Ctrl Pts',(0.443652349415121,-0.639262299658962,
-0.138008093978455));
#34312=CARTESIAN_POINT('Ctrl Pts',(0.69248978975463,-0.354930164383859,
-0.127574131375975));
#34313=CARTESIAN_POINT('Ctrl Pts',(0.749438354901214,-0.109676454265914,
-0.120618156307654));
#34314=CARTESIAN_POINT('Ctrl Pts',(0.747395528060274,0.012496985056547,
-0.117140168773494));
#34315=CARTESIAN_POINT('Ctrl Pts',(-0.454743647135464,0.59526009884658,
-1.13299148312149));
#34316=CARTESIAN_POINT('Ctrl Pts',(-0.552049078435987,0.520924481859268,
-1.12951349558733));
#34317=CARTESIAN_POINT('Ctrl Pts',(-0.709431880792854,0.323716019874443,
-1.12255752051901));
#34318=CARTESIAN_POINT('Ctrl Pts',(-0.778260040912912,-0.048619495750048,
-1.11212355791653));
#34319=CARTESIAN_POINT('Ctrl Pts',(-0.663651266471094,-0.409404197277858,
-1.10168959531405));
#34320=CARTESIAN_POINT('Ctrl Pts',(-0.392610989723487,-0.673732890143879,
-1.09125563271157));
#34321=CARTESIAN_POINT('Ctrl Pts',(-0.0290299167445311,-0.779233990024141,
-1.08082167010908));
#34322=CARTESIAN_POINT('Ctrl Pts',(0.341394439427495,-0.701073692506756,
-1.0703877075066));
#34323=CARTESIAN_POINT('Ctrl Pts',(0.631348582478227,-0.457657953570587,
-1.05995374490412));
#34324=CARTESIAN_POINT('Ctrl Pts',(0.772488099658164,-0.106370870957121,
-1.04951978230164));
#34325=CARTESIAN_POINT('Ctrl Pts',(0.731544823668042,0.269990319029405,
-1.03908581969916));
#34326=CARTESIAN_POINT('Ctrl Pts',(0.51816959980594,0.582711493978724,-1.02865185709668));
#34327=CARTESIAN_POINT('Ctrl Pts',(0.182656907952848,0.758082477697759,
-1.0182178944942));
#34328=CARTESIAN_POINT('Ctrl Pts',(-0.19590972281978,0.754766099154424,
-1.00778393189172));
#34329=CARTESIAN_POINT('Ctrl Pts',(-0.528298596051656,0.573544355519815,
-0.997349969289239));
#34330=CARTESIAN_POINT('Ctrl Pts',(-0.736162521039286,0.257132765118676,
-0.98691600668676));
#34331=CARTESIAN_POINT('Ctrl Pts',(-0.77050602107108,-0.119887409454019,
-0.976482044084279));
#34332=CARTESIAN_POINT('Ctrl Pts',(-0.623234008102322,-0.46864900769872,
-0.966048081481798));
#34333=CARTESIAN_POINT('Ctrl Pts',(-0.329059881148492,-0.706945622689532,
-0.955614118879318));
#34334=CARTESIAN_POINT('Ctrl Pts',(0.0426767532874504,-0.778608512204756,
-0.945180156276837));
#34335=CARTESIAN_POINT('Ctrl Pts',(0.404354075695015,-0.666746054432853,
-0.934746193674357));
#34336=CARTESIAN_POINT('Ctrl Pts',(0.670721341414739,-0.397725284812044,
-0.924312231071876));
#34337=CARTESIAN_POINT('Ctrl Pts',(0.778993281877019,-0.0349569263343644,
-0.913878268469395));
#34338=CARTESIAN_POINT('Ctrl Pts',(0.703649182952154,0.336051108064826,
-0.903444305866915));
#34339=CARTESIAN_POINT('Ctrl Pts',(0.462448357003043,0.627848737386999,
-0.893010343264434));
#34340=CARTESIAN_POINT('Ctrl Pts',(0.112244106104242,0.771656517208898,
-0.882576380661952));
#34341=CARTESIAN_POINT('Ctrl Pts',(-0.264417135746451,0.733577602061106,
-0.872142418059474));
#34342=CARTESIAN_POINT('Ctrl Pts',(-0.578752773069475,0.522587550157066,
-0.861708455456991));
#34343=CARTESIAN_POINT('Ctrl Pts',(-0.756670941263009,0.188418700147704,
-0.851274492854512));
#34344=CARTESIAN_POINT('Ctrl Pts',(-0.756234655578182,-0.19016220870472,
-0.840840530252031));
#34345=CARTESIAN_POINT('Ctrl Pts',(-0.577546752652513,-0.523920097359396,
-0.83040656764955));
#34346=CARTESIAN_POINT('Ctrl Pts',(-0.262725650946226,-0.734185094000027,
-0.81997260504707));
#34347=CARTESIAN_POINT('Ctrl Pts',(0.114022356418756,-0.771395762338239,
-0.809538642444589));
#34348=CARTESIAN_POINT('Ctrl Pts',(0.463894222518143,-0.626781198051682,
-0.799104679842109));
#34349=CARTESIAN_POINT('Ctrl Pts',(0.70442185957082,-0.334428413379528,
-0.788670717239628));
#34350=CARTESIAN_POINT('Ctrl Pts',(0.778910642463376,0.0367522920926843,
-0.778236754637148));
#34351=CARTESIAN_POINT('Ctrl Pts',(0.669802864842397,0.399270136831811,
-0.767802792034666));
#34352=CARTESIAN_POINT('Ctrl Pts',(0.402816255551772,0.667676257013847,
-0.757368829432186));
#34353=CARTESIAN_POINT('Ctrl Pts',(0.0408820681867802,0.778704806982432,
-0.746934866829706));
#34354=CARTESIAN_POINT('Ctrl Pts',(-0.330688406958327,0.706185313795279,
-0.736500904227224));
#34355=CARTESIAN_POINT('Ctrl Pts',(-0.624312515974406,0.46721130371009,
-0.726066941624745));
#34356=CARTESIAN_POINT('Ctrl Pts',(-0.770780296177272,0.118111197359309,
-0.715632979022264));
#34357=CARTESIAN_POINT('Ctrl Pts',(-0.73556791491489,-0.258828828503577,
-0.705199016419783));
#34358=CARTESIAN_POINT('Ctrl Pts',(-0.526975261461873,-0.574760466389229,
-0.694765053817303));
#34359=CARTESIAN_POINT('Ctrl Pts',(-0.19416958509504,-0.755215659358831,
-0.684331091214822));
#34360=CARTESIAN_POINT('Ctrl Pts',(0.18440368775378,-0.757659422075367,
-0.673897128612342));
#34361=CARTESIAN_POINT('Ctrl Pts',(0.519511277927458,-0.581515736694162,
-0.663463166009861));
#34362=CARTESIAN_POINT('Ctrl Pts',(0.732165176270937,-0.268303325683674,
-0.65302920340738));
#34363=CARTESIAN_POINT('Ctrl Pts',(0.772240859909325,0.108150701353621,
-0.6425952408049));
#34364=CARTESIAN_POINT('Ctrl Pts',(0.63029211348091,0.459112591420168,-0.632161278202419));
#34365=CARTESIAN_POINT('Ctrl Pts',(0.339777590896291,0.701857327839131,
-0.621727315599939));
#34366=CARTESIAN_POINT('Ctrl Pts',(-0.0308257039136559,0.779167694334796,
-0.611293352997458));
#34367=CARTESIAN_POINT('Ctrl Pts',(-0.394163090536681,0.672820910774439,
-0.600859390394977));
#34368=CARTESIAN_POINT('Ctrl Pts',(-0.664592531422757,0.407883913747361,
-0.590425427792497));
#34369=CARTESIAN_POINT('Ctrl Pts',(-0.778371265205501,0.0468048439711169,
-0.579991465190016));
#34370=CARTESIAN_POINT('Ctrl Pts',(-0.708680574764767,-0.325306567514172,
-0.569557502587535));
#34371=CARTESIAN_POINT('Ctrl Pts',(-0.471947210958994,-0.620740163018957,
-0.559123539985055));
#34372=CARTESIAN_POINT('Ctrl Pts',(-0.12397145302956,-0.769859466883738,
-0.548689577382575));
#34373=CARTESIAN_POINT('Ctrl Pts',(0.253225541762308,-0.737515657403935,
-0.538255614780094));
#34374=CARTESIAN_POINT('Ctrl Pts',(0.570734895935091,-0.531332474519237,
-0.527821652177613));
#34375=CARTESIAN_POINT('Ctrl Pts',(0.753716669989902,-0.199909232643481,
-0.517387689575133));
#34376=CARTESIAN_POINT('Ctrl Pts',(0.759040339677031,0.17863449459651,-0.506953726972652));
#34377=CARTESIAN_POINT('Ctrl Pts',(0.585451066006505,0.515072392221348,
-0.496519764370171));
#34378=CARTESIAN_POINT('Ctrl Pts',(0.273865472594036,0.730102885104296,
-0.486085801767691));
#34379=CARTESIAN_POINT('Ctrl Pts',(-0.102272787158506,0.773041264696527,
-0.47565183916521));
#34380=CARTESIAN_POINT('Ctrl Pts',(-0.454304389570946,0.633766551289466,
-0.465217876562729));
#34381=CARTESIAN_POINT('Ctrl Pts',(-0.699252176710741,0.345107104073579,
-0.454783913960249));
#34382=CARTESIAN_POINT('Ctrl Pts',(-0.779379652537759,-0.0248973317232062,
-0.444349951357768));
#34383=CARTESIAN_POINT('Ctrl Pts',(-0.675800017767717,-0.389033232387453,
-0.433915988755288));
#34384=CARTESIAN_POINT('Ctrl Pts',(-0.412927966008004,-0.661470343103483,
-0.423482026152808));
#34385=CARTESIAN_POINT('Ctrl Pts',(-0.0527249109646764,-0.777992675852612,
-0.413048063550326));
#34386=CARTESIAN_POINT('Ctrl Pts',(0.319905901228356,-0.711134821448214,
-0.402614100947846));
#34387=CARTESIAN_POINT('Ctrl Pts',(0.617131885254584,-0.476655804663409,
-0.392180138345365));
#34388=CARTESIAN_POINT('Ctrl Pts',(0.768894082626002,-0.129824533958299,
-0.381746175742884));
#34389=CARTESIAN_POINT('Ctrl Pts',(0.739420716803662,0.247607599809939,
-0.371312213140404));
#34390=CARTESIAN_POINT('Ctrl Pts',(0.535658937155234,0.566676294679626,
-0.360878250537923));
#34391=CARTESIAN_POINT('Ctrl Pts',(0.205637310626139,0.752174059916794,
-0.350444287935443));
#34392=CARTESIAN_POINT('Ctrl Pts',(-0.172854963141732,0.760377328448251,
-0.340010325332963));
#34393=CARTESIAN_POINT('Ctrl Pts',(-0.510603697094476,0.58935251286622,
-0.329576362730482));
#34394=CARTESIAN_POINT('Ctrl Pts',(-0.727998339939048,0.279411769712726,
-0.319142400128001));
#34395=CARTESIAN_POINT('Ctrl Pts',(-0.773796930208484,-0.0963889538944908,
-0.308708437525521));
#34396=CARTESIAN_POINT('Ctrl Pts',(-0.637204310729103,-0.449469895473667,
-0.29827447492304));
#34397=CARTESIAN_POINT('Ctrl Pts',(-0.350416643817245,-0.696606556498865,
-0.287840512320559));
#34398=CARTESIAN_POINT('Ctrl Pts',(0.0189675173356764,-0.779546505705979,
-0.277406549718079));
#34399=CARTESIAN_POINT('Ctrl Pts',(0.383880861799188,-0.678740011636779,
-0.266972587115598));
#34400=CARTESIAN_POINT('Ctrl Pts',(0.65830986777388,-0.417948123900598,
-0.256538624513118));
#34401=CARTESIAN_POINT('Ctrl Pts',(0.777569070626036,-0.0586419196868223,
-0.246104661910636));
#34402=CARTESIAN_POINT('Ctrl Pts',(0.713547892540654,0.314486707157708,
-0.235670699308157));
#34403=CARTESIAN_POINT('Ctrl Pts',(0.481336850230822,0.613487918075931,
-0.225236736705676));
#34404=CARTESIAN_POINT('Ctrl Pts',(0.135670026800076,0.767884146994865,
-0.214802774103195));
#34405=CARTESIAN_POINT('Ctrl Pts',(-0.241975180980523,0.741283085733481,
-0.204368811500715));
#34406=CARTESIAN_POINT('Ctrl Pts',(-0.562585186373481,0.539954196552607,
-0.193934848898234));
#34407=CARTESIAN_POINT('Ctrl Pts',(-0.750587350010884,0.211353885858112,
-0.183500886295754));
#34408=CARTESIAN_POINT('Ctrl Pts',(-0.76167142949834,-0.167066211673776,
-0.173066923693273));
#34409=CARTESIAN_POINT('Ctrl Pts',(-0.593217650425967,-0.506103908795648,
-0.162632961090792));
#34410=CARTESIAN_POINT('Ctrl Pts',(-0.284946229083341,-0.725854698300192,
-0.152198998488312));
#34411=CARTESIAN_POINT('Ctrl Pts',(0.090508090371596,-0.77450183073683,
-0.141765035885831));
#34412=CARTESIAN_POINT('Ctrl Pts',(0.44459231790613,-0.640617059956736,
-0.131331073283351));
#34413=CARTESIAN_POINT('Ctrl Pts',(0.693957024835472,-0.355681462393161,
-0.12089711068087));
#34414=CARTESIAN_POINT('Ctrl Pts',(0.751026167303854,-0.109909948718274,
-0.113941135612549));
#34415=CARTESIAN_POINT('Ctrl Pts',(0.748978993560761,0.0125234617264684,
-0.110463148078389));
#34416=CARTESIAN_POINT('Ctrl Pts',(-0.457725546467602,0.599163409431303,
-1.12801069747057));
#34417=CARTESIAN_POINT('Ctrl Pts',(-0.555667179198619,0.524341772031441,
-1.12453270993641));
#34418=CARTESIAN_POINT('Ctrl Pts',(-0.714084824405276,0.325837708337132,
-1.11757673486809));
#34419=CARTESIAN_POINT('Ctrl Pts',(-0.783362670351873,-0.0489378503027571,
-1.1071427722656));
#34420=CARTESIAN_POINT('Ctrl Pts',(-0.66800317241879,-0.412088937642738,
-1.09670880966313));
#34421=CARTESIAN_POINT('Ctrl Pts',(-0.395185257636931,-0.678150527881453,
-1.08627484706064));
#34422=CARTESIAN_POINT('Ctrl Pts',(-0.0292203366733291,-0.784343583971594,
-1.07584088445816));
#34423=CARTESIAN_POINT('Ctrl Pts',(0.343633040095596,-0.705670692032948,
-1.06540692185568));
#34424=CARTESIAN_POINT('Ctrl Pts',(0.635488397768257,-0.460658889708478,
-1.0549729592532));
#34425=CARTESIAN_POINT('Ctrl Pts',(0.777553410767088,-0.10706835061983,
-1.04453899665072));
#34426=CARTESIAN_POINT('Ctrl Pts',(0.736341651251883,0.271760675877957,
-1.03410503404824));
#34427=CARTESIAN_POINT('Ctrl Pts',(0.521567305771499,0.586532409010022,
-1.02367107144576));
#34428=CARTESIAN_POINT('Ctrl Pts',(0.18385461127603,0.763053319515688,-1.01323710884328));
#34429=CARTESIAN_POINT('Ctrl Pts',(-0.197194327096827,0.759715196564627,
-1.0028031462408));
#34430=CARTESIAN_POINT('Ctrl Pts',(-0.531762717152967,0.577305158239884,
-0.992369183638318));
#34431=CARTESIAN_POINT('Ctrl Pts',(-0.740989631772397,0.258818817356289,
-0.981935221035838));
#34432=CARTESIAN_POINT('Ctrl Pts',(-0.775558326712226,-0.120673526448064,
-0.971501258433358));
#34433=CARTESIAN_POINT('Ctrl Pts',(-0.62732063238631,-0.471721998562323,
-0.961067295830877));
#34434=CARTESIAN_POINT('Ctrl Pts',(-0.331217568484232,-0.711581154688748,
-0.950633333228396));
#34435=CARTESIAN_POINT('Ctrl Pts',(0.0429565901738457,-0.783713946820615,
-0.940199370625916));
#34436=CARTESIAN_POINT('Ctrl Pts',(0.407005476575291,-0.671117992759009,
-0.929765408023435));
#34437=CARTESIAN_POINT('Ctrl Pts',(0.67511934619927,-0.400333219873851,
-0.919331445420955));
#34438=CARTESIAN_POINT('Ctrl Pts',(0.784101239483766,-0.0351861433287503,
-0.908897482818473));
#34439=CARTESIAN_POINT('Ctrl Pts',(0.70826309976199,0.338254637741565,-0.898463520215994));
#34440=CARTESIAN_POINT('Ctrl Pts',(0.465480689448243,0.631965621074234,
-0.888029557613512));
#34441=CARTESIAN_POINT('Ctrl Pts',(0.112980104923758,0.776716366722,-0.877595595011032));
#34442=CARTESIAN_POINT('Ctrl Pts',(-0.266150952393824,0.738387763304695,
-0.867161632408551));
#34443=CARTESIAN_POINT('Ctrl Pts',(-0.582547728300971,0.526014222908733,
-0.856727669806071));
#34444=CARTESIAN_POINT('Ctrl Pts',(-0.761632528456596,0.189654185427614,
-0.846293707203591));
#34445=CARTESIAN_POINT('Ctrl Pts',(-0.761193381991245,-0.191409126391062,
-0.835859744601108));
#34446=CARTESIAN_POINT('Ctrl Pts',(-0.581333799855445,-0.527355507791801,
-0.82542578199863));
#34447=CARTESIAN_POINT('Ctrl Pts',(-0.264448376313448,-0.738999238645273,
-0.814991819396148));
#34448=CARTESIAN_POINT('Ctrl Pts',(0.114770015450622,-0.77645390204848,
-0.804557856793668));
#34449=CARTESIAN_POINT('Ctrl Pts',(0.466936035686987,-0.630891081748588,
-0.794123894191188));
#34450=CARTESIAN_POINT('Ctrl Pts',(0.709040842918429,-0.336621302841119,
-0.783689931588707));
#34451=CARTESIAN_POINT('Ctrl Pts',(0.784018058194348,0.0369932815265814,
-0.773255968986227));
#34452=CARTESIAN_POINT('Ctrl Pts',(0.674194847057107,0.401888201686226,
-0.762822006383746));
#34453=CARTESIAN_POINT('Ctrl Pts',(0.405457572755745,0.672054294791692,
-0.752388043781264));
#34454=CARTESIAN_POINT('Ctrl Pts',(0.0411501370855589,0.783810873024088,
-0.741954081178785));
#34455=CARTESIAN_POINT('Ctrl Pts',(-0.332856772724146,0.710815860335577,
-0.731520118576304));
#34456=CARTESIAN_POINT('Ctrl Pts',(-0.628406212210275,0.470274867400413,
-0.721086155973823));
#34457=CARTESIAN_POINT('Ctrl Pts',(-0.775834400197947,0.118885667439072,
-0.710652193371343));
#34458=CARTESIAN_POINT('Ctrl Pts',(-0.74039112689201,-0.260526001912516,
-0.700218230768861));
#34459=CARTESIAN_POINT('Ctrl Pts',(-0.530430704992227,-0.578529243560246,
-0.689784268166382));
#34460=CARTESIAN_POINT('Ctrl Pts',(-0.195442779655914,-0.760167704084639,
-0.6793503055639));
#34461=CARTESIAN_POINT('Ctrl Pts',(0.185612846088945,-0.762627490862808,
-0.668916342961421));
#34462=CARTESIAN_POINT('Ctrl Pts',(0.52291777917247,-0.585328809028116,
-0.658482380358939));
#34463=CARTESIAN_POINT('Ctrl Pts',(0.736966076059816,-0.27006262457056,
-0.648048417756459));
#34464=CARTESIAN_POINT('Ctrl Pts',(0.777304541031368,0.108859859199587,
-0.637614455153979));
#34465=CARTESIAN_POINT('Ctrl Pts',(0.634425018694941,0.462123050828311,
-0.627180492551498));
#34466=CARTESIAN_POINT('Ctrl Pts',(0.342005555592328,0.70645949522738,-0.616746529949017));
#34467=CARTESIAN_POINT('Ctrl Pts',(-0.0310278319582662,0.784276795587446,
-0.606312567346536));
#34468=CARTESIAN_POINT('Ctrl Pts',(-0.396747667841734,0.677232682698558,
-0.595878604744056));
#34469=CARTESIAN_POINT('Ctrl Pts',(-0.668950348821351,0.410558460227938,
-0.585444642141575));
#34470=CARTESIAN_POINT('Ctrl Pts',(-0.783475144171482,0.0471117492608272,
-0.575010679539094));
#34471=CARTESIAN_POINT('Ctrl Pts',(-0.713327483047265,-0.32743964387715,
-0.564576716936614));
#34472=CARTESIAN_POINT('Ctrl Pts',(-0.475041828592946,-0.624810434884062,
-0.554142754334133));
#34473=CARTESIAN_POINT('Ctrl Pts',(-0.12478434954795,-0.774907532910112,
-0.543708791731654));
#34474=CARTESIAN_POINT('Ctrl Pts',(0.254885973710434,-0.742351640975236,
-0.533274829129171));
#34475=CARTESIAN_POINT('Ctrl Pts',(0.574477276930804,-0.534816488847445,
-0.522840866526692));
#34476=CARTESIAN_POINT('Ctrl Pts',(0.758658885652574,-0.201220062800251,
-0.51240690392421));
#34477=CARTESIAN_POINT('Ctrl Pts',(0.764017463316078,0.179805823601479,
-0.501972941321731));
#34478=CARTESIAN_POINT('Ctrl Pts',(0.589289942793166,0.518449787130605,
-0.49153897871925));
#34479=CARTESIAN_POINT('Ctrl Pts',(0.275661243182654,0.734890262188806,
-0.481105016116769));
#34480=CARTESIAN_POINT('Ctrl Pts',(-0.102943402776662,0.778110194174133,
-0.470671053514289));
#34481=CARTESIAN_POINT('Ctrl Pts',(-0.45728332099061,0.637922238832241,
-0.460237090911808));
#34482=CARTESIAN_POINT('Ctrl Pts',(-0.7038372617931,0.347370015062498,-0.449803128309328));
#34483=CARTESIAN_POINT('Ctrl Pts',(-0.78449014362719,-0.0250605866805392,
-0.439369165706847));
#34484=CARTESIAN_POINT('Ctrl Pts',(-0.680231324073692,-0.391584172562934,
-0.428935203104366));
#34485=CARTESIAN_POINT('Ctrl Pts',(-0.415635586978078,-0.665807687917839,
-0.418501240501886));
#34486=CARTESIAN_POINT('Ctrl Pts',(-0.0530706348834358,-0.783094072360267,
-0.408067277899405));
#34487=CARTESIAN_POINT('Ctrl Pts',(0.32200356473851,-0.715797822537027,
-0.397633315296924));
#34488=CARTESIAN_POINT('Ctrl Pts',(0.621178497185401,-0.479781297142652,
-0.387199352694444));
#34489=CARTESIAN_POINT('Ctrl Pts',(0.773935818505536,-0.130675809869565,
-0.376765390091964));
#34490=CARTESIAN_POINT('Ctrl Pts',(0.744269192090715,0.249231194201058,
-0.366331427489482));
#34491=CARTESIAN_POINT('Ctrl Pts',(0.5391713206469,0.57039206291312,-0.355897464887002));
#34492=CARTESIAN_POINT('Ctrl Pts',(0.206985700515677,0.757106160489391,
-0.345463502284521));
#34493=CARTESIAN_POINT('Ctrl Pts',(-0.173988395026941,0.765363218892891,
-0.335029539682041));
#34494=CARTESIAN_POINT('Ctrl Pts',(-0.513951790203906,0.593216971932302,
-0.324595577079561));
#34495=CARTESIAN_POINT('Ctrl Pts',(-0.73277191725422,0.281243908077434,
-0.314161614477079));
#34496=CARTESIAN_POINT('Ctrl Pts',(-0.778870814680853,-0.0970209884795414,
-0.303727651874599));
#34497=CARTESIAN_POINT('Ctrl Pts',(-0.641382540095329,-0.452417126489892,
-0.293293689272119));
#34498=CARTESIAN_POINT('Ctrl Pts',(-0.352714370131861,-0.701174293940717,
-0.282859726669638));
#34499=CARTESIAN_POINT('Ctrl Pts',(0.0190918897513265,-0.784658090821038,
-0.272425764067158));
#34500=CARTESIAN_POINT('Ctrl Pts',(0.386398017223727,-0.683190595956685,
-0.261991801464677));
#34501=CARTESIAN_POINT('Ctrl Pts',(0.662626488959985,-0.420688662481488,
-0.251557838862196));
#34502=CARTESIAN_POINT('Ctrl Pts',(0.782667689483342,-0.0590264425752619,
-0.241123876259716));
#34503=CARTESIAN_POINT('Ctrl Pts',(0.718226716476135,0.316548837101499,
-0.230689913657235));
#34504=CARTESIAN_POINT('Ctrl Pts',(0.484493036851995,0.617510634526485,
-0.220255951054755));
#34505=CARTESIAN_POINT('Ctrl Pts',(0.136559632479492,0.772919263601255,
-0.209821988452274));
#34506=CARTESIAN_POINT('Ctrl Pts',(-0.243561843146319,0.746143766900965,
-0.199388025849793));
#34507=CARTESIAN_POINT('Ctrl Pts',(-0.566274128183446,0.543494756230508,
-0.188954063247312));
#34508=CARTESIAN_POINT('Ctrl Pts',(-0.755509047325738,0.212739737177783,
-0.178520100644832));
#34509=CARTESIAN_POINT('Ctrl Pts',(-0.766665803559577,-0.168161640964725,
-0.168086138042351));
#34510=CARTESIAN_POINT('Ctrl Pts',(-0.597107457561118,-0.509422584813046,
-0.157652175439871));
#34511=CARTESIAN_POINT('Ctrl Pts',(-0.286814649975479,-0.730614045087353,
-0.14721821283739));
#34512=CARTESIAN_POINT('Ctrl Pts',(0.0911015483498663,-0.779580681377717,
-0.13678425023491));
#34513=CARTESIAN_POINT('Ctrl Pts',(0.447507596061844,-0.644816980204478,
-0.126350287632429));
#34514=CARTESIAN_POINT('Ctrl Pts',(0.698507324942248,-0.358015175128559,
-0.115916325029949));
#34515=CARTESIAN_POINT('Ctrl Pts',(0.755950846588162,-0.110628321320819,
-0.108960349961628));
#34516=CARTESIAN_POINT('Ctrl Pts',(0.753890288033488,0.0126055820648028,
-0.105482362427468));
#34517=CARTESIAN_POINT('Ctrl Pts',(-0.459778808448979,0.601851132366393,
-1.12625));
#34518=CARTESIAN_POINT('Ctrl Pts',(-0.558161082255852,0.526692871143935,
-1.12277201246584));
#34519=CARTESIAN_POINT('Ctrl Pts',(-0.717287384517958,0.327300059154954,
-1.11581603739752));
#34520=CARTESIAN_POINT('Ctrl Pts',(-0.786877139371749,-0.0491576947563845,
-1.10538207479504));
#34521=CARTESIAN_POINT('Ctrl Pts',(-0.670999603978842,-0.41393738145968,
-1.09494811219256));
#34522=CARTESIAN_POINT('Ctrl Pts',(-0.396958121390901,-0.681192740453033,
-1.08451414959008));
#34523=CARTESIAN_POINT('Ctrl Pts',(-0.0293513702614931,-0.787862050964758,
-1.0740801869876));
#34524=CARTESIAN_POINT('Ctrl Pts',(0.345174528791177,-0.70883629909999,
-1.06364622438512));
#34525=CARTESIAN_POINT('Ctrl Pts',(0.638339163802789,-0.462725361017625,
-1.05321226178264));
#34526=CARTESIAN_POINT('Ctrl Pts',(0.781041451767081,-0.107548656621832,
-1.04277829918015));
#34527=CARTESIAN_POINT('Ctrl Pts',(0.73964482858492,0.272979776873333,-1.03234433657767));
#34528=CARTESIAN_POINT('Ctrl Pts',(0.523907016570375,0.589163548674701,
-1.02191037397519));
#34529=CARTESIAN_POINT('Ctrl Pts',(0.184679370276391,0.766476320999641,
-1.01147641137271));
#34530=CARTESIAN_POINT('Ctrl Pts',(-0.198078926680871,0.763123222427557,
-1.00104244877023));
#34531=CARTESIAN_POINT('Ctrl Pts',(-0.534148165188284,0.579894906686739,
-0.990608486167751));
#34532=CARTESIAN_POINT('Ctrl Pts',(-0.744313656594542,0.25997985934869,
-0.980174523565271));
#34533=CARTESIAN_POINT('Ctrl Pts',(-0.779037423985492,-0.121214858921561,
-0.969740560962792));
#34534=CARTESIAN_POINT('Ctrl Pts',(-0.630134746400966,-0.473838108603289,
-0.959306598360309));
#34535=CARTESIAN_POINT('Ctrl Pts',(-0.332703386000083,-0.714773255138962,
-0.94887263575783));
#34536=CARTESIAN_POINT('Ctrl Pts',(0.0431492902551158,-0.78722962966257,
-0.938438673155349));
#34537=CARTESIAN_POINT('Ctrl Pts',(0.408831273062274,-0.67412857846459,
-0.928004710552867));
#34538=CARTESIAN_POINT('Ctrl Pts',(0.678147881681892,-0.402129085108458,
-0.917570747950389));
#34539=CARTESIAN_POINT('Ctrl Pts',(0.787618659686819,-0.0353439857660798,
-0.907136785347906));
#34540=CARTESIAN_POINT('Ctrl Pts',(0.711440315674566,0.339772023043393,
-0.896702822745428));
#34541=CARTESIAN_POINT('Ctrl Pts',(0.467568801414539,0.634800572137751,
-0.886268860142945));
#34542=CARTESIAN_POINT('Ctrl Pts',(0.113486925323206,0.78020065893068,-0.875834897540465));
#34543=CARTESIAN_POINT('Ctrl Pts',(-0.267344885893195,0.741700116231729,
-0.865400934937985));
#34544=CARTESIAN_POINT('Ctrl Pts',(-0.585160994350141,0.528373883831427,
-0.854966972335503));
#34545=CARTESIAN_POINT('Ctrl Pts',(-0.765049155681855,0.19050496008484,
-0.844533009733023));
#34546=CARTESIAN_POINT('Ctrl Pts',(-0.764608039237945,-0.192267773583724,
-0.834099047130543));
#34547=CARTESIAN_POINT('Ctrl Pts',(-0.583941620311302,-0.52972118561936,
-0.823665084528062));
#34548=CARTESIAN_POINT('Ctrl Pts',(-0.265634672182434,-0.742314334605435,
-0.813231121925581));
#34549=CARTESIAN_POINT('Ctrl Pts',(0.115284865256511,-0.779937016860141,
-0.802797159323101));
#34550=CARTESIAN_POINT('Ctrl Pts',(0.469030676228697,-0.63372121250791,
-0.79236319672062));
#34551=CARTESIAN_POINT('Ctrl Pts',(0.712221547729785,-0.338131361123721,
-0.781929234118141));
#34552=CARTESIAN_POINT('Ctrl Pts',(0.787535105251363,0.0371592306530875,
-0.771495271515659));
#34553=CARTESIAN_POINT('Ctrl Pts',(0.677219235306731,0.403691042452731,
-0.761061308913179));
#34554=CARTESIAN_POINT('Ctrl Pts',(0.407276425457032,0.675069080682076,
-0.750627346310697));
#34555=CARTESIAN_POINT('Ctrl Pts',(0.0413347335588409,0.787326990663742,
-0.740193383708218));
#34556=CARTESIAN_POINT('Ctrl Pts',(-0.334349943602904,0.714004527743863,
-0.729759421105736));
#34557=CARTESIAN_POINT('Ctrl Pts',(-0.631225196028523,0.472384485694395,
-0.719325458503257));
#34558=CARTESIAN_POINT('Ctrl Pts',(-0.779314735970096,0.119418979755564,
-0.708891495900775));
#34559=CARTESIAN_POINT('Ctrl Pts',(-0.743712466759963,-0.261694702299867,
-0.698457533298295));
#34560=CARTESIAN_POINT('Ctrl Pts',(-0.532810177927122,-0.581124482983871,
-0.688023570695815));
#34561=CARTESIAN_POINT('Ctrl Pts',(-0.19631952151896,-0.763577760216057,
-0.677589608093334));
#34562=CARTESIAN_POINT('Ctrl Pts',(0.186445491596607,-0.766048581415893,
-0.667155645490853));
#34563=CARTESIAN_POINT('Ctrl Pts',(0.525263549677469,-0.587954550799829,
-0.656721682888373));
#34564=CARTESIAN_POINT('Ctrl Pts',(0.740272051402901,-0.271274105542239,
-0.646287720285891));
#34565=CARTESIAN_POINT('Ctrl Pts',(0.780791471746632,0.109348196481392,
-0.635853757683412));
#34566=CARTESIAN_POINT('Ctrl Pts',(0.637271002434187,0.464196100675705,
-0.625419795080931));
#34567=CARTESIAN_POINT('Ctrl Pts',(0.343539767234785,0.709628620303799,
-0.61498583247845));
#34568=CARTESIAN_POINT('Ctrl Pts',(-0.0311670205189552,0.787795003321279,
-0.604551869875969));
#34569=CARTESIAN_POINT('Ctrl Pts',(-0.398527448553385,0.680270698454323,
-0.594117907273489));
#34570=CARTESIAN_POINT('Ctrl Pts',(-0.671951210639545,0.412400195133385,
-0.583683944671008));
#34571=CARTESIAN_POINT('Ctrl Pts',(-0.78698975575632,0.0473230890856653,
-0.573249982068528));
#34572=CARTESIAN_POINT('Ctrl Pts',(-0.716527417409385,-0.328908513916318,
-0.562816019466047));
#34573=CARTESIAN_POINT('Ctrl Pts',(-0.477172831122479,-0.627613288311012,
-0.552382056863567));
#34574=CARTESIAN_POINT('Ctrl Pts',(-0.125344122916371,-0.778383710824121,
-0.541948094261086));
#34575=CARTESIAN_POINT('Ctrl Pts',(0.256029373348162,-0.74568177556445,
-0.531514131658605));
#34576=CARTESIAN_POINT('Ctrl Pts',(0.577054339531638,-0.537215636084532,
-0.521080169056125));
#34577=CARTESIAN_POINT('Ctrl Pts',(0.762062173336032,-0.202122721128445,
-0.510646206453644));
#34578=CARTESIAN_POINT('Ctrl Pts',(0.767444789182847,0.180612419235498,
-0.500212243851163));
#34579=CARTESIAN_POINT('Ctrl Pts',(0.591933453918155,0.520775514553563,
-0.489778281248683));
#34580=CARTESIAN_POINT('Ctrl Pts',(0.276897839143596,0.738186925584305,
-0.479344318646202));
#34581=CARTESIAN_POINT('Ctrl Pts',(-0.103405199272279,0.781600738989841,
-0.468910356043722));
#34582=CARTESIAN_POINT('Ctrl Pts',(-0.459334660167689,0.640783910842521,
-0.458476393441241));
#34583=CARTESIAN_POINT('Ctrl Pts',(-0.706994623724161,0.348928291273615,
-0.448042430838761));
#34584=CARTESIAN_POINT('Ctrl Pts',(-0.78800930842456,-0.0251730066199923,
-0.43760846823628));
#34585=CARTESIAN_POINT('Ctrl Pts',(-0.683282791513017,-0.393340790216431,
-0.4271745056338));
#34586=CARTESIAN_POINT('Ctrl Pts',(-0.417500097498841,-0.668794451991519,
-0.416740543031319));
#34587=CARTESIAN_POINT('Ctrl Pts',(-0.0533087058287156,-0.786606974485123,
-0.406306580428838));
#34588=CARTESIAN_POINT('Ctrl Pts',(0.323448048928478,-0.719008838659509,
-0.395872617826358));
#34589=CARTESIAN_POINT('Ctrl Pts',(0.623965058008296,-0.481933560577751,
-0.385438655223877));
#34590=CARTESIAN_POINT('Ctrl Pts',(0.777407637380551,-0.131262011893554,
-0.375004692621396));
#34591=CARTESIAN_POINT('Ctrl Pts',(0.747607928672497,0.250349226915972,
-0.364570730018916));
#34592=CARTESIAN_POINT('Ctrl Pts',(0.541590003337538,0.572950799545676,
-0.354136767416435));
#34593=CARTESIAN_POINT('Ctrl Pts',(0.207914223068499,0.760502482762855,
-0.343702804813955));
#34594=CARTESIAN_POINT('Ctrl Pts',(-0.174768894106406,0.768796581719083,
-0.333268842211474));
#34595=CARTESIAN_POINT('Ctrl Pts',(-0.516257339945076,0.595878099420955,
-0.322834879608994));
#34596=CARTESIAN_POINT('Ctrl Pts',(-0.736059077911029,0.282505547458041,
-0.312400917006512));
#34597=CARTESIAN_POINT('Ctrl Pts',(-0.782364771583725,-0.0974562174576635,
-0.301966954404033));
#34598=CARTESIAN_POINT('Ctrl Pts',(-0.644259734761709,-0.454446636287429,
-0.291532991801551));
#34599=CARTESIAN_POINT('Ctrl Pts',(-0.354296620723981,-0.704319709976538,
-0.281099029199071));
#34600=CARTESIAN_POINT('Ctrl Pts',(0.0191775345559673,-0.788178009053099,
-0.270665066596591));
#34601=CARTESIAN_POINT('Ctrl Pts',(0.388131370170813,-0.686255338400113,
-0.26023110399411));
#34602=CARTESIAN_POINT('Ctrl Pts',(0.665598982404191,-0.422575840864817,
-0.249797141391629));
#34603=CARTESIAN_POINT('Ctrl Pts',(0.786178678898116,-0.0592912305593806,
-0.239363178789148));
#34604=CARTESIAN_POINT('Ctrl Pts',(0.721448628413702,0.317968851246866,
-0.228929216186668));
#34605=CARTESIAN_POINT('Ctrl Pts',(0.486666436849571,0.620280742650431,
-0.218495253584187));
#34606=CARTESIAN_POINT('Ctrl Pts',(0.137172228805461,0.776386520196726,
-0.208061290981707));
#34607=CARTESIAN_POINT('Ctrl Pts',(-0.24465444339174,0.749490916798135,
-0.197627328379226));
#34608=CARTESIAN_POINT('Ctrl Pts',(-0.568814392418833,0.545932825443553,
-0.187193365776746));
#34609=CARTESIAN_POINT('Ctrl Pts',(-0.758898204371723,0.213694087832844,
-0.176759403174265));
#34610=CARTESIAN_POINT('Ctrl Pts',(-0.770105011053624,-0.16891603298111,
-0.166325440571784));
#34611=CARTESIAN_POINT('Ctrl Pts',(-0.599786034786057,-0.511707755229724,
-0.155891477969304));
#34612=CARTESIAN_POINT('Ctrl Pts',(-0.288101284597239,-0.733891647041663,
-0.145457515366823));
#34613=CARTESIAN_POINT('Ctrl Pts',(0.0915102336223773,-0.783077583290339,
-0.135023552764343));
#34614=CARTESIAN_POINT('Ctrl Pts',(0.449515061170511,-0.64771005951776,
-0.124589590161862));
#34615=CARTESIAN_POINT('Ctrl Pts',(0.701640821699945,-0.35962018580118,
-0.114155627559382));
#34616=CARTESIAN_POINT('Ctrl Pts',(0.759341912736311,-0.111126206723824,
-0.107199652491061));
#34617=CARTESIAN_POINT('Ctrl Pts',(0.757272083693561,0.0126621280946378,
-0.103721664956901));
#34618=CARTESIAN_POINT('Ctrl Pts',(0.555007866453731,-0.51535192480862,
-0.12));
#34619=CARTESIAN_POINT('Ctrl Pts',(0.591072083605958,-0.472049785910246,
-0.12));
#34620=CARTESIAN_POINT('Ctrl Pts',(0.641266713589829,-0.405214104043369,
-0.12));
#34621=CARTESIAN_POINT('Ctrl Pts',(0.703252213124764,-0.26398462653494,
-0.12));
#34622=CARTESIAN_POINT('Ctrl Pts',(0.719761895146736,-0.212714660677395,
-0.12));
#34623=CARTESIAN_POINT('Ctrl Pts',(0.74280866170717,-0.103336683918317,
-0.12));
#34624=CARTESIAN_POINT('Ctrl Pts',(0.748364886323481,-0.0454765203713978,
-0.12));
#34625=CARTESIAN_POINT('Ctrl Pts',(0.747395528060274,0.0124969850565462,
-0.12));
#34626=CARTESIAN_POINT('',(-0.738674446606903,0.114170753859866,-1.12625));
#34627=CARTESIAN_POINT('Ctrl Pts',(-0.738728321778977,0.114178441930237,
-1.12625));
#34628=CARTESIAN_POINT('Ctrl Pts',(-0.729872306490507,0.171476380149586,
-1.12625));
#34629=CARTESIAN_POINT('Ctrl Pts',(-0.714604763127109,0.227558322531749,
-1.12625));
#34630=CARTESIAN_POINT('Ctrl Pts',(-0.673382241080466,0.331452140304365,
-1.12625));
#34631=CARTESIAN_POINT('Ctrl Pts',(-0.648435827358878,0.379185799077542,
-1.12625));
#34632=CARTESIAN_POINT('Ctrl Pts',(-0.563441537104106,0.507894222797761,
-1.12625));
#34633=CARTESIAN_POINT('Ctrl Pts',(-0.50265383037774,0.565275533421068,
-1.12625));
#34634=CARTESIAN_POINT('Ctrl Pts',(-0.459778808448982,0.60185113236639,
-1.12625));
#34635=CARTESIAN_POINT('Ctrl Pts',(-0.738674444793491,0.11417075360109,
-1.12625));
#34636=CARTESIAN_POINT('Ctrl Pts',(-0.744523251396961,0.0764015856923646,
-1.12516243468899));
#34637=CARTESIAN_POINT('Ctrl Pts',(-0.747504748693495,0.0381902463136716,
-1.12407486937799));
#34638=CARTESIAN_POINT('Ctrl Pts',(-0.747536615034749,-1.54000427280091E-5,
-1.12298730406698));
#34639=CARTESIAN_POINT('Origin',(-9.99409214431492E-17,0.,-1.12625));
#34640=CARTESIAN_POINT('',(-0.82685,-1.01259920587499E-16,-1.12625));
#34641=CARTESIAN_POINT('Origin',(0.,0.,-1.12625));
#34642=CARTESIAN_POINT('Origin',(0.,0.,-1.12625));
#34643=CARTESIAN_POINT('',(0.589301091561372,-0.565833523687256,-1.12625));
#34644=CARTESIAN_POINT('Ctrl Pts',(0.82685,-4.02455846426619E-15,-1.12625));
#34645=CARTESIAN_POINT('Ctrl Pts',(0.82685,-0.0640849384885572,-1.12625));
#34646=CARTESIAN_POINT('Ctrl Pts',(0.819177389464161,-0.127972397977404,
-1.12625));
#34647=CARTESIAN_POINT('Ctrl Pts',(0.789918090291955,-0.247778859616483,
-1.12625));
#34648=CARTESIAN_POINT('Ctrl Pts',(0.769494724754842,-0.303642805552845,
-1.12625));
#34649=CARTESIAN_POINT('Ctrl Pts',(0.695180543122701,-0.45245484006238,
-1.12625));
#34650=CARTESIAN_POINT('Ctrl Pts',(0.636182670612352,-0.521654825860832,
-1.12625));
#34651=CARTESIAN_POINT('Ctrl Pts',(0.589301091561372,-0.565833523687256,
-1.12625));
#34652=CARTESIAN_POINT('',(-0.459778808448984,-0.601851132366389,-1.12625));
#34653=CARTESIAN_POINT('Ctrl Pts',(0.589349009255746,-0.565869316348659,
-1.12625));
#34654=CARTESIAN_POINT('Ctrl Pts',(0.561797955794771,-0.591801457111584,
-1.12625));
#34655=CARTESIAN_POINT('Ctrl Pts',(0.53250376759913,-0.615719001693644,
-1.12625));
#34656=CARTESIAN_POINT('Ctrl Pts',(0.50171824497732,-0.637497823098451,
-1.12625));
#34657=CARTESIAN_POINT('Ctrl Pts',(0.47102306597979,-0.659212732070052,
-1.12625));
#34658=CARTESIAN_POINT('Ctrl Pts',(0.438844183868412,-0.678802004601254,
-1.12625));
#34659=CARTESIAN_POINT('Ctrl Pts',(0.405405868387424,-0.696097894311317,
-1.12625));
#34660=CARTESIAN_POINT('Ctrl Pts',(0.394915382569507,-0.701524073324875,
-1.12625));
#34661=CARTESIAN_POINT('Ctrl Pts',(0.384300816323456,-0.706724162922218,
-1.12625));
#34662=CARTESIAN_POINT('Ctrl Pts',(0.373568843076819,-0.71169193771826,
-1.12625));
#34663=CARTESIAN_POINT('Ctrl Pts',(0.363930578232978,-0.716153440562932,
-1.12625));
#34664=CARTESIAN_POINT('Ctrl Pts',(0.354194037388044,-0.720428823536218,
-1.12625));
#34665=CARTESIAN_POINT('Ctrl Pts',(0.344389136277292,-0.724503440483072,
-1.12625));
#34666=CARTESIAN_POINT('Ctrl Pts',(0.319404665564138,-0.734886222178274,
-1.12625));
#34667=CARTESIAN_POINT('Ctrl Pts',(0.293946819978443,-0.74398129459371,
-1.12625));
#34668=CARTESIAN_POINT('Ctrl Pts',(0.268101859965993,-0.751732914379289,
-1.12625));
#34669=CARTESIAN_POINT('Ctrl Pts',(0.236780787659365,-0.76112697200912,
-1.12625));
#34670=CARTESIAN_POINT('Ctrl Pts',(0.204890853635393,-0.768548833828937,
-1.12625));
#34671=CARTESIAN_POINT('Ctrl Pts',(0.172622384826077,-0.773986220742674,
-1.12625));
#34672=CARTESIAN_POINT('Ctrl Pts',(0.153540924365737,-0.777201535482743,
-1.12625));
#34673=CARTESIAN_POINT('Ctrl Pts',(0.134327020168648,-0.779722340056214,
-1.12625));
#34674=CARTESIAN_POINT('Ctrl Pts',(0.115020357875576,-0.781541004368796,
-1.12625));
#34675=CARTESIAN_POINT('Ctrl Pts',(0.103888024742563,-0.782589656729181,
-1.12625));
#34676=CARTESIAN_POINT('Ctrl Pts',(0.0927190764996314,-0.783404877148015,
-1.12625));
#34677=CARTESIAN_POINT('Ctrl Pts',(0.0815541189285967,-0.783983582560309,
-1.12625));
#34678=CARTESIAN_POINT('Ctrl Pts',(0.0448646731867934,-0.78588528085963,
-1.12625));
#34679=CARTESIAN_POINT('Ctrl Pts',(0.00816270548253231,-0.785244764668211,
-1.12625));
#34680=CARTESIAN_POINT('Ctrl Pts',(-0.0282824614483715,-0.782055278068206,
-1.12625));
#34681=CARTESIAN_POINT('Ctrl Pts',(-0.0590932645533356,-0.779358880934808,
-1.12625));
#34682=CARTESIAN_POINT('Ctrl Pts',(-0.0897210642546043,-0.774839835383014,
-1.12625));
#34683=CARTESIAN_POINT('Ctrl Pts',(-0.119998031533345,-0.768465408942048,
-1.12625));
#34684=CARTESIAN_POINT('Ctrl Pts',(-0.136473000057242,-0.764996816001217,
-1.12625));
#34685=CARTESIAN_POINT('Ctrl Pts',(-0.15284394986517,-0.760978380225078,
-1.12625));
#34686=CARTESIAN_POINT('Ctrl Pts',(-0.169085499191771,-0.756419224292495,
-1.12625));
#34687=CARTESIAN_POINT('Ctrl Pts',(-0.177940972575151,-0.753933409472752,
-1.12625));
#34688=CARTESIAN_POINT('Ctrl Pts',(-0.186757956444784,-0.751286813976276,
-1.12625));
#34689=CARTESIAN_POINT('Ctrl Pts',(-0.195532162363131,-0.748480681723287,
-1.12625));
#34690=CARTESIAN_POINT('Ctrl Pts',(-0.202583374992159,-0.746225590451764,
-1.12625));
#34691=CARTESIAN_POINT('Ctrl Pts',(-0.209606136438257,-0.743867596213384,
-1.12625));
#34692=CARTESIAN_POINT('Ctrl Pts',(-0.216586046839137,-0.741412001951311,
-1.12625));
#34693=CARTESIAN_POINT('Ctrl Pts',(-0.250777745045288,-0.72938305987278,
-1.12625));
#34694=CARTESIAN_POINT('Ctrl Pts',(-0.284021591248731,-0.714991447728378,
-1.12625));
#34695=CARTESIAN_POINT('Ctrl Pts',(-0.316082870432815,-0.6983703238303,
-1.12625));
#34696=CARTESIAN_POINT('Ctrl Pts',(-0.347689999419729,-0.681984639281106,
-1.12625));
#34697=CARTESIAN_POINT('Ctrl Pts',(-0.378148790586058,-0.663431461241488,
-1.12625));
#34698=CARTESIAN_POINT('Ctrl Pts',(-0.40720704752916,-0.642797035900976,
-1.12625));
#34699=CARTESIAN_POINT('Ctrl Pts',(-0.42529729927964,-0.629951050339376,
-1.12625));
#34700=CARTESIAN_POINT('Ctrl Pts',(-0.442844152594049,-0.616297659807387,
-1.12625));
#34701=CARTESIAN_POINT('Ctrl Pts',(-0.459778808448986,-0.601851132366388,
-1.12625));
#34702=CARTESIAN_POINT('Ctrl Pts',(-0.459778808448986,-0.601851132366387,
-1.12625));
#34703=CARTESIAN_POINT('Ctrl Pts',(-0.506938887193883,-0.5616200596157,
-1.12625));
#34704=CARTESIAN_POINT('Ctrl Pts',(-0.580457877279435,-0.492400554929899,
-1.12625));
#34705=CARTESIAN_POINT('Ctrl Pts',(-0.691141067841612,-0.302309651856748,
-1.12625));
#34706=CARTESIAN_POINT('Ctrl Pts',(-0.723888788631575,-0.210189415916573,
-1.12625));
#34707=CARTESIAN_POINT('Ctrl Pts',(-0.738728321778978,-0.114178441930233,
-1.12625));
#34708=CARTESIAN_POINT('Origin',(0.,0.,-1.12625));
#34709=CARTESIAN_POINT('Origin',(0.,0.,-1.33003901172249));
#34710=CARTESIAN_POINT('Ctrl Pts',(-0.748490343485035,-0.115687267835002,
-1.1425283350431));
#34711=CARTESIAN_POINT('Ctrl Pts',(-0.72957939383647,-0.238040085590799,
-1.13905034750894));
#34712=CARTESIAN_POINT('Ctrl Pts',(-0.630653629844317,-0.473183377928881,
-1.13209437244062));
#34713=CARTESIAN_POINT('Ctrl Pts',(-0.333406559150428,-0.714445366112161,
-1.12166040983814));
#34714=CARTESIAN_POINT('Ctrl Pts',(0.0423441932323986,-0.787268438306115,
-1.11122644723566));
#34715=CARTESIAN_POINT('Ctrl Pts',(0.408154628293017,-0.674543622261519,
-1.10079248463318));
#34716=CARTESIAN_POINT('Ctrl Pts',(0.677738701453828,-0.402813068451861,
-1.0903585220307));
#34717=CARTESIAN_POINT('Ctrl Pts',(0.787583785039379,-0.0361404951497401,
-1.07992455942821));
#34718=CARTESIAN_POINT('Ctrl Pts',(0.711782686348953,0.339053175380463,
-1.06949059682573));
#34719=CARTESIAN_POINT('Ctrl Pts',(0.468210400798597,0.634327583870302,
-1.05905663422325));
#34720=CARTESIAN_POINT('Ctrl Pts',(0.114275158775038,0.780085648735316,
-1.04862267162077));
#34721=CARTESIAN_POINT('Ctrl Pts',(-0.266595119432202,0.74196987248233,
-1.03818870901829));
#34722=CARTESIAN_POINT('Ctrl Pts',(-0.584626774041373,0.528964985372604,
-1.02775474641581));
#34723=CARTESIAN_POINT('Ctrl Pts',(-0.764856223313065,0.19127799592914,
-1.01732078381333));
#34724=CARTESIAN_POINT('Ctrl Pts',(-0.764801961726996,-0.191494973175329,
-1.00688682121085));
#34725=CARTESIAN_POINT('Ctrl Pts',(-0.584476642087926,-0.529130798350251,
-0.99645285860837));
#34726=CARTESIAN_POINT('Ctrl Pts',(-0.266384707070968,-0.742045509438616,
-0.98601889600589));
#34727=CARTESIAN_POINT('Ctrl Pts',(0.114496619465385,-0.780053123936526,
-0.975584933403408));
#34728=CARTESIAN_POINT('Ctrl Pts',(0.468390010412392,-0.634194881491942,
-0.965150970800929));
#34729=CARTESIAN_POINT('Ctrl Pts',(0.711879475926064,-0.338850945209237,
-0.954717008198448));
#34730=CARTESIAN_POINT('Ctrl Pts',(0.787572255433587,0.0363633449241354,
-0.944283045595968));
#34731=CARTESIAN_POINT('Ctrl Pts',(0.677626851623736,0.403006452460033,
-0.933849082993486));
#34732=CARTESIAN_POINT('Ctrl Pts',(0.407958428506616,0.674657150909495,
-0.923415120391007));
#34733=CARTESIAN_POINT('Ctrl Pts',(0.042130369016677,0.787284816735879,
-0.912981157788525));
#34734=CARTESIAN_POINT('Ctrl Pts',(-0.333628214598003,0.714342050500304,
-0.902547195186045));
#34735=CARTESIAN_POINT('Ctrl Pts',(-0.630747491734475,0.473022147824027,
-0.892113232583564));
#34736=CARTESIAN_POINT('Ctrl Pts',(-0.779193655806613,0.120206478312629,
-0.881679269981084));
#34737=CARTESIAN_POINT('Ctrl Pts',(-0.743976550446063,-0.260942988134434,
-0.871245307378604));
#34738=CARTESIAN_POINT('Ctrl Pts',(-0.533397178462468,-0.58058573930206,
-0.860811344776122));
#34739=CARTESIAN_POINT('Ctrl Pts',(-0.197091077355777,-0.763378973969726,
-0.850377382173643));
#34740=CARTESIAN_POINT('Ctrl Pts',(0.185671243420201,-0.766236608391142,
-0.83994341957116));
#34741=CARTESIAN_POINT('Ctrl Pts',(0.524669106735824,-0.588485071271487,
-0.829509456968682));
#34742=CARTESIAN_POINT('Ctrl Pts',(0.739997529484913,-0.272022070847804,
-0.819075494366199));
#34743=CARTESIAN_POINT('Ctrl Pts',(0.780901578249222,0.108559088795519,
-0.80864153176372));
#34744=CARTESIAN_POINT('Ctrl Pts',(0.637739784219531,0.46355185070908,-0.798207569161239));
#34745=CARTESIAN_POINT('Ctrl Pts',(0.344256728029392,0.709281083829744,
-0.787773606558758));
#34746=CARTESIAN_POINT('Ctrl Pts',(-0.0303708751141343,0.787826097953732,
-0.777339643956278));
#34747=CARTESIAN_POINT('Ctrl Pts',(-0.397839777494349,0.680673094896106,
-0.766905681353797));
#34748=CARTESIAN_POINT('Ctrl Pts',(-0.671534104459313,0.413079044760479,
-0.756471718751317));
#34749=CARTESIAN_POINT('Ctrl Pts',(-0.786941530302541,0.0481183806594935,
-0.746037756148835));
#34750=CARTESIAN_POINT('Ctrl Pts',(-0.716859439874856,-0.32818423809578,
-0.735603793546356));
#34751=CARTESIAN_POINT('Ctrl Pts',(-0.477806840690935,-0.627130746863161,
-0.725169830943874));
#34752=CARTESIAN_POINT('Ctrl Pts',(-0.126130677572575,-0.778256643304304,
-0.714735868341395));
#34753=CARTESIAN_POINT('Ctrl Pts',(0.25527567193062,-0.745940132981574,
-0.704301905738912));
#34754=CARTESIAN_POINT('Ctrl Pts',(0.576511145861978,-0.537798521166717,
-0.693867943136434));
#34755=CARTESIAN_POINT('Ctrl Pts',(0.761857523268443,-0.202892742382455,
-0.683433980533952));
#34756=CARTESIAN_POINT('Ctrl Pts',(0.767626920662054,0.179836763057753,
-0.673000017931472));
#34757=CARTESIAN_POINT('Ctrl Pts',(0.5924594368424,0.520177052904666,-0.662566055328991));
#34758=CARTESIAN_POINT('Ctrl Pts',(0.277643694393179,0.737906721500696,
-0.652132092726511));
#34759=CARTESIAN_POINT('Ctrl Pts',(-0.102615276791043,0.781704839208058,
-0.64169813012403));
#34760=CARTESIAN_POINT('Ctrl Pts',(-0.458686862609216,0.641247777962555,
-0.631264167521549));
#34761=CARTESIAN_POINT('Ctrl Pts',(-0.706641643062577,0.349642587454705,
-0.620830204919069));
#34762=CARTESIAN_POINT('Ctrl Pts',(-0.78803434551991,-0.0243766477023704,
-0.610396242316588));
#34763=CARTESIAN_POINT('Ctrl Pts',(-0.683679944886674,-0.392650077845343,
-0.599962279714107));
#34764=CARTESIAN_POINT('Ctrl Pts',(-0.418175754367012,-0.668372193565666,
-0.589528317111627));
#34765=CARTESIAN_POINT('Ctrl Pts',(-0.0541036075165375,-0.786552700285172,
-0.579094354509147));
#34766=CARTESIAN_POINT('Ctrl Pts',(0.322721268222062,-0.719335341624019,
-0.568660391906665));
#34767=CARTESIAN_POINT('Ctrl Pts',(0.623477707326195,-0.482563880889846,
-0.558226429304185));
#34768=CARTESIAN_POINT('Ctrl Pts',(0.777274589863052,-0.132047577128186,
-0.547792466701704));
#34769=CARTESIAN_POINT('Ctrl Pts',(0.747860544863849,0.24959358186489,-0.537358504099224));
#34770=CARTESIAN_POINT('Ctrl Pts',(0.542168739239194,0.572403187328635,
-0.526924541496743));
#34771=CARTESIAN_POINT('Ctrl Pts',(0.208682665163581,0.760291980710322,
-0.516490578894263));
#34772=CARTESIAN_POINT('Ctrl Pts',(-0.17399187479518,0.768972807176858,
-0.506056616291782));
#34773=CARTESIAN_POINT('Ctrl Pts',(-0.515654894268523,0.596399514326692,
-0.495622653689302));
#34774=CARTESIAN_POINT('Ctrl Pts',(-0.735773207791699,0.283249249545548,
-0.485188691086821));
#34775=CARTESIAN_POINT('Ctrl Pts',(-0.782462859663334,-0.0966655260145846,
-0.47475472848434));
#34776=CARTESIAN_POINT('Ctrl Pts',(-0.64471866003509,-0.453795328396784,
-0.46432076588186));
#34777=CARTESIAN_POINT('Ctrl Pts',(-0.355008211612258,-0.703961306010569,
-0.453886803279379));
#34778=CARTESIAN_POINT('Ctrl Pts',(0.0183810095128271,-0.788196986267641,
-0.443452840676899));
#34779=CARTESIAN_POINT('Ctrl Pts',(0.38743765390661,-0.686647227481269,
-0.433018878074418));
#34780=CARTESIAN_POINT('Ctrl Pts',(0.665171601199011,-0.423248262406725,
-0.422584915471937));
#34781=CARTESIAN_POINT('Ctrl Pts',(0.786118349198421,-0.0600857031737155,
-0.412150952869457));
#34782=CARTESIAN_POINT('Ctrl Pts',(0.721769612451196,0.317239621129978,
-0.401716990266976));
#34783=CARTESIAN_POINT('Ctrl Pts',(0.48729299311423,0.619788584544703,-0.391283027664495));
#34784=CARTESIAN_POINT('Ctrl Pts',(0.137956834542062,0.776247552318673,
-0.380849065062015));
#34785=CARTESIAN_POINT('Ctrl Pts',(-0.24389704678188,0.749737674945354,
-0.370415102459534));
#34786=CARTESIAN_POINT('Ctrl Pts',(-0.568262101448461,0.54650757977013,
-0.359981139857054));
#34787=CARTESIAN_POINT('Ctrl Pts',(-0.758682436896782,0.214460510585722,
-0.349547177254573));
#34788=CARTESIAN_POINT('Ctrl Pts',(-0.770274190049179,-0.168136916847512,
-0.339113214652093));
#34789=CARTESIAN_POINT('Ctrl Pts',(-0.600305075684733,-0.511102892647913,
-0.328679252049612));
#34790=CARTESIAN_POINT('Ctrl Pts',(-0.288838411909729,-0.73359711162755,
-0.318245289447131));
#34791=CARTESIAN_POINT('Ctrl Pts',(0.0907101808452941,-0.783175596150043,
-0.307811326844651));
#34792=CARTESIAN_POINT('Ctrl Pts',(0.448877531081785,-0.648152228766222,
-0.29737736424217));
#34793=CARTESIAN_POINT('Ctrl Pts',(0.70124022796002,-0.360353291538616,
-0.286943401639689));
#34794=CARTESIAN_POINT('Ctrl Pts',(0.78831401046138,0.0123843106225018,
-0.276509439037209));
#34795=CARTESIAN_POINT('Ctrl Pts',(0.689574771586232,0.382202801273025,
-0.266075476434728));
#34796=CARTESIAN_POINT('Ctrl Pts',(0.42829627406239,0.661932524534907,-0.255641513832248));
#34797=CARTESIAN_POINT('Ctrl Pts',(0.0660643238823282,0.785638478676651,
-0.245207551229767));
#34798=CARTESIAN_POINT('Ctrl Pts',(-0.311739618905983,0.724162157724785,
-0.234773588627286));
#34799=CARTESIAN_POINT('Ctrl Pts',(-0.616063582497866,0.491993812660696,
-0.224339626024806));
#34800=CARTESIAN_POINT('Ctrl Pts',(-0.775175608854641,0.143858286910066,
-0.213905663422325));
#34801=CARTESIAN_POINT('Ctrl Pts',(-0.751571377703373,-0.238186748774504,
-0.203471700819845));
#34802=CARTESIAN_POINT('Ctrl Pts',(-0.550814864235531,-0.564087434409687,
-0.193037738217364));
#34803=CARTESIAN_POINT('Ctrl Pts',(-0.220225801435375,-0.757030349608765,
-0.182603775614884));
#34804=CARTESIAN_POINT('Ctrl Pts',(0.162271947040125,-0.771528308468155,
-0.172169813012403));
#34805=CARTESIAN_POINT('Ctrl Pts',(0.50652186418947,-0.604181181458613,
-0.161735850409922));
#34806=CARTESIAN_POINT('Ctrl Pts',(0.731377474710374,-0.294400431622865,
-0.151301887807442));
#34807=CARTESIAN_POINT('Ctrl Pts',(0.783845102655791,0.0847288019872719,
-0.140867925204961));
#34808=CARTESIAN_POINT('Ctrl Pts',(0.651544586453759,0.443977659175325,
-0.130433962602481));
#34809=CARTESIAN_POINT('Ctrl Pts',(0.460967102820801,0.613562143858194,
-0.12347798753416));
#34810=CARTESIAN_POINT('Ctrl Pts',(0.35128376055981,0.670985139773177,-0.12));
#34811=CARTESIAN_POINT('Ctrl Pts',(-0.745983409600527,-0.115299794123061,
-1.14120781194017));
#34812=CARTESIAN_POINT('Ctrl Pts',(-0.727135791628741,-0.237242859367695,
-1.13772982440601));
#34813=CARTESIAN_POINT('Ctrl Pts',(-0.628541377473353,-0.471598508427931,
-1.13077384933769));
#34814=CARTESIAN_POINT('Ctrl Pts',(-0.332289872157584,-0.712052475912534,
-1.12033988673521));
#34815=CARTESIAN_POINT('Ctrl Pts',(0.0422023676689075,-0.784631620439639,
-1.10990592413273));
#34816=CARTESIAN_POINT('Ctrl Pts',(0.406787590016807,-0.672284365610761,
-1.09947196153025));
#34817=CARTESIAN_POINT('Ctrl Pts',(0.675468739687113,-0.401463918278453,
-1.08903799892777));
#34818=CARTESIAN_POINT('Ctrl Pts',(0.784945917892683,-0.036019450074174,
-1.07860403632529));
#34819=CARTESIAN_POINT('Ctrl Pts',(0.709398700781977,0.337917579445235,
-1.06817007372281));
#34820=CARTESIAN_POINT('Ctrl Pts',(0.466642216044095,0.632203019823103,
-1.05773611112033));
#34821=CARTESIAN_POINT('Ctrl Pts',(0.113892415079302,0.777472895144444,
-1.04730214851785));
#34822=CARTESIAN_POINT('Ctrl Pts',(-0.265702207996828,0.739484780514238,
-1.03686818591537));
#34823=CARTESIAN_POINT('Ctrl Pts',(-0.582668673968479,0.527193314268239,
-1.02643422331289));
#34824=CARTESIAN_POINT('Ctrl Pts',(-0.762294477768732,0.190637345373093,
-1.01600026071041));
#34825=CARTESIAN_POINT('Ctrl Pts',(-0.76224039792685,-0.190853595901271,
-1.00556629810792));
#34826=CARTESIAN_POINT('Ctrl Pts',(-0.58251904484713,-0.527358571859844,
-0.995132335505447));
#34827=CARTESIAN_POINT('Ctrl Pts',(-0.265492500386351,-0.739560164195111,
-0.984698372902963));
#34828=CARTESIAN_POINT('Ctrl Pts',(0.114113134053,-0.777440479167041,-0.974264410300485));
#34829=CARTESIAN_POINT('Ctrl Pts',(0.466821224039013,-0.632070762133705,
-0.963830447698002));
#34830=CARTESIAN_POINT('Ctrl Pts',(0.709495166277289,-0.337716026159997,
-0.953396485095523));
#34831=CARTESIAN_POINT('Ctrl Pts',(0.784934426712147,0.036241552574442,
-0.942962522493043));
#34832=CARTESIAN_POINT('Ctrl Pts',(0.675357264853418,0.401656656313797,
-0.932528559890561));
#34833=CARTESIAN_POINT('Ctrl Pts',(0.406592046625541,0.672397510606692,
-0.922094597288082));
#34834=CARTESIAN_POINT('Ctrl Pts',(0.0419892610781143,0.784647950737612,
-0.911660634685599));
#34835=CARTESIAN_POINT('Ctrl Pts',(-0.332510788126124,0.711949492909918,
-0.901226672083121));
#34836=CARTESIAN_POINT('Ctrl Pts',(-0.628634918776022,0.47143784695666,
-0.890792709480638));
#34837=CARTESIAN_POINT('Ctrl Pts',(-0.776583889666874,0.119803868775785,
-0.880358746878159));
#34838=CARTESIAN_POINT('Ctrl Pts',(-0.741484737537109,-0.260069007488211,
-0.869924784275677));
#34839=CARTESIAN_POINT('Ctrl Pts',(-0.531610662510997,-0.578641173926874,
-0.859490821673197));
#34840=CARTESIAN_POINT('Ctrl Pts',(-0.196430956965558,-0.760822176204229,
-0.849056859070717));
#34841=CARTESIAN_POINT('Ctrl Pts',(0.185049371667793,-0.763670239503633,
-0.838622896468236));
#34842=CARTESIAN_POINT('Ctrl Pts',(0.522911823858683,-0.586514048533684,
-0.828188933865755));
#34843=CARTESIAN_POINT('Ctrl Pts',(0.737519043576373,-0.271110982847447,
-0.817754971263275));
#34844=CARTESIAN_POINT('Ctrl Pts',(0.778286091736729,0.108195490052141,
-0.807321008660794));
#34845=CARTESIAN_POINT('Ctrl Pts',(0.63560379186074,0.46199926886376,-0.796887046058315));
#34846=CARTESIAN_POINT('Ctrl Pts',(0.343103703302493,0.70690547701834,-0.786453083455833));
#34847=CARTESIAN_POINT('Ctrl Pts',(-0.0302691534421004,0.785187419033389,
-0.776019120853353));
#34848=CARTESIAN_POINT('Ctrl Pts',(-0.396507286177706,0.678393305293029,
-0.765585158250871));
#34849=CARTESIAN_POINT('Ctrl Pts',(-0.669284924227368,0.411695512315087,
-0.755151195648392));
#34850=CARTESIAN_POINT('Ctrl Pts',(-0.784305814079195,0.0479572169749487,
-0.74471723304591));
#34851=CARTESIAN_POINT('Ctrl Pts',(-0.714458450750784,-0.327085045224027,
-0.734283270443431));
#34852=CARTESIAN_POINT('Ctrl Pts',(-0.47620651437298,-0.625030287527851,
-0.723849307840949));
#34853=CARTESIAN_POINT('Ctrl Pts',(-0.125708226017614,-0.775650015515966,
-0.713415345238469));
#34854=CARTESIAN_POINT('Ctrl Pts',(0.254420672919862,-0.743441743413307,
-0.702981382635988));
#34855=CARTESIAN_POINT('Ctrl Pts',(0.574580227589684,-0.535997263725664,
-0.692547420033508));
#34856=CARTESIAN_POINT('Ctrl Pts',(0.75930582132283,-0.202213190380046,
-0.682113457431026));
#34857=CARTESIAN_POINT('Ctrl Pts',(0.765055895178765,0.17923443282648,-0.671679494828547));
#34858=CARTESIAN_POINT('Ctrl Pts',(0.59047510269656,0.518434815337377,-0.661245532226065));
#34859=CARTESIAN_POINT('Ctrl Pts',(0.276713777796529,0.73543523836976,-0.650811569623586));
#34860=CARTESIAN_POINT('Ctrl Pts',(-0.102271585755068,0.77908666232041,
-0.640377607021104));
#34861=CARTESIAN_POINT('Ctrl Pts',(-0.457150575148634,0.639100036222566,
-0.629943644418625));
#34862=CARTESIAN_POINT('Ctrl Pts',(-0.70427487657359,0.348471523780162,
-0.619509681816143));
#34863=CARTESIAN_POINT('Ctrl Pts',(-0.785394969112564,-0.0242950025948932,
-0.609075719213664));
#34864=CARTESIAN_POINT('Ctrl Pts',(-0.681390084391421,-0.391334968475175,
-0.598641756611182));
#34865=CARTESIAN_POINT('Ctrl Pts',(-0.416775151428224,-0.666133603573932,
-0.588207794008702));
#34866=CARTESIAN_POINT('Ctrl Pts',(-0.0539223974131412,-0.783918286376605,
-0.577773831406221));
#34867=CARTESIAN_POINT('Ctrl Pts',(0.321640372565246,-0.716926059921455,
-0.567339868803741));
#34868=CARTESIAN_POINT('Ctrl Pts',(0.62138948317635,-0.480947621738835,
-0.55690590620126));
#34869=CARTESIAN_POINT('Ctrl Pts',(0.774671251282472,-0.131605308004129,
-0.546471943598779));
#34870=CARTESIAN_POINT('Ctrl Pts',(0.745355723228448,0.248757613971936,
-0.536037980996299));
#34871=CARTESIAN_POINT('Ctrl Pts',(0.540352844554801,0.57048602790949,-0.525604018393818));
#34872=CARTESIAN_POINT('Ctrl Pts',(0.207983720877477,0.757745522262172,
-0.515170055791338));
#34873=CARTESIAN_POINT('Ctrl Pts',(-0.173409120944393,0.766397273893708,
-0.504736093188856));
#34874=CARTESIAN_POINT('Ctrl Pts',(-0.513927802841605,0.594401983614464,
-0.494302130586377));
#34875=CARTESIAN_POINT('Ctrl Pts',(-0.733308870473353,0.282300558170737,
-0.483868167983895));
#34876=CARTESIAN_POINT('Ctrl Pts',(-0.779842143925295,-0.0963417625768395,
-0.473434205381416));
#34877=CARTESIAN_POINT('Ctrl Pts',(-0.642559293212633,-0.452275424232272,
-0.463000242778934));
#34878=CARTESIAN_POINT('Ctrl Pts',(-0.353819176764386,-0.701603516818599,
-0.452566280176454));
#34879=CARTESIAN_POINT('Ctrl Pts',(0.0183194456950479,-0.785557065124962,
-0.442132317573973));
#34880=CARTESIAN_POINT('Ctrl Pts',(0.386140002593756,-0.68434742861757,
-0.431698354971493));
#34881=CARTESIAN_POINT('Ctrl Pts',(0.662943731003984,-0.421830670033247,
-0.421264392369012));
#34882=CARTESIAN_POINT('Ctrl Pts',(0.7834853900691,-0.0598844571388489,
-0.410830429766532));
#34883=CARTESIAN_POINT('Ctrl Pts',(0.719352177605274,0.316177085244017,
-0.400396467164051));
#34884=CARTESIAN_POINT('Ctrl Pts',(0.485660894669788,0.617712716434524,
-0.38996250456157));
#34885=CARTESIAN_POINT('Ctrl Pts',(0.13749477344486,0.773647653611852,-0.37952854195909));
#34886=CARTESIAN_POINT('Ctrl Pts',(-0.243080158387662,0.747226566207262,
-0.369094579356609));
#34887=CARTESIAN_POINT('Ctrl Pts',(-0.566358811836438,0.544677152935719,
-0.358660616754129));
#34888=CARTESIAN_POINT('Ctrl Pts',(-0.756141369320212,0.213742214466813,
-0.348226654151648));
#34889=CARTESIAN_POINT('Ctrl Pts',(-0.767694298022977,-0.167573773103754,
-0.337792691549167));
#34890=CARTESIAN_POINT('Ctrl Pts',(-0.598294464011491,-0.509391047315,-0.327358728946686));
#34891=CARTESIAN_POINT('Ctrl Pts',(-0.28787100066151,-0.731140062743844,
-0.316924766344206));
#34892=CARTESIAN_POINT('Ctrl Pts',(0.0904063637433995,-0.780552493232092,
-0.306490803741726));
#34893=CARTESIAN_POINT('Ctrl Pts',(0.447374098176336,-0.645981361835213,
-0.296056841139245));
#34894=CARTESIAN_POINT('Ctrl Pts',(0.698891552520447,-0.359146354327081,
-0.285622878536764));
#34895=CARTESIAN_POINT('Ctrl Pts',(0.785673697365901,0.0123428316480947,
-0.275188915934284));
#34896=CARTESIAN_POINT('Ctrl Pts',(0.687265167454291,0.380922683136212,
-0.264754953331803));
#34897=CARTESIAN_POINT('Ctrl Pts',(0.42686177429362,0.65971550303675,-0.254320990729322));
#34898=CARTESIAN_POINT('Ctrl Pts',(0.0658430535679694,0.783007126777559,
-0.243887028126842));
#34899=CARTESIAN_POINT('Ctrl Pts',(-0.310695504294148,0.721736709503349,
-0.233453065524361));
#34900=CARTESIAN_POINT('Ctrl Pts',(-0.614000190546954,0.490345969652942,
-0.223019102921881));
#34901=CARTESIAN_POINT('Ctrl Pts',(-0.772579300526886,0.143376460042316,
-0.2125851403194));
#34902=CARTESIAN_POINT('Ctrl Pts',(-0.749054127115351,-0.237388986095505,
-0.20215117771692));
#34903=CARTESIAN_POINT('Ctrl Pts',(-0.548970011334125,-0.562198126842394,
-0.191717215114439));
#34904=CARTESIAN_POINT('Ctrl Pts',(-0.219488194761954,-0.754494815860368,
-0.181283252511959));
#34905=CARTESIAN_POINT('Ctrl Pts',(0.161728445419113,-0.768944215087351,
-0.170849289909478));
#34906=CARTESIAN_POINT('Ctrl Pts',(0.504825365157434,-0.602157589282083,
-0.160415327306997));
#34907=CARTESIAN_POINT('Ctrl Pts',(0.728927854200643,-0.29341438785622,
-0.149981364704517));
#34908=CARTESIAN_POINT('Ctrl Pts',(0.781219769114282,0.0844450113192067,
-0.139547402102036));
#34909=CARTESIAN_POINT('Ctrl Pts',(0.649362332362858,0.442490652619712,
-0.129113439499555));
#34910=CARTESIAN_POINT('Ctrl Pts',(0.459423217828217,0.611507106016669,
-0.122157464431235));
#34911=CARTESIAN_POINT('Ctrl Pts',(0.350107198737617,0.668737795639028,
-0.118679476897075));
#34912=CARTESIAN_POINT('Ctrl Pts',(-0.740853004920359,-0.114506834660721,
-1.13671995863906));
#34913=CARTESIAN_POINT('Ctrl Pts',(-0.722134886980705,-0.235612041726607,
-1.1332419711049));
#34914=CARTESIAN_POINT('Ctrl Pts',(-0.624218812318237,-0.468354692822251,
-1.12628599603658));
#34915=CARTESIAN_POINT('Ctrl Pts',(-0.330004563367695,-0.707155702503664,
-1.1158520334341));
#34916=CARTESIAN_POINT('Ctrl Pts',(0.0419121041683271,-0.779235354142126,
-1.10541807083161));
#34917=CARTESIAN_POINT('Ctrl Pts',(0.40399000002701,-0.667660918672005,
-1.09498410822914));
#34918=CARTESIAN_POINT('Ctrl Pts',(0.670823328245096,-0.398702898627244,
-1.08455014562665));
#34919=CARTESIAN_POINT('Ctrl Pts',(0.779547608102049,-0.0357717483197776,
-1.07411618302417));
#34920=CARTESIAN_POINT('Ctrl Pts',(0.704519947383164,0.335593624574011,
-1.06368222042169));
#34921=CARTESIAN_POINT('Ctrl Pts',(0.463432975704643,0.627855162501341,
-1.05324825781921));
#34922=CARTESIAN_POINT('Ctrl Pts',(0.113109141693867,0.772125978326591,
-1.04281429521673));
#34923=CARTESIAN_POINT('Ctrl Pts',(-0.26387489246471,0.734399116602389,
-1.03238033261425));
#34924=CARTESIAN_POINT('Ctrl Pts',(-0.578661483474972,0.523567645181706,
-1.02194637001177));
#34925=CARTESIAN_POINT('Ctrl Pts',(-0.757051945540773,0.189326273808813,
-1.01151240740929));
#34926=CARTESIAN_POINT('Ctrl Pts',(-0.756998237707173,-0.18954103724319,
-1.00107844480681));
#34927=CARTESIAN_POINT('Ctrl Pts',(-0.578512883273854,-0.523731765804213,
-0.99064448220433));
#34928=CARTESIAN_POINT('Ctrl Pts',(-0.263666627302358,-0.734473982814123,
-0.980210519601847));
#34929=CARTESIAN_POINT('Ctrl Pts',(0.113328343147265,-0.772093783330432,
-0.969776556999367));
#34930=CARTESIAN_POINT('Ctrl Pts',(0.463610751763097,-0.627723818257463,
-0.959342594396887));
#34931=CARTESIAN_POINT('Ctrl Pts',(0.704615751113342,-0.335393449806213,
-0.948908631794406));
#34932=CARTESIAN_POINT('Ctrl Pts',(0.779536192689487,0.0359923083399053,
-0.938474669191926));
#34933=CARTESIAN_POINT('Ctrl Pts',(0.670712626473464,0.398894340692951,
-0.928040706589444));
#34934=CARTESIAN_POINT('Ctrl Pts',(0.403795788817699,0.66777322736188,-0.917606743986965));
#34935=CARTESIAN_POINT('Ctrl Pts',(0.0417004880928141,0.779251686898004,
-0.907172781384483));
#34936=CARTESIAN_POINT('Ctrl Pts',(-0.33022400978122,0.707053198590567,
-0.896738818782004));
#34937=CARTESIAN_POINT('Ctrl Pts',(-0.624311604253702,0.468195624755374,
-0.886304856179521));
#34938=CARTESIAN_POINT('Ctrl Pts',(-0.771243084840896,0.118979940943888,
-0.875870893577043));
#34939=CARTESIAN_POINT('Ctrl Pts',(-0.736385320310804,-0.258280433415597,
-0.865436930974559));
#34940=CARTESIAN_POINT('Ctrl Pts',(-0.527954613461226,-0.574661681671945,
-0.855002968372082));
#34941=CARTESIAN_POINT('Ctrl Pts',(-0.195080041221753,-0.755589769500391,
-0.844569005769599));
#34942=CARTESIAN_POINT('Ctrl Pts',(0.183776730565653,-0.758418245797768,
-0.83413504316712));
#34943=CARTESIAN_POINT('Ctrl Pts',(0.519315599381725,-0.582480412113205,
-0.823701080564639));
#34944=CARTESIAN_POINT('Ctrl Pts',(0.73244689963983,-0.269246469734522,
-0.813267117962159));
#34945=CARTESIAN_POINT('Ctrl Pts',(0.772933580346709,0.107451396589594,
-0.802833155359677));
#34946=CARTESIAN_POINT('Ctrl Pts',(0.631232550267715,0.458821958649651,
-0.792399192757197));
#34947=CARTESIAN_POINT('Ctrl Pts',(0.340744074241428,0.702043871938179,
-0.781965230154717));
#34948=CARTESIAN_POINT('Ctrl Pts',(-0.0300609832200121,0.779787445105681,
-0.771531267552235));
#34949=CARTESIAN_POINT('Ctrl Pts',(-0.393780384350698,0.673727787134545,
-0.761097304949757));
#34950=CARTESIAN_POINT('Ctrl Pts',(-0.664682047190082,0.408864156413597,
-0.750663342347273));
#34951=CARTESIAN_POINT('Ctrl Pts',(-0.778911903218281,0.047627400532361,
-0.740229379744795));
#34952=CARTESIAN_POINT('Ctrl Pts',(-0.709544901561173,-0.324835581371782,
-0.729795417142313));
#34953=CARTESIAN_POINT('Ctrl Pts',(-0.472931496588075,-0.620731763156647,
-0.719361454539833));
#34954=CARTESIAN_POINT('Ctrl Pts',(-0.124843692115849,-0.770315633228017,
-0.708927491937352));
#34955=CARTESIAN_POINT('Ctrl Pts',(0.252670944170861,-0.738328867259302,
-0.698493529334872));
#34956=CARTESIAN_POINT('Ctrl Pts',(0.570628663704237,-0.532311046678269,
-0.688059566732391));
#34957=CARTESIAN_POINT('Ctrl Pts',(0.754083843055084,-0.20082250844931,
-0.677625604129911));
#34958=CARTESIAN_POINT('Ctrl Pts',(0.759794371895204,0.178001782836491,
-0.667191641527429));
#34959=CARTESIAN_POINT('Ctrl Pts',(0.586414224895629,0.51486938061673,-0.65675767892495));
#34960=CARTESIAN_POINT('Ctrl Pts',(0.274810732549857,0.730377425398683,
-0.646323716322469));
#34961=CARTESIAN_POINT('Ctrl Pts',(-0.101568232793424,0.773728645161738,
-0.635889753719988));
#34962=CARTESIAN_POINT('Ctrl Pts',(-0.454006610883545,0.634704749888194,
-0.625455791117507));
#34963=CARTESIAN_POINT('Ctrl Pts',(-0.699431362936911,0.346074978576626,
-0.615021828515027));
#34964=CARTESIAN_POINT('Ctrl Pts',(-0.779993567799511,-0.0241279184345948,
-0.604587865912546));
#34965=CARTESIAN_POINT('Ctrl Pts',(-0.676703956466903,-0.388643638258286,
-0.594153903310066));
#34966=CARTESIAN_POINT('Ctrl Pts',(-0.41390886129561,-0.661552399132199,
-0.583719940707585));
#34967=CARTESIAN_POINT('Ctrl Pts',(-0.053551556601009,-0.778527040662177,
-0.573285978105104));
#34968=CARTESIAN_POINT('Ctrl Pts',(0.319428353391418,-0.711995540229181,
-0.562852015502625));
#34969=CARTESIAN_POINT('Ctrl Pts',(0.617115997729736,-0.477639997909126,
-0.552418052900142));
#34970=CARTESIAN_POINT('Ctrl Pts',(0.769343600255384,-0.130700218066691,
-0.541984090297663));
#34971=CARTESIAN_POINT('Ctrl Pts',(0.740229684050112,0.247046831810627,
-0.531550127695182));
#34972=CARTESIAN_POINT('Ctrl Pts',(0.536636672846459,0.566562621086918,
-0.521116165092702));
#34973=CARTESIAN_POINT('Ctrl Pts',(0.206553353244347,0.752534274648081,
-0.51068220249022));
#34974=CARTESIAN_POINT('Ctrl Pts',(-0.172216533405129,0.761126525538637,
-0.500248239887741));
#34975=CARTESIAN_POINT('Ctrl Pts',(-0.510393364223772,0.59031409945294,
-0.489814277285259));
#34976=CARTESIAN_POINT('Ctrl Pts',(-0.728265681184372,0.280359090927444,
-0.479380314682779));
#34977=CARTESIAN_POINT('Ctrl Pts',(-0.77447893108866,-0.0956791908220543,
-0.468946352080298));
#34978=CARTESIAN_POINT('Ctrl Pts',(-0.638140216510379,-0.449164987870463,
-0.458512389477818));
#34979=CARTESIAN_POINT('Ctrl Pts',(-0.351385854116396,-0.696778374939642,
-0.448078426875337));
#34980=CARTESIAN_POINT('Ctrl Pts',(0.0181934572663925,-0.780154549028075,
-0.437644464272857));
#34981=CARTESIAN_POINT('Ctrl Pts',(0.383484399745436,-0.679640962132693,
-0.427210501670376));
#34982=CARTESIAN_POINT('Ctrl Pts',(0.658384464291117,-0.418929611553615,
-0.416776539067896));
#34983=CARTESIAN_POINT('Ctrl Pts',(0.778097121514928,-0.0594726134192682,
-0.406342576465414));
#34984=CARTESIAN_POINT('Ctrl Pts',(0.714404972759968,0.314002638767335,
-0.395908613862934));
#34985=CARTESIAN_POINT('Ctrl Pts',(0.482320856221212,0.613464517236842,
-0.385474651260454));
#34986=CARTESIAN_POINT('Ctrl Pts',(0.136549179853027,0.768327042178898,
-0.375040688657973));
#34987=CARTESIAN_POINT('Ctrl Pts',(-0.241408421824046,0.74208766066977,
-0.364606726055492));
#34988=CARTESIAN_POINT('Ctrl Pts',(-0.562463789140705,0.540931241636695,
-0.354172763453012));
#34989=CARTESIAN_POINT('Ctrl Pts',(-0.750941153956061,0.21227224391263,
-0.343738800850531));
#34990=CARTESIAN_POINT('Ctrl Pts',(-0.762414629636959,-0.166421317035261,
-0.333304838248051));
#34991=CARTESIAN_POINT('Ctrl Pts',(-0.59417981007126,-0.505887809352505,
-0.32287087564557));
#34992=CARTESIAN_POINT('Ctrl Pts',(-0.2858912237842,-0.726111789007469,
-0.312436913043089));
#34993=CARTESIAN_POINT('Ctrl Pts',(0.0897846115448619,-0.77518439510846,
-0.302002950440609));
#34994=CARTESIAN_POINT('Ctrl Pts',(0.444297369724562,-0.641538750516217,
-0.291568987838128));
#34995=CARTESIAN_POINT('Ctrl Pts',(0.694085061664183,-0.356676395059487,
-0.281135025235648));
#34996=CARTESIAN_POINT('Ctrl Pts',(0.780270379123696,0.0122579462393452,
-0.270701062633167));
#34997=CARTESIAN_POINT('Ctrl Pts',(0.682538634845947,0.378302961353538,
-0.260267100030687));
#34998=CARTESIAN_POINT('Ctrl Pts',(0.423926115256723,0.655178437904007,
-0.249833137428206));
#34999=CARTESIAN_POINT('Ctrl Pts',(0.0653902309856967,0.777622147249573,
-0.239399174825725));
#35000=CARTESIAN_POINT('Ctrl Pts',(-0.308558756771405,0.716773105772152,
-0.228965212223245));
#35001=CARTESIAN_POINT('Ctrl Pts',(-0.60977752264731,0.486973709982111,
-0.218531249620764));
#35002=CARTESIAN_POINT('Ctrl Pts',(-0.767266038211421,0.142390417335117,
-0.208097287018284));
#35003=CARTESIAN_POINT('Ctrl Pts',(-0.743902649484968,-0.235756391513122,
-0.197663324415803));
#35004=CARTESIAN_POINT('Ctrl Pts',(-0.545194583421681,-0.558331714416402,
-0.187229361813323));
#35005=CARTESIAN_POINT('Ctrl Pts',(-0.217978694187387,-0.749305932283897,
-0.176795399210842));
#35006=CARTESIAN_POINT('Ctrl Pts',(0.160616163563403,-0.763655935021635,
-0.166361436608361));
#35007=CARTESIAN_POINT('Ctrl Pts',(0.501353577761108,-0.59801639819482,
-0.155927474005881));
#35008=CARTESIAN_POINT('Ctrl Pts',(0.723914693935939,-0.291396426753068,
-0.1454935114034));
#35009=CARTESIAN_POINT('Ctrl Pts',(0.775847282725173,0.0838641360470627,
-0.135059548800919));
#35010=CARTESIAN_POINT('Ctrl Pts',(0.644896041046783,0.439447767297551,
-0.124625586198439));
#35011=CARTESIAN_POINT('Ctrl Pts',(0.45626430167519,0.607301174227473,-0.117669611130118));
#35012=CARTESIAN_POINT('Ctrl Pts',(0.347699381636261,0.66413863770549,-0.114191623595958));
#35013=CARTESIAN_POINT('Ctrl Pts',(-0.738728321778978,-0.114178441930233,
-1.13006310830201));
#35014=CARTESIAN_POINT('Ctrl Pts',(-0.720064366806754,-0.234933217536769,
-1.12658512076785));
#35015=CARTESIAN_POINT('Ctrl Pts',(-0.622428042508284,-0.467013310191975,
-1.11962914569953));
#35016=CARTESIAN_POINT('Ctrl Pts',(-0.329058258071164,-0.705126571760288,
-1.10919518309705));
#35017=CARTESIAN_POINT('Ctrl Pts',(0.0417919924060089,-0.777000845426073,
-1.09876122049457));
#35018=CARTESIAN_POINT('Ctrl Pts',(0.402831247473459,-0.66574573944522,
-1.08832725789209));
#35019=CARTESIAN_POINT('Ctrl Pts',(0.668899333621666,-0.39755947669164,
-1.0778932952896));
#35020=CARTESIAN_POINT('Ctrl Pts',(0.777311738081329,-0.0356690904367907,
-1.06745933268712));
#35021=CARTESIAN_POINT('Ctrl Pts',(0.702499287124512,0.334631062607015,
-1.05702537008464));
#35022=CARTESIAN_POINT('Ctrl Pts',(0.462103778469495,0.626054396882013,
-1.04659140748216));
#35023=CARTESIAN_POINT('Ctrl Pts',(0.112784729733038,0.769911399718677,
-1.03615744487968));
#35024=CARTESIAN_POINT('Ctrl Pts',(-0.263118061333202,0.73229275590801,
-1.0257234822772));
#35025=CARTESIAN_POINT('Ctrl Pts',(-0.577001796823257,0.522065974186607,
-1.01528951967472));
#35026=CARTESIAN_POINT('Ctrl Pts',(-0.754880609472423,0.188783259239166,
-1.00485555707224));
#35027=CARTESIAN_POINT('Ctrl Pts',(-0.754827055346662,-0.188997406198555,
-0.994421594469758));
#35028=CARTESIAN_POINT('Ctrl Pts',(-0.576853623322529,-0.522229625831565,
-0.98398763186728));
#35029=CARTESIAN_POINT('Ctrl Pts',(-0.262910392619021,-0.732367403574915,
-0.973553669264797));
#35030=CARTESIAN_POINT('Ctrl Pts',(0.113003300781567,-0.769879304770086,
-0.963119706662317));
#35031=CARTESIAN_POINT('Ctrl Pts',(0.462281047969412,-0.625923414086446,
-0.952685744059838));
#35032=CARTESIAN_POINT('Ctrl Pts',(0.702594809534997,-0.334431492061369,
-0.942251781457356));
#35033=CARTESIAN_POINT('Ctrl Pts',(0.777300368274831,0.0358890770986708,
-0.931817818854876));
#35034=CARTESIAN_POINT('Ctrl Pts',(0.668788924044225,0.397750253078562,
-0.921383856252395));
#35035=CARTESIAN_POINT('Ctrl Pts',(0.402637643125386,0.665857955560156,
-0.910949893649915));
#35036=CARTESIAN_POINT('Ctrl Pts',(0.0415808849614458,0.777016678487022,
-0.900515931047433));
#35037=CARTESIAN_POINT('Ctrl Pts',(-0.329276878767882,0.705025266057697,
-0.890081968444954));
#35038=CARTESIAN_POINT('Ctrl Pts',(-0.622520986779629,0.466852770864623,
-0.879648005842472));
#35039=CARTESIAN_POINT('Ctrl Pts',(-0.76903104627692,0.118638688979371,
-0.869214043239993));
#35040=CARTESIAN_POINT('Ctrl Pts',(-0.734273258940723,-0.25753964715726,
-0.858780080637511));
#35041=CARTESIAN_POINT('Ctrl Pts',(-0.526440362004133,-0.573013467475887,
-0.848346118035031));
#35042=CARTESIAN_POINT('Ctrl Pts',(-0.194520522980727,-0.753422626946348,
-0.837912155432551));
#35043=CARTESIAN_POINT('Ctrl Pts',(0.183249631881523,-0.756242990757862,
-0.82747819283007));
#35044=CARTESIAN_POINT('Ctrl Pts',(0.517826125887222,-0.5808097726486,-0.81704423022759));
#35045=CARTESIAN_POINT('Ctrl Pts',(0.730346134239288,-0.268474231271757,
-0.806610267625109));
#35046=CARTESIAN_POINT('Ctrl Pts',(0.770716693193102,0.107143210185493,
-0.796176305022628));
#35047=CARTESIAN_POINT('Ctrl Pts',(0.629422082502815,0.457505989811206,
-0.785742342420148));
#35048=CARTESIAN_POINT('Ctrl Pts',(0.339766770136572,0.700030306891271,
-0.775308379817667));
#35049=CARTESIAN_POINT('Ctrl Pts',(-0.0299747639002413,0.777550900060215,
-0.764874417215186));
#35050=CARTESIAN_POINT('Ctrl Pts',(-0.392650964310469,0.671795436782195,
-0.754440454612705));
#35051=CARTESIAN_POINT('Ctrl Pts',(-0.662775641349895,0.407691473897311,
-0.744006492010225));
#35052=CARTESIAN_POINT('Ctrl Pts',(-0.77667786935568,0.0474907981449312,
-0.733572529407744));
#35053=CARTESIAN_POINT('Ctrl Pts',(-0.707509822458421,-0.323903905163518,
-0.723138566805264));
#35054=CARTESIAN_POINT('Ctrl Pts',(-0.471575059520285,-0.618951413193123,
-0.712704604202783));
#35055=CARTESIAN_POINT('Ctrl Pts',(-0.124485622050972,-0.768106254731665,
-0.702270641600303));
#35056=CARTESIAN_POINT('Ctrl Pts',(0.251946246752525,-0.736211231510794,
-0.691836678997822));
#35057=CARTESIAN_POINT('Ctrl Pts',(0.568992016796649,-0.530784300330188,
-0.681402716395341));
#35058=CARTESIAN_POINT('Ctrl Pts',(0.751921019719524,-0.200246519967949,
-0.670968753792861));
#35059=CARTESIAN_POINT('Ctrl Pts',(0.757615169923306,0.177491247551542,
-0.66053479119038));
#35060=CARTESIAN_POINT('Ctrl Pts',(0.584732302677578,0.513392659531377,
-0.650100828587899));
#35061=CARTESIAN_POINT('Ctrl Pts',(0.274022534963215,0.728282595554539,
-0.639666865985419));
#35062=CARTESIAN_POINT('Ctrl Pts',(-0.101276920168097,0.771509477645342,
-0.629232903382938));
#35063=CARTESIAN_POINT('Ctrl Pts',(-0.452704453170499,0.632884323344261,
-0.618798940780458));
#35064=CARTESIAN_POINT('Ctrl Pts',(-0.697425290949937,0.345082384654329,
-0.608364978177976));
#35065=CARTESIAN_POINT('Ctrl Pts',(-0.777756431563853,-0.0240587160169735,
-0.597931015575498));
#35066=CARTESIAN_POINT('Ctrl Pts',(-0.674763070023318,-0.38752895116111,
-0.587497052973015));
#35067=CARTESIAN_POINT('Ctrl Pts',(-0.412721709823994,-0.659654969582799,
-0.577063090370536));
#35068=CARTESIAN_POINT('Ctrl Pts',(-0.0533979628629402,-0.776294110641973,
-0.566629127768054));
#35069=CARTESIAN_POINT('Ctrl Pts',(0.318512185908032,-0.709953432334411,
-0.556195165165574));
#35070=CARTESIAN_POINT('Ctrl Pts',(0.615346018313083,-0.476270056167252,
-0.545761202563093));
#35071=CARTESIAN_POINT('Ctrl Pts',(0.767137009692518,-0.130325350624296,
-0.535327239960613));
#35072=CARTESIAN_POINT('Ctrl Pts',(0.738106596479569,0.246338265173459,
-0.524893277358132));
#35073=CARTESIAN_POINT('Ctrl Pts',(0.535097519966526,0.564937636187391,
-0.514459314755652));
#35074=CARTESIAN_POINT('Ctrl Pts',(0.205960927857503,0.750375895702546,
-0.504025352153171));
#35075=CARTESIAN_POINT('Ctrl Pts',(-0.171722591066159,0.758943502754224,
-0.49359138955069));
#35076=CARTESIAN_POINT('Ctrl Pts',(-0.508929481011548,0.588620991821254,
-0.48315742694821));
#35077=CARTESIAN_POINT('Ctrl Pts',(-0.726176908133127,0.279554979833196,
-0.47272346434573));
#35078=CARTESIAN_POINT('Ctrl Pts',(-0.772257611641912,-0.0954047688349727,
-0.462289501743249));
#35079=CARTESIAN_POINT('Ctrl Pts',(-0.636309936543053,-0.447876716644087,
-0.451855539140769));
#35080=CARTESIAN_POINT('Ctrl Pts',(-0.350378027822189,-0.694779912112316,
-0.441421576538287));
#35081=CARTESIAN_POINT('Ctrl Pts',(0.0181412757559533,-0.777916951074585,
-0.430987613935807));
#35082=CARTESIAN_POINT('Ctrl Pts',(0.382384510102879,-0.677691651925025,
-0.420553651333326));
#35083=CARTESIAN_POINT('Ctrl Pts',(0.656496120844634,-0.417728059832058,
-0.410119688730846));
#35084=CARTESIAN_POINT('Ctrl Pts',(0.775865424566033,-0.059302037219655,
-0.399685726128365));
#35085=CARTESIAN_POINT('Ctrl Pts',(0.712355954258472,0.313102033031217,
-0.389251763525884));
#35086=CARTESIAN_POINT('Ctrl Pts',(0.480937489089399,0.611705010803167,
-0.378817800923404));
#35087=CARTESIAN_POINT('Ctrl Pts',(0.136157536728385,0.76612336725398,-0.368383838320924));
#35088=CARTESIAN_POINT('Ctrl Pts',(-0.240716026976006,0.739959244149261,
-0.357949875718442));
#35089=CARTESIAN_POINT('Ctrl Pts',(-0.560850560293331,0.539379771301723,
-0.347515913115962));
#35090=CARTESIAN_POINT('Ctrl Pts',(-0.748787344315938,0.211663415907114,
-0.337081950513481));
#35091=CARTESIAN_POINT('Ctrl Pts',(-0.760227912378577,-0.165943996230135,
-0.326647987911001));
#35092=CARTESIAN_POINT('Ctrl Pts',(-0.592475615017121,-0.504436848731709,
-0.316214025308521));
#35093=CARTESIAN_POINT('Ctrl Pts',(-0.285071245711697,-0.724029193640397,
-0.30578006270604));
#35094=CARTESIAN_POINT('Ctrl Pts',(0.0895270960624317,-0.772961052277889,
-0.295346100103559));
#35095=CARTESIAN_POINT('Ctrl Pts',(0.443023059573026,-0.639698723071951,
-0.284912137501079));
#35096=CARTESIAN_POINT('Ctrl Pts',(0.692094323595697,-0.355653394680012,
-0.274478174898598));
#35097=CARTESIAN_POINT('Ctrl Pts',(0.77803244906981,0.0122227885764535,
-0.264044212296118));
#35098=CARTESIAN_POINT('Ctrl Pts',(0.680581013455972,0.377217932977406,
-0.253610249693636));
#35099=CARTESIAN_POINT('Ctrl Pts',(0.422710233282305,0.653299289538504,
-0.243176287091156));
#35100=CARTESIAN_POINT('Ctrl Pts',(0.0652026812946639,0.775391813136047,
-0.232742324488675));
#35101=CARTESIAN_POINT('Ctrl Pts',(-0.307673763129735,0.714717294055676,
-0.222308361886195));
#35102=CARTESIAN_POINT('Ctrl Pts',(-0.608028594518627,0.485576999870044,
-0.211874399283715));
#35103=CARTESIAN_POINT('Ctrl Pts',(-0.765065399588571,0.141982016572898,
-0.201440436681234));
#35104=CARTESIAN_POINT('Ctrl Pts',(-0.741769040716881,-0.235080199432113,
-0.191006474078753));
#35105=CARTESIAN_POINT('Ctrl Pts',(-0.543630858812939,-0.556730352880329,
-0.180572511476273));
#35106=CARTESIAN_POINT('Ctrl Pts',(-0.217353551159869,-0.747156781385138,
-0.170138548873792));
#35107=CARTESIAN_POINT('Ctrl Pts',(0.16015559496067,-0.761465719142782,
-0.159704586271311));
#35108=CARTESIAN_POINT('Ctrl Pts',(0.499915420847107,-0.596301077920999,
-0.149270623668831));
#35109=CARTESIAN_POINT('Ctrl Pts',(0.721838796965714,-0.290560898293607,
-0.13883666106635));
#35110=CARTESIAN_POINT('Ctrl Pts',(0.773621246330564,0.0836240792666152,
-0.12840269846387));
#35111=CARTESIAN_POINT('Ctrl Pts',(0.643048073335996,0.438186347774578,
-0.117968735861389));
#35112=CARTESIAN_POINT('Ctrl Pts',(0.454952994195837,0.605560964824544,
-0.111012760793069));
#35113=CARTESIAN_POINT('Ctrl Pts',(0.346702218893416,0.662233962746084,
-0.107534773258908));
#35114=CARTESIAN_POINT('Ctrl Pts',(-0.738728321778978,-0.114178441930233,
-1.12625));
#35115=CARTESIAN_POINT('Ctrl Pts',(-0.720064014057805,-0.23493549980332,
-1.12277201246584));
#35116=CARTESIAN_POINT('Ctrl Pts',(-0.622428467720143,-0.467011987146764,
-1.11581603739752));
#35117=CARTESIAN_POINT('Ctrl Pts',(-0.329058176975965,-0.705127368582219,
-1.10538207479504));
#35118=CARTESIAN_POINT('Ctrl Pts',(0.0417919283474094,-0.777000661774149,
-1.09494811219256));
#35119=CARTESIAN_POINT('Ctrl Pts',(0.402831360764579,-0.665746034504356,
-1.08451414959008));
#35120=CARTESIAN_POINT('Ctrl Pts',(0.668899442574653,-0.397559467050135,
-1.0740801869876));
#35121=CARTESIAN_POINT('Ctrl Pts',(0.777311895666571,-0.0356691406410416,
-1.06364622438512));
#35122=CARTESIAN_POINT('Ctrl Pts',(0.702499416237836,0.334631148448012,
-1.05321226178264));
#35123=CARTESIAN_POINT('Ctrl Pts',(0.46210386898375,0.626054505003765,-1.04277829918015));
#35124=CARTESIAN_POINT('Ctrl Pts',(0.112784749994036,0.769911552166375,
-1.03234433657768));
#35125=CARTESIAN_POINT('Ctrl Pts',(-0.26311811085717,0.732292892594134,
-1.02191037397519));
#35126=CARTESIAN_POINT('Ctrl Pts',(-0.577001907123836,0.522066075167687,
-1.01147641137271));
#35127=CARTESIAN_POINT('Ctrl Pts',(-0.75488075319647,0.188783294475201,
-1.00104244877023));
#35128=CARTESIAN_POINT('Ctrl Pts',(-0.754827199305277,-0.188997441843081,
-0.990608486167751));
#35129=CARTESIAN_POINT('Ctrl Pts',(-0.576853733233578,-0.522229725565815,
-0.980174523565273));
#35130=CARTESIAN_POINT('Ctrl Pts',(-0.262910442753167,-0.732367543071951,
-0.969740560962789));
#35131=CARTESIAN_POINT('Ctrl Pts',(0.113003322331734,-0.769879451565163,
-0.959306598360312));
#35132=CARTESIAN_POINT('Ctrl Pts',(0.462281136078415,-0.62592353336717,
-0.948872635757828));
#35133=CARTESIAN_POINT('Ctrl Pts',(0.702594943458043,-0.334431555819591,
-0.938438673155349));
#35134=CARTESIAN_POINT('Ctrl Pts',(0.777300516433143,0.0358890839459625,
-0.928004710552868));
#35135=CARTESIAN_POINT('Ctrl Pts',(0.668789051521523,0.397750328889649,
-0.917570747950388));
#35136=CARTESIAN_POINT('Ctrl Pts',(0.402637719871008,0.665858082479754,
-0.907136785347906));
#35137=CARTESIAN_POINT('Ctrl Pts',(0.0415808928872853,0.777016826591823,
-0.896702822745427));
#35138=CARTESIAN_POINT('Ctrl Pts',(-0.329276941530812,0.705025400441648,
-0.886268860142945));
#35139=CARTESIAN_POINT('Ctrl Pts',(-0.622521105437113,0.466852859850312,
-0.875834897540466));
#35140=CARTESIAN_POINT('Ctrl Pts',(-0.769031192860478,0.118638711592977,
-0.865400934937984));
#35141=CARTESIAN_POINT('Ctrl Pts',(-0.73427339889913,-0.257539696246457,
-0.854966972335505));
#35142=CARTESIAN_POINT('Ctrl Pts',(-0.526440462347927,-0.573013576696855,
-0.844533009733022));
#35143=CARTESIAN_POINT('Ctrl Pts',(-0.194520560057907,-0.753422770554806,
-0.834099047130545));
#35144=CARTESIAN_POINT('Ctrl Pts',(0.183249666810382,-0.75624313490388,
-0.823665084528061));
#35145=CARTESIAN_POINT('Ctrl Pts',(0.517826224589069,-0.580809883355642,
-0.813231121925582));
#35146=CARTESIAN_POINT('Ctrl Pts',(0.730346273449163,-0.268474282445113,
-0.802797159323101));
#35147=CARTESIAN_POINT('Ctrl Pts',(0.770716840097934,0.107143230607854,
-0.79236319672062));
#35148=CARTESIAN_POINT('Ctrl Pts',(0.629422202475751,0.457506077015547,
-0.781929234118141));
#35149=CARTESIAN_POINT('Ctrl Pts',(0.339766834898865,0.700030440322704,
-0.771495271515659));
#35150=CARTESIAN_POINT('Ctrl Pts',(-0.0299747696136733,0.777551048267703,
-0.76106130891318));
#35151=CARTESIAN_POINT('Ctrl Pts',(-0.392651039152918,0.671795564831834,
-0.750627346310697));
#35152=CARTESIAN_POINT('Ctrl Pts',(-0.662775767680288,0.407691551606601,
-0.740193383708218));
#35153=CARTESIAN_POINT('Ctrl Pts',(-0.776678017396761,0.0474908071970611,
-0.729759421105736));
#35154=CARTESIAN_POINT('Ctrl Pts',(-0.707509957315512,-0.32390396690222,
-0.719325458503256));
#35155=CARTESIAN_POINT('Ctrl Pts',(-0.471575149406303,-0.618951531170265,
-0.708891495900776));
#35156=CARTESIAN_POINT('Ctrl Pts',(-0.124485645778937,-0.768106401138927,
-0.698457533298295));
#35157=CARTESIAN_POINT('Ctrl Pts',(0.251946294775516,-0.736211371838605,
-0.688023570695814));
#35158=CARTESIAN_POINT('Ctrl Pts',(0.568992125251126,-0.530784401501965,
-0.677589608093334));
#35159=CARTESIAN_POINT('Ctrl Pts',(0.751921163041749,-0.200246558136555,
-0.667155645490853));
#35160=CARTESIAN_POINT('Ctrl Pts',(0.757615314330881,0.177491281382809,
-0.656721682888373));
#35161=CARTESIAN_POINT('Ctrl Pts',(0.584732414132281,0.513392757388168,
-0.646287720285892));
#35162=CARTESIAN_POINT('Ctrl Pts',(0.274022587194125,0.728282734371089,
-0.635853757683411));
#35163=CARTESIAN_POINT('Ctrl Pts',(-0.101276939472296,0.771509624701284,
-0.625419795080931));
#35164=CARTESIAN_POINT('Ctrl Pts',(-0.452704539459628,0.632884443977129,
-0.61498583247845));
#35165=CARTESIAN_POINT('Ctrl Pts',(-0.697425423884835,0.34508245042982,
-0.60455186987597));
#35166=CARTESIAN_POINT('Ctrl Pts',(-0.777756579810516,-0.0240587206027588,
-0.594117907273489));
#35167=CARTESIAN_POINT('Ctrl Pts',(-0.674763198638613,-0.387529025027261,
-0.583683944671008));
#35168=CARTESIAN_POINT('Ctrl Pts',(-0.412721788492088,-0.659655095318368,
-0.573249982068528));
#35169=CARTESIAN_POINT('Ctrl Pts',(-0.0533979730410232,-0.776294258609905,
-0.562816019466047));
#35170=CARTESIAN_POINT('Ctrl Pts',(0.318512246619028,-0.709953567657274,
-0.552382056863567));
#35171=CARTESIAN_POINT('Ctrl Pts',(0.615346135603009,-0.476270146948173,
-0.541948094261086));
#35172=CARTESIAN_POINT('Ctrl Pts',(0.767137155915032,-0.130325375465362,
-0.531514131658606));
#35173=CARTESIAN_POINT('Ctrl Pts',(0.738106737168653,0.246338312127524,
-0.521080169056125));
#35174=CARTESIAN_POINT('Ctrl Pts',(0.535097621960438,0.56493774386907,-0.510646206453644));
#35175=CARTESIAN_POINT('Ctrl Pts',(0.20596096711532,0.750376038730258,-0.500212243851164));
#35176=CARTESIAN_POINT('Ctrl Pts',(-0.171722623797873,0.758943647414989,
-0.489778281248683));
#35177=CARTESIAN_POINT('Ctrl Pts',(-0.50892957801762,0.588621104017174,
-0.479344318646202));
#35178=CARTESIAN_POINT('Ctrl Pts',(-0.726177046548315,0.279555033118634,
-0.468910356043722));
#35179=CARTESIAN_POINT('Ctrl Pts',(-0.772257758840454,-0.0954047870198923,
-0.458476393441241));
#35180=CARTESIAN_POINT('Ctrl Pts',(-0.636310057828871,-0.44787680201301,
-0.448042430838761));
#35181=CARTESIAN_POINT('Ctrl Pts',(-0.350378094607072,-0.694780044542982,
-0.43760846823628));
#35182=CARTESIAN_POINT('Ctrl Pts',(0.0181412792138254,-0.777917099351843,
-0.4271745056338));
#35183=CARTESIAN_POINT('Ctrl Pts',(0.382384582988461,-0.677691781098534,
-0.416740543031318));
#35184=CARTESIAN_POINT('Ctrl Pts',(0.656496245978095,-0.417728139454399,
-0.406306580428839));
#35185=CARTESIAN_POINT('Ctrl Pts',(0.775865572452267,-0.0593020485231105,
-0.395872617826357));
#35186=CARTESIAN_POINT('Ctrl Pts',(0.71235609003925,0.313102092711011,-0.385438655223877));
#35187=CARTESIAN_POINT('Ctrl Pts',(0.480937580760022,0.611705127399056,
-0.375004692621396));
#35188=CARTESIAN_POINT('Ctrl Pts',(0.136157562681014,0.766123513283346,
-0.364570730018916));
#35189=CARTESIAN_POINT('Ctrl Pts',(-0.240716072858233,0.739959385191357,
-0.354136767416435));
#35190=CARTESIAN_POINT('Ctrl Pts',(-0.560850667196364,0.539379874112098,
-0.343702804813955));
#35191=CARTESIAN_POINT('Ctrl Pts',(-0.748787487040106,0.211663456251418,
-0.333268842211474));
#35192=CARTESIAN_POINT('Ctrl Pts',(-0.760228057285642,-0.165944027859509,
-0.322834879608993));
#35193=CARTESIAN_POINT('Ctrl Pts',(-0.592475727944849,-0.504436944883207,
-0.312400917006513));
#35194=CARTESIAN_POINT('Ctrl Pts',(-0.285071300054314,-0.724029331642755,
-0.301966954404032));
#35195=CARTESIAN_POINT('Ctrl Pts',(0.0895271131383019,-0.772961199617318,
-0.291532991801552));
#35196=CARTESIAN_POINT('Ctrl Pts',(0.443023143994601,-0.639698844990308,
-0.281099029199071));
#35197=CARTESIAN_POINT('Ctrl Pts',(0.692094455558156,-0.355653462496774,
-0.27066506659659));
#35198=CARTESIAN_POINT('Ctrl Pts',(0.778032597283115,0.0122227909580681,
-0.26023110399411));
#35199=CARTESIAN_POINT('Ctrl Pts',(0.680581143349384,0.377218004776158,
-0.249797141391629));
#35200=CARTESIAN_POINT('Ctrl Pts',(0.422710313521399,0.653299414263413,
-0.239363178789149));
#35201=CARTESIAN_POINT('Ctrl Pts',(0.0652026943778876,0.775391960536891,
-0.228929216186668));
#35202=CARTESIAN_POINT('Ctrl Pts',(-0.307673823063876,0.714717431064052,
-0.218495253584187));
#35203=CARTESIAN_POINT('Ctrl Pts',(-0.608028707877235,0.485577090895019,
-0.208061290981707));
#35204=CARTESIAN_POINT('Ctrl Pts',(-0.765065550407644,0.1419820466464,-0.197627328379226));
#35205=CARTESIAN_POINT('Ctrl Pts',(-0.741769172281951,-0.235080250164509,
-0.187193365776746));
#35206=CARTESIAN_POINT('Ctrl Pts',(-0.543630981761309,-0.556730447339977,
-0.176759403174265));
#35207=CARTESIAN_POINT('Ctrl Pts',(-0.217353554555294,-0.747156946739445,
-0.166325440571784));
#35208=CARTESIAN_POINT('Ctrl Pts',(0.160155550638919,-0.761465819139253,
-0.155891477969304));
#35209=CARTESIAN_POINT('Ctrl Pts',(0.499915663487151,-0.59630128045638,
-0.145457515366823));
#35210=CARTESIAN_POINT('Ctrl Pts',(0.721838643854921,-0.290560778341041,
-0.135023552764343));
#35211=CARTESIAN_POINT('Ctrl Pts',(0.773621974230802,0.0836237451066752,
-0.124589590161862));
#35212=CARTESIAN_POINT('Ctrl Pts',(0.643046958594177,0.438187177596506,
-0.114155627559381));
#35213=CARTESIAN_POINT('Ctrl Pts',(0.454955040136648,0.605559893704277,
-0.107199652491061));
#35214=CARTESIAN_POINT('Ctrl Pts',(0.346702218893416,0.662233962746084,
-0.103721664956901));
#35215=CARTESIAN_POINT('',(0.351283760559811,0.670985139773177,-0.12));
#35216=CARTESIAN_POINT('Ctrl Pts',(0.708746600204741,0.237559480337495,
-0.12));
#35217=CARTESIAN_POINT('Ctrl Pts',(0.677871308579869,0.329674339059907,
-0.12));
#35218=CARTESIAN_POINT('Ctrl Pts',(0.630004482514663,0.414923577124779,
-0.12));
#35219=CARTESIAN_POINT('Ctrl Pts',(0.488745407170187,0.583538685988183,
-0.12));
#35220=CARTESIAN_POINT('Ctrl Pts',(0.404572366318542,0.639316291073142,
-0.12));
#35221=CARTESIAN_POINT('Ctrl Pts',(0.35128376055981,0.670985139773177,-0.12));
#35222=CARTESIAN_POINT('Ctrl Pts',(-0.459745842892902,-0.601806928197395,
-1.12625));
#35223=CARTESIAN_POINT('Ctrl Pts',(-0.416468302643127,-0.63488822608401,
-1.12472013661271));
#35224=CARTESIAN_POINT('Ctrl Pts',(-0.263250172568346,-0.728042154867832,
-1.11971228569126));
#35225=CARTESIAN_POINT('Ctrl Pts',(0.0423441932323986,-0.787268438306115,
-1.11122644723566));
#35226=CARTESIAN_POINT('Ctrl Pts',(0.408154628293017,-0.674543622261519,
-1.10079248463318));
#35227=CARTESIAN_POINT('Ctrl Pts',(0.677738701453828,-0.402813068451861,
-1.0903585220307));
#35228=CARTESIAN_POINT('Ctrl Pts',(0.787583785039379,-0.0361404951497401,
-1.07992455942821));
#35229=CARTESIAN_POINT('Ctrl Pts',(0.711782686348953,0.339053175380463,
-1.06949059682573));
#35230=CARTESIAN_POINT('Ctrl Pts',(0.468210400798597,0.634327583870302,
-1.05905663422325));
#35231=CARTESIAN_POINT('Ctrl Pts',(0.114275158775038,0.780085648735316,
-1.04862267162077));
#35232=CARTESIAN_POINT('Ctrl Pts',(-0.266595119432202,0.74196987248233,
-1.03818870901829));
#35233=CARTESIAN_POINT('Ctrl Pts',(-0.584626774041373,0.528964985372604,
-1.02775474641581));
#35234=CARTESIAN_POINT('Ctrl Pts',(-0.764856223313065,0.19127799592914,
-1.01732078381333));
#35235=CARTESIAN_POINT('Ctrl Pts',(-0.764801961726996,-0.191494973175329,
-1.00688682121085));
#35236=CARTESIAN_POINT('Ctrl Pts',(-0.584476642087926,-0.529130798350251,
-0.99645285860837));
#35237=CARTESIAN_POINT('Ctrl Pts',(-0.266384707070968,-0.742045509438616,
-0.98601889600589));
#35238=CARTESIAN_POINT('Ctrl Pts',(0.114496619465385,-0.780053123936526,
-0.975584933403408));
#35239=CARTESIAN_POINT('Ctrl Pts',(0.468390010412392,-0.634194881491942,
-0.965150970800929));
#35240=CARTESIAN_POINT('Ctrl Pts',(0.711879475926064,-0.338850945209237,
-0.954717008198448));
#35241=CARTESIAN_POINT('Ctrl Pts',(0.787572255433587,0.0363633449241354,
-0.944283045595968));
#35242=CARTESIAN_POINT('Ctrl Pts',(0.677626851623736,0.403006452460033,
-0.933849082993486));
#35243=CARTESIAN_POINT('Ctrl Pts',(0.407958428506616,0.674657150909495,
-0.923415120391007));
#35244=CARTESIAN_POINT('Ctrl Pts',(0.042130369016677,0.787284816735879,
-0.912981157788525));
#35245=CARTESIAN_POINT('Ctrl Pts',(-0.333628214598003,0.714342050500304,
-0.902547195186045));
#35246=CARTESIAN_POINT('Ctrl Pts',(-0.630747491734475,0.473022147824027,
-0.892113232583564));
#35247=CARTESIAN_POINT('Ctrl Pts',(-0.779193655806613,0.120206478312629,
-0.881679269981084));
#35248=CARTESIAN_POINT('Ctrl Pts',(-0.743976550446063,-0.260942988134434,
-0.871245307378604));
#35249=CARTESIAN_POINT('Ctrl Pts',(-0.533397178462468,-0.58058573930206,
-0.860811344776122));
#35250=CARTESIAN_POINT('Ctrl Pts',(-0.197091077355777,-0.763378973969726,
-0.850377382173643));
#35251=CARTESIAN_POINT('Ctrl Pts',(0.185671243420201,-0.766236608391142,
-0.83994341957116));
#35252=CARTESIAN_POINT('Ctrl Pts',(0.524669106735824,-0.588485071271487,
-0.829509456968682));
#35253=CARTESIAN_POINT('Ctrl Pts',(0.739997529484913,-0.272022070847804,
-0.819075494366199));
#35254=CARTESIAN_POINT('Ctrl Pts',(0.780901578249222,0.108559088795519,
-0.80864153176372));
#35255=CARTESIAN_POINT('Ctrl Pts',(0.637739784219531,0.46355185070908,-0.798207569161239));
#35256=CARTESIAN_POINT('Ctrl Pts',(0.344256728029392,0.709281083829744,
-0.787773606558758));
#35257=CARTESIAN_POINT('Ctrl Pts',(-0.0303708751141343,0.787826097953732,
-0.777339643956278));
#35258=CARTESIAN_POINT('Ctrl Pts',(-0.397839777494349,0.680673094896106,
-0.766905681353797));
#35259=CARTESIAN_POINT('Ctrl Pts',(-0.671534104459313,0.413079044760479,
-0.756471718751317));
#35260=CARTESIAN_POINT('Ctrl Pts',(-0.786941530302541,0.0481183806594935,
-0.746037756148835));
#35261=CARTESIAN_POINT('Ctrl Pts',(-0.716859439874856,-0.32818423809578,
-0.735603793546356));
#35262=CARTESIAN_POINT('Ctrl Pts',(-0.477806840690935,-0.627130746863161,
-0.725169830943874));
#35263=CARTESIAN_POINT('Ctrl Pts',(-0.126130677572575,-0.778256643304304,
-0.714735868341395));
#35264=CARTESIAN_POINT('Ctrl Pts',(0.25527567193062,-0.745940132981574,
-0.704301905738912));
#35265=CARTESIAN_POINT('Ctrl Pts',(0.576511145861978,-0.537798521166717,
-0.693867943136434));
#35266=CARTESIAN_POINT('Ctrl Pts',(0.761857523268443,-0.202892742382455,
-0.683433980533952));
#35267=CARTESIAN_POINT('Ctrl Pts',(0.767626920662054,0.179836763057753,
-0.673000017931472));
#35268=CARTESIAN_POINT('Ctrl Pts',(0.5924594368424,0.520177052904666,-0.662566055328991));
#35269=CARTESIAN_POINT('Ctrl Pts',(0.277643694393179,0.737906721500696,
-0.652132092726511));
#35270=CARTESIAN_POINT('Ctrl Pts',(-0.102615276791043,0.781704839208058,
-0.64169813012403));
#35271=CARTESIAN_POINT('Ctrl Pts',(-0.458686862609216,0.641247777962555,
-0.631264167521549));
#35272=CARTESIAN_POINT('Ctrl Pts',(-0.706641643062577,0.349642587454705,
-0.620830204919069));
#35273=CARTESIAN_POINT('Ctrl Pts',(-0.78803434551991,-0.0243766477023704,
-0.610396242316588));
#35274=CARTESIAN_POINT('Ctrl Pts',(-0.683679944886674,-0.392650077845343,
-0.599962279714107));
#35275=CARTESIAN_POINT('Ctrl Pts',(-0.418175754367012,-0.668372193565666,
-0.589528317111627));
#35276=CARTESIAN_POINT('Ctrl Pts',(-0.0541036075165375,-0.786552700285172,
-0.579094354509147));
#35277=CARTESIAN_POINT('Ctrl Pts',(0.322721268222062,-0.719335341624019,
-0.568660391906665));
#35278=CARTESIAN_POINT('Ctrl Pts',(0.623477707326195,-0.482563880889846,
-0.558226429304185));
#35279=CARTESIAN_POINT('Ctrl Pts',(0.777274589863052,-0.132047577128186,
-0.547792466701704));
#35280=CARTESIAN_POINT('Ctrl Pts',(0.747860544863849,0.24959358186489,-0.537358504099224));
#35281=CARTESIAN_POINT('Ctrl Pts',(0.542168739239194,0.572403187328635,
-0.526924541496743));
#35282=CARTESIAN_POINT('Ctrl Pts',(0.208682665163581,0.760291980710322,
-0.516490578894263));
#35283=CARTESIAN_POINT('Ctrl Pts',(-0.17399187479518,0.768972807176858,
-0.506056616291782));
#35284=CARTESIAN_POINT('Ctrl Pts',(-0.515654894268523,0.596399514326692,
-0.495622653689302));
#35285=CARTESIAN_POINT('Ctrl Pts',(-0.735773207791699,0.283249249545548,
-0.485188691086821));
#35286=CARTESIAN_POINT('Ctrl Pts',(-0.782462859663334,-0.0966655260145846,
-0.47475472848434));
#35287=CARTESIAN_POINT('Ctrl Pts',(-0.64471866003509,-0.453795328396784,
-0.46432076588186));
#35288=CARTESIAN_POINT('Ctrl Pts',(-0.355008211612258,-0.703961306010569,
-0.453886803279379));
#35289=CARTESIAN_POINT('Ctrl Pts',(0.0183810095128271,-0.788196986267641,
-0.443452840676899));
#35290=CARTESIAN_POINT('Ctrl Pts',(0.38743765390661,-0.686647227481269,
-0.433018878074418));
#35291=CARTESIAN_POINT('Ctrl Pts',(0.665171601199011,-0.423248262406725,
-0.422584915471937));
#35292=CARTESIAN_POINT('Ctrl Pts',(0.786118349198421,-0.0600857031737155,
-0.412150952869457));
#35293=CARTESIAN_POINT('Ctrl Pts',(0.721769612451196,0.317239621129978,
-0.401716990266976));
#35294=CARTESIAN_POINT('Ctrl Pts',(0.48729299311423,0.619788584544703,-0.391283027664495));
#35295=CARTESIAN_POINT('Ctrl Pts',(0.137956834542062,0.776247552318673,
-0.380849065062015));
#35296=CARTESIAN_POINT('Ctrl Pts',(-0.24389704678188,0.749737674945354,
-0.370415102459534));
#35297=CARTESIAN_POINT('Ctrl Pts',(-0.568262101448461,0.54650757977013,
-0.359981139857054));
#35298=CARTESIAN_POINT('Ctrl Pts',(-0.758682436896782,0.214460510585722,
-0.349547177254573));
#35299=CARTESIAN_POINT('Ctrl Pts',(-0.770274190049179,-0.168136916847512,
-0.339113214652093));
#35300=CARTESIAN_POINT('Ctrl Pts',(-0.600305075684733,-0.511102892647913,
-0.328679252049612));
#35301=CARTESIAN_POINT('Ctrl Pts',(-0.288838411909729,-0.73359711162755,
-0.318245289447131));
#35302=CARTESIAN_POINT('Ctrl Pts',(0.0907101808452941,-0.783175596150043,
-0.307811326844651));
#35303=CARTESIAN_POINT('Ctrl Pts',(0.448877531081785,-0.648152228766222,
-0.29737736424217));
#35304=CARTESIAN_POINT('Ctrl Pts',(0.70124022796002,-0.360353291538616,
-0.286943401639689));
#35305=CARTESIAN_POINT('Ctrl Pts',(0.78831401046138,0.0123843106225018,
-0.276509439037209));
#35306=CARTESIAN_POINT('Ctrl Pts',(0.689574771586232,0.382202801273025,
-0.266075476434728));
#35307=CARTESIAN_POINT('Ctrl Pts',(0.42829627406239,0.661932524534907,-0.255641513832248));
#35308=CARTESIAN_POINT('Ctrl Pts',(0.0660643238823282,0.785638478676651,
-0.245207551229767));
#35309=CARTESIAN_POINT('Ctrl Pts',(-0.311739618905983,0.724162157724785,
-0.234773588627286));
#35310=CARTESIAN_POINT('Ctrl Pts',(-0.616063582497866,0.491993812660696,
-0.224339626024806));
#35311=CARTESIAN_POINT('Ctrl Pts',(-0.775175608854641,0.143858286910066,
-0.213905663422325));
#35312=CARTESIAN_POINT('Ctrl Pts',(-0.751571377703373,-0.238186748774504,
-0.203471700819845));
#35313=CARTESIAN_POINT('Ctrl Pts',(-0.550814864235531,-0.564087434409687,
-0.193037738217364));
#35314=CARTESIAN_POINT('Ctrl Pts',(-0.220225801435375,-0.757030349608765,
-0.182603775614884));
#35315=CARTESIAN_POINT('Ctrl Pts',(0.162271947040125,-0.771528308468155,
-0.172169813012403));
#35316=CARTESIAN_POINT('Ctrl Pts',(0.50652186418947,-0.604181181458613,
-0.161735850409922));
#35317=CARTESIAN_POINT('Ctrl Pts',(0.731377474710374,-0.294400431622865,
-0.151301887807442));
#35318=CARTESIAN_POINT('Ctrl Pts',(0.783845102655791,0.0847288019872719,
-0.140867925204961));
#35319=CARTESIAN_POINT('Ctrl Pts',(0.651544586453759,0.443977659175325,
-0.130433962602481));
#35320=CARTESIAN_POINT('Ctrl Pts',(0.460967102820801,0.613562143858194,
-0.12347798753416));
#35321=CARTESIAN_POINT('Ctrl Pts',(0.35128376055981,0.670985139773177,-0.12));
#35322=CARTESIAN_POINT('Ctrl Pts',(-0.495956409719265,-0.649207665313755,
-1.15727273924394));
#35323=CARTESIAN_POINT('Ctrl Pts',(-0.388302693694881,-0.731448762184642,
-1.15374460067508));
#35324=CARTESIAN_POINT('Ctrl Pts',(-0.13140455693268,-0.841265750467438,
-1.14668832353737));
#35325=CARTESIAN_POINT('Ctrl Pts',(0.286034174319602,-0.801958781222045,
-1.1361039078308));
#35326=CARTESIAN_POINT('Ctrl Pts',(0.634034477218437,-0.568280999134343,
-1.12551949212423));
#35327=CARTESIAN_POINT('Ctrl Pts',(0.828384689818385,-0.196826841568886,
-1.11493507641766));
#35328=CARTESIAN_POINT('Ctrl Pts',(0.821897829369206,0.222332451391628,
-1.10435066071109));
#35329=CARTESIAN_POINT('Ctrl Pts',(0.616183750099589,0.587599496275833,
-1.09376624500451));
#35330=CARTESIAN_POINT('Ctrl Pts',(0.261091496307317,0.810421806269904,
-1.08318182929794));
#35331=CARTESIAN_POINT('Ctrl Pts',(-0.157289815040412,0.836787381022574,
-1.07259741359137));
#35332=CARTESIAN_POINT('Ctrl Pts',(-0.537543482173721,0.660303137862947,
-1.0620129978848));
#35333=CARTESIAN_POINT('Ctrl Pts',(-0.7874880639875,0.323752245535046,-1.05142858217823));
#35334=CARTESIAN_POINT('Ctrl Pts',(-0.846534688677586,-0.0912809764781306,
-1.04084416647166));
#35335=CARTESIAN_POINT('Ctrl Pts',(-0.700368959446377,-0.484186307032688,
-1.03025975076509));
#35336=CARTESIAN_POINT('Ctrl Pts',(-0.38442387329105,-0.759717979177561,
-1.01967533505852));
#35337=CARTESIAN_POINT('Ctrl Pts',(0.0247111232736773,-0.851083110906004,
-1.00909091935195));
#35338=CARTESIAN_POINT('Ctrl Pts',(0.42785576069194,-0.736133514901142,
-0.998506503645377));
#35339=CARTESIAN_POINT('Ctrl Pts',(0.727282047487868,-0.442734604895683,
-0.987922087938807));
#35340=CARTESIAN_POINT('Ctrl Pts',(0.850404740342968,-0.0420104871635215,
-0.977337672232236));
#35341=CARTESIAN_POINT('Ctrl Pts',(0.767377146099821,0.368897575755567,
-0.966753256525664));
#35342=CARTESIAN_POINT('Ctrl Pts',(0.498326337204486,0.690379581274127,
-0.956168840819095));
#35343=CARTESIAN_POINT('Ctrl Pts',(0.108474086749781,0.844503687104731,
-0.945584425112522));
#35344=CARTESIAN_POINT('Ctrl Pts',(-0.307673836701548,0.793908001690772,
-0.935000009405953));
#35345=CARTESIAN_POINT('Ctrl Pts',(-0.649237214524841,0.550857644208324,
-0.924415593699381));
#35346=CARTESIAN_POINT('Ctrl Pts',(-0.833416191506255,0.174271502818131,
-0.913831177992811));
#35347=CARTESIAN_POINT('Ctrl Pts',(-0.815563145108209,-0.244560547230945,
-0.90324676228624));
#35348=CARTESIAN_POINT('Ctrl Pts',(-0.600005909618337,-0.604107617370174,
-0.892662346579669));
#35349=CARTESIAN_POINT('Ctrl Pts',(-0.238998646675454,-0.817210347352623,
-0.882077930873097));
#35350=CARTESIAN_POINT('Ctrl Pts',(0.17994531181254,-0.832209582792671,
-0.871493515166529));
#35351=CARTESIAN_POINT('Ctrl Pts',(0.555267949047113,-0.64546929415458,
-0.860909099459956));
#35352=CARTESIAN_POINT('Ctrl Pts',(0.795985681346874,-0.302258002417496,
-0.850324683753387));
#35353=CARTESIAN_POINT('Ctrl Pts',(0.843745082180559,0.114224958881187,
-0.839740268046815));
#35354=CARTESIAN_POINT('Ctrl Pts',(0.686968588642089,0.503018153901045,
-0.829155852340245));
#35355=CARTESIAN_POINT('Ctrl Pts',(0.363661068552687,0.769872542797965,
-0.818571436633673));
#35356=CARTESIAN_POINT('Ctrl Pts',(-0.047803103913807,0.850098799076459,
-0.807987020927103));
#35357=CARTESIAN_POINT('Ctrl Pts',(-0.447679119223231,0.724248928992339,
-0.797402605220532));
#35358=CARTESIAN_POINT('Ctrl Pts',(-0.739031303134287,0.422830743823914,
-0.786818189513961));
#35359=CARTESIAN_POINT('Ctrl Pts',(-0.85123171271497,0.0189123294010521,
-0.776233773807391));
#35360=CARTESIAN_POINT('Ctrl Pts',(-0.757081361438328,-0.389590704583327,
-0.765649358100819));
#35361=CARTESIAN_POINT('Ctrl Pts',(-0.479403643135562,-0.703651370980965,
-0.755064942394249));
#35362=CARTESIAN_POINT('Ctrl Pts',(-0.0855116143916565,-0.847136865411472,
-0.744480526687678));
#35363=CARTESIAN_POINT('Ctrl Pts',(0.329109654614668,-0.785264248628737,
-0.733896110981106));
#35364=CARTESIAN_POINT('Ctrl Pts',(0.663950028923553,-0.533032329251663,
-0.723311695274536));
#35365=CARTESIAN_POINT('Ctrl Pts',(0.837839405292465,-0.151585737700515,
-0.712727279567964));
#35366=CARTESIAN_POINT('Ctrl Pts',(0.808624507964925,0.266607408099481,
-0.702142863861395));
#35367=CARTESIAN_POINT('Ctrl Pts',(0.583387446549703,0.620171099087388,
-0.691558448154823));
#35368=CARTESIAN_POINT('Ctrl Pts',(0.216728911202081,0.82339643185054,-0.680974032448252));
#35369=CARTESIAN_POINT('Ctrl Pts',(-0.202467816811898,0.82701867457178,
-0.670389616741683));
#35370=CARTESIAN_POINT('Ctrl Pts',(-0.572583445726543,0.6301597437277,-0.659805201035111));
#35371=CARTESIAN_POINT('Ctrl Pts',(-0.803896645273107,0.280541064113054,
-0.64922078532854));
#35372=CARTESIAN_POINT('Ctrl Pts',(-0.840333782374013,-0.137084788127738,
-0.63863636962197));
#35373=CARTESIAN_POINT('Ctrl Pts',(-0.67306197304253,-0.521479324018831,
-0.628051953915399));
#35374=CARTESIAN_POINT('Ctrl Pts',(-0.342630299990165,-0.779459801698388,
-0.617467538208828));
#35375=CARTESIAN_POINT('Ctrl Pts',(0.0708598658787424,-0.848488057866867,
-0.606883122502257));
#35376=CARTESIAN_POINT('Ctrl Pts',(0.467172585207631,-0.7118306544154,-0.596298706795686));
#35377=CARTESIAN_POINT('Ctrl Pts',(0.750235977744155,-0.402615303525977,
-0.585714291089116));
#35378=CARTESIAN_POINT('Ctrl Pts',(0.851431422320551,0.00419976430822168,
-0.575129875382545));
#35379=CARTESIAN_POINT('Ctrl Pts',(0.746227693570422,0.409996749113464,
-0.564545459675974));
#35380=CARTESIAN_POINT('Ctrl Pts',(0.460127682361612,0.716404648826047,
-0.553961043969404));
#35381=CARTESIAN_POINT('Ctrl Pts',(0.0624861297268952,0.849145799334128,
-0.543376628262831));
#35382=CARTESIAN_POINT('Ctrl Pts',(-0.350302955852819,0.776041844268606,
-0.532792212556262));
#35383=CARTESIAN_POINT('Ctrl Pts',(-0.67817358692588,0.514814229534427,
-0.522207796849691));
#35384=CARTESIAN_POINT('Ctrl Pts',(-0.841645225850065,0.12878827096765,
-0.511623381143119));
#35385=CARTESIAN_POINT('Ctrl Pts',(-0.80109000565714,-0.288457809343551,
-0.501038965436549));
#35386=CARTESIAN_POINT('Ctrl Pts',(-0.566339092665934,-0.635777584579208,
-0.490454549729978));
#35387=CARTESIAN_POINT('Ctrl Pts',(-0.194299470937418,-0.82897576594764,
-0.479870134023407));
#35388=CARTESIAN_POINT('Ctrl Pts',(0.224841125840774,-0.821218346766367,
-0.469285718316837));
#35389=CARTESIAN_POINT('Ctrl Pts',(0.589477012918694,-0.614385836568145,
-0.458701302610266));
#35390=CARTESIAN_POINT('Ctrl Pts',(0.811215227944597,-0.258617398652365,
-0.448116886903695));
#35391=CARTESIAN_POINT('Ctrl Pts',(0.8363032512486,0.159843601330507,-0.437532471197124));
#35392=CARTESIAN_POINT('Ctrl Pts',(0.658659386600812,0.539556222628657,
-0.426948055490553));
#35393=CARTESIAN_POINT('Ctrl Pts',(0.321347051500517,0.788472686544893,
-0.416363639783983));
#35394=CARTESIAN_POINT('Ctrl Pts',(-0.0938644121072648,0.846252076555809,
-0.405779224077412));
#35395=CARTESIAN_POINT('Ctrl Pts',(-0.48632179762979,0.698887840846459,
-0.395194808370841));
#35396=CARTESIAN_POINT('Ctrl Pts',(-0.760887812970069,0.382103181111099,
-0.38461039266427));
#35397=CARTESIAN_POINT('Ctrl Pts',(-0.851003722888249,-0.0273087632644408,
-0.374025976957699));
#35398=CARTESIAN_POINT('Ctrl Pts',(-0.734824139984663,-0.43010067223277,
-0.363441561251128));
#35399=CARTESIAN_POINT('Ctrl Pts',(-0.440512659294738,-0.728630017160833,
-0.352857145544558));
#35400=CARTESIAN_POINT('Ctrl Pts',(-0.0394145998886176,-0.850529008473494,
-0.342272729837987));
#35401=CARTESIAN_POINT('Ctrl Pts',(0.371238123405903,-0.766247584505002,
-0.331688314131416));
#35402=CARTESIAN_POINT('Ctrl Pts',(0.691897407156195,-0.496216769731146,
-0.321103898424845));
#35403=CARTESIAN_POINT('Ctrl Pts',(0.844830849187047,-0.105895901792902,
-0.310519482718274));
#35404=CARTESIAN_POINT('Ctrl Pts',(0.792965189320117,0.310095649688961,
-0.299935067011704));
#35405=CARTESIAN_POINT('Ctrl Pts',(0.548873412549209,0.650915573609104,
-0.289350651305133));
#35406=CARTESIAN_POINT('Ctrl Pts',(0.171726850179941,0.833944238330876,
-0.278766235598562));
#35407=CARTESIAN_POINT('Ctrl Pts',(-0.247048745074761,0.814812873511381,
-0.268181819891991));
#35408=CARTESIAN_POINT('Ctrl Pts',(-0.605936216145871,0.598159196372131,
-0.257597404185421));
#35409=CARTESIAN_POINT('Ctrl Pts',(-0.817936008537478,0.236503161103038,
-0.247012988478849));
#35410=CARTESIAN_POINT('Ctrl Pts',(-0.831656513568513,-0.182484627408237,
-0.236428572772279));
#35411=CARTESIAN_POINT('Ctrl Pts',(-0.643771334910445,-0.557235529878874,
-0.225844157065708));
#35412=CARTESIAN_POINT('Ctrl Pts',(-0.29982721760122,-0.796904554312883,
-0.215259741359137));
#35413=CARTESIAN_POINT('Ctrl Pts',(0.116800205661488,-0.843392505842622,
-0.204675325652567));
#35414=CARTESIAN_POINT('Ctrl Pts',(0.50511183077167,-0.685430019722115,
-0.194090909945995));
#35415=CARTESIAN_POINT('Ctrl Pts',(0.770980560490097,-0.361309503413322,
-0.183506494239425));
#35416=CARTESIAN_POINT('Ctrl Pts',(0.849945784476039,0.0503976618012751,
-0.172922078532854));
#35417=CARTESIAN_POINT('Ctrl Pts',(0.722885284777081,0.449887613677287,
-0.162337662826283));
#35418=CARTESIAN_POINT('Ctrl Pts',(0.42056085792794,0.740318564577236,-0.151753247119712));
#35419=CARTESIAN_POINT('Ctrl Pts',(0.0163382438424028,0.85128520335196,
-0.141168831413141));
#35420=CARTESIAN_POINT('Ctrl Pts',(-0.391950752487246,0.755890089971351,
-0.130584415706571));
#35421=CARTESIAN_POINT('Ctrl Pts',(-0.600629835243707,0.5701228592569,-0.123528138568857));
#35422=CARTESIAN_POINT('Ctrl Pts',(-0.676565692095422,0.457932546695692,
-0.12));
#35423=CARTESIAN_POINT('Ctrl Pts',(-0.483897209295839,-0.633422154331299,
-1.14693182616263));
#35424=CARTESIAN_POINT('Ctrl Pts',(-0.378861097787544,-0.71366355556206,
-1.14340368759377));
#35425=CARTESIAN_POINT('Ctrl Pts',(-0.128209449746748,-0.820810339275165,
-1.13634741045605));
#35426=CARTESIAN_POINT('Ctrl Pts',(0.279079241651182,-0.782459120597521,
-1.12576299474949));
#35427=CARTESIAN_POINT('Ctrl Pts',(0.618617902926218,-0.554463223355893,
-1.11517857904291));
#35428=CARTESIAN_POINT('Ctrl Pts',(0.808242482143577,-0.192040988851441,
-1.10459416333634));
#35429=CARTESIAN_POINT('Ctrl Pts',(0.80191334997201,0.216926428726288,-1.09400974762977));
#35430=CARTESIAN_POINT('Ctrl Pts',(0.601201216968671,0.57331199044784,-1.0834253319232));
#35431=CARTESIAN_POINT('Ctrl Pts',(0.254743045876755,0.790716366844582,
-1.07284091621663));
#35432=CARTESIAN_POINT('Ctrl Pts',(-0.15346530674298,0.816440861566847,
-1.06225650051006));
#35433=CARTESIAN_POINT('Ctrl Pts',(-0.524473090379596,0.644247840010836,
-1.05167208480349));
#35434=CARTESIAN_POINT('Ctrl Pts',(-0.768340259445449,0.315880196419577,
-1.04108766909692));
#35435=CARTESIAN_POINT('Ctrl Pts',(-0.825951163036847,-0.0890614757949581,
-1.03050325339035));
#35436=CARTESIAN_POINT('Ctrl Pts',(-0.683339459500824,-0.47241329713835,
-1.01991883768378));
#35437=CARTESIAN_POINT('Ctrl Pts',(-0.375076591060762,-0.741245405385504,
-1.0093344219772));
#35438=CARTESIAN_POINT('Ctrl Pts',(0.0241102712987759,-0.830388990192415,
-0.998750006270636));
#35439=CARTESIAN_POINT('Ctrl Pts',(0.417452430339941,-0.718234398324306,
-0.988165590564063));
#35440=CARTESIAN_POINT('Ctrl Pts',(0.709598154703862,-0.431969494837229,
-0.977581174857493));
#35441=CARTESIAN_POINT('Ctrl Pts',(0.829727114237416,-0.0409890004468207,
-0.966996759150922));
#35442=CARTESIAN_POINT('Ctrl Pts',(0.748718339350226,0.359927816086022,
-0.956412343444352));
#35443=CARTESIAN_POINT('Ctrl Pts',(0.486209511897153,0.673592973468133,
-0.945827927737781));
#35444=CARTESIAN_POINT('Ctrl Pts',(0.105836534885889,0.823969545350454,
-0.93524351203121));
#35445=CARTESIAN_POINT('Ctrl Pts',(-0.300192734755657,0.774604096100419,
-0.924659096324639));
#35446=CARTESIAN_POINT('Ctrl Pts',(-0.633450985052106,0.537463518018798,
-0.914074680618068));
#35447=CARTESIAN_POINT('Ctrl Pts',(-0.813151642661748,0.170034084086582,
-0.903490264911497));
#35448=CARTESIAN_POINT('Ctrl Pts',(-0.795732693818374,-0.238614047504507,
-0.892905849204926));
#35449=CARTESIAN_POINT('Ctrl Pts',(-0.585416741341586,-0.589418715901377,
-0.882321433498356));
#35450=CARTESIAN_POINT('Ctrl Pts',(-0.233187384788913,-0.797339844272723,
-0.871737017791784));
#35451=CARTESIAN_POINT('Ctrl Pts',(0.175569934182818,-0.811974372688474,
-0.861152602085215));
#35452=CARTESIAN_POINT('Ctrl Pts',(0.541766586114726,-0.629774681820032,
-0.850568186378643));
#35453=CARTESIAN_POINT('Ctrl Pts',(0.776631256890554,-0.294908586704127,
-0.839983770672073));
#35454=CARTESIAN_POINT('Ctrl Pts',(0.823229385936095,0.111447574325788,
-0.829399354965501));
#35455=CARTESIAN_POINT('Ctrl Pts',(0.670264919261704,0.490787246878494,
-0.818814939258932));
#35456=CARTESIAN_POINT('Ctrl Pts',(0.354818634770338,0.75115306037541,-0.808230523552359));
#35457=CARTESIAN_POINT('Ctrl Pts',(-0.0466407694834795,0.829428611945336,
-0.79764610784579));
#35458=CARTESIAN_POINT('Ctrl Pts',(-0.436793783096309,0.70663878660883,
-0.787061692139218));
#35459=CARTESIAN_POINT('Ctrl Pts',(-0.721061726717829,0.412549596962952,
-0.776477276432648));
#35460=CARTESIAN_POINT('Ctrl Pts',(-0.830533978742309,0.0184524753367595,
-0.765892860726077));
#35461=CARTESIAN_POINT('Ctrl Pts',(-0.738672897114632,-0.380117790638464,
-0.755308445019506));
#35462=CARTESIAN_POINT('Ctrl Pts',(-0.467746923909844,-0.686542059064458,
-0.744724029312935));
#35463=CARTESIAN_POINT('Ctrl Pts',(-0.0834323959840071,-0.826538697818774,
-0.734139613606364));
#35464=CARTESIAN_POINT('Ctrl Pts',(0.321107339877917,-0.766170516248254,
-0.723555197899794));
#35465=CARTESIAN_POINT('Ctrl Pts',(0.647806056765878,-0.520071626325674,
-0.712970782193223));
#35466=CARTESIAN_POINT('Ctrl Pts',(0.817467305823512,-0.147899924277319,
-0.702386366486651));
#35467=CARTESIAN_POINT('Ctrl Pts',(0.788962769921528,0.260124838047687,
-0.691801950780082));
#35468=CARTESIAN_POINT('Ctrl Pts',(0.569202356883383,0.605091613402457,
-0.68121753507351));
#35469=CARTESIAN_POINT('Ctrl Pts',(0.211459138846046,0.803375513872608,
-0.67063311936694));
#35470=CARTESIAN_POINT('Ctrl Pts',(-0.197544803550289,0.806909681613664,
-0.660048703660368));
#35471=CARTESIAN_POINT('Ctrl Pts',(-0.558661055782917,0.61483738373907,
-0.649464287953798));
#35472=CARTESIAN_POINT('Ctrl Pts',(-0.784349865404781,0.273719696644377,
-0.638879872247227));
#35473=CARTESIAN_POINT('Ctrl Pts',(-0.819901032024117,-0.133751565887559,
-0.628295456540657));
#35474=CARTESIAN_POINT('Ctrl Pts',(-0.656696443590252,-0.508799532888447,
-0.617711040834085));
#35475=CARTESIAN_POINT('Ctrl Pts',(-0.334299230207119,-0.760507204682845,
-0.607126625127515));
#35476=CARTESIAN_POINT('Ctrl Pts',(0.0691369053365199,-0.827857035974254,
-0.596542209420944));
#35477=CARTESIAN_POINT('Ctrl Pts',(0.455813264656582,-0.69452246288705,
-0.585957793714373));
#35478=CARTESIAN_POINT('Ctrl Pts',(0.731993959205463,-0.392825695924158,
-0.575373378007802));
#35479=CARTESIAN_POINT('Ctrl Pts',(0.830728832400646,0.0040976468669884,
-0.564788962301232));
#35480=CARTESIAN_POINT('Ctrl Pts',(0.728083136625648,0.400027661359743,
-0.55420454659466));
#35481=CARTESIAN_POINT('Ctrl Pts',(0.448939658911917,0.69898524043619,-0.543620130888091));
#35482=CARTESIAN_POINT('Ctrl Pts',(0.060966776922306,0.828498784430789,
-0.533035715181518));
#35483=CARTESIAN_POINT('Ctrl Pts',(-0.341785325128097,0.757172355028014,
-0.522451299474948));
#35484=CARTESIAN_POINT('Ctrl Pts',(-0.661683768372588,0.502296500449523,
-0.511866883768377));
#35485=CARTESIAN_POINT('Ctrl Pts',(-0.821180587698315,0.125656778882156,
-0.501282468061807));
#35486=CARTESIAN_POINT('Ctrl Pts',(-0.781611469346073,-0.281443945890219,
-0.490698052355235));
#35487=CARTESIAN_POINT('Ctrl Pts',(-0.552568534422829,-0.620318626560091,
-0.480113636648665));
#35488=CARTESIAN_POINT('Ctrl Pts',(-0.189575071340432,-0.808819186232531,
-0.469529220942094));
#35489=CARTESIAN_POINT('Ctrl Pts',(0.219374104653414,-0.8012503890165,-0.458944805235523));
#35490=CARTESIAN_POINT('Ctrl Pts',(0.575143855196601,-0.599447019778413,
-0.448360389528952));
#35491=CARTESIAN_POINT('Ctrl Pts',(0.791490496438744,-0.252329106007655,
-0.437775973822382));
#35492=CARTESIAN_POINT('Ctrl Pts',(0.815968503428166,0.155956997614794,
-0.42719155811581));
#35493=CARTESIAN_POINT('Ctrl Pts',(0.64264405662799,0.526436890967901,-0.416607142409241));
#35494=CARTESIAN_POINT('Ctrl Pts',(0.313533484776547,0.769300940865017,
-0.406022726702668));
#35495=CARTESIAN_POINT('Ctrl Pts',(-0.0915820950809177,0.825675422640392,
-0.395438310996099));
#35496=CARTESIAN_POINT('Ctrl Pts',(-0.474496863194084,0.681894354360349,
-0.384853895289527));
#35497=CARTESIAN_POINT('Ctrl Pts',(-0.742386794621416,0.372812326606253,
-0.374269479582957));
#35498=CARTESIAN_POINT('Ctrl Pts',(-0.830311532497566,-0.0266447495667293,
-0.363685063876386));
#35499=CARTESIAN_POINT('Ctrl Pts',(-0.716956860912571,-0.419642756764674,
-0.353100648169815));
#35500=CARTESIAN_POINT('Ctrl Pts',(-0.429801575934612,-0.710913348438998,
-0.342516232463245));
#35501=CARTESIAN_POINT('Ctrl Pts',(-0.0384562322773691,-0.829848360783256,
-0.331931816756673));
#35502=CARTESIAN_POINT('Ctrl Pts',(0.36221145322434,-0.747616243091868,
-0.321347401050103));
#35503=CARTESIAN_POINT('Ctrl Pts',(0.675073893351689,-0.484151238643362,
-0.310762985343532));
#35504=CARTESIAN_POINT('Ctrl Pts',(0.824288752473332,-0.103321038601875,
-0.300178569636961));
#35505=CARTESIAN_POINT('Ctrl Pts',(0.773684208251188,0.30255566126105,-0.28959415393039));
#35506=CARTESIAN_POINT('Ctrl Pts',(0.535527533033774,0.635088534766467,
-0.27900973822382));
#35507=CARTESIAN_POINT('Ctrl Pts',(0.167551304781554,0.813666850006192,
-0.268425322517249));
#35508=CARTESIAN_POINT('Ctrl Pts',(-0.2410417447158,0.795000665106163,-0.257840906810678));
#35509=CARTESIAN_POINT('Ctrl Pts',(-0.591202852222919,0.583614931003628,
-0.247256491104107));
#35510=CARTESIAN_POINT('Ctrl Pts',(-0.798047860976135,0.230752577050439,
-0.236672075397536));
#35511=CARTESIAN_POINT('Ctrl Pts',(-0.811434751365163,-0.17804750621576,
-0.226087659690966));
#35512=CARTESIAN_POINT('Ctrl Pts',(-0.62811800852449,-0.543686325137944,
-0.215503243984394));
#35513=CARTESIAN_POINT('Ctrl Pts',(-0.292536906520256,-0.777527787422745,
-0.204918828277824));
#35514=CARTESIAN_POINT('Ctrl Pts',(0.113960203875109,-0.822885382506262,
-0.194334412571253));
#35515=CARTESIAN_POINT('Ctrl Pts',(0.492830015910225,-0.668763760708061,
-0.183749996864682));
#35516=CARTESIAN_POINT('Ctrl Pts',(0.752234136571959,-0.352524248033688,
-0.173165581158111));
#35517=CARTESIAN_POINT('Ctrl Pts',(0.829279317901195,0.0491722405896055,
-0.162581165451541));
#35518=CARTESIAN_POINT('Ctrl Pts',(0.705308299458539,0.438948577917225,
-0.15199674974497));
#35519=CARTESIAN_POINT('Ctrl Pts',(0.410334903435544,0.72231768834605,-0.141412334038399));
#35520=CARTESIAN_POINT('Ctrl Pts',(0.0159409787739384,0.830586168752268,
-0.130827918331828));
#35521=CARTESIAN_POINT('Ctrl Pts',(-0.3824204538809,0.737510591462186,-0.120243502625258));
#35522=CARTESIAN_POINT('Ctrl Pts',(-0.586025496189812,0.556260298574102,
-0.113187225487544));
#35523=CARTESIAN_POINT('Ctrl Pts',(-0.660114969570814,0.446797898059657,
-0.109659086918687));
#35524=CARTESIAN_POINT('Ctrl Pts',(-0.471838008872413,-0.617636643348843,
-1.13659091308131));
#35525=CARTESIAN_POINT('Ctrl Pts',(-0.369419501880207,-0.695878348939477,
-1.13306277451246));
#35526=CARTESIAN_POINT('Ctrl Pts',(-0.125014342560816,-0.800354928082894,
-1.12600649737474));
#35527=CARTESIAN_POINT('Ctrl Pts',(0.272124308982761,-0.762959459972996,
-1.11542208166817));
#35528=CARTESIAN_POINT('Ctrl Pts',(0.603201328633999,-0.540645447577443,
-1.1048376659616));
#35529=CARTESIAN_POINT('Ctrl Pts',(0.78810027446877,-0.187255136133995,
-1.09425325025503));
#35530=CARTESIAN_POINT('Ctrl Pts',(0.781928870574814,0.211520406060948,
-1.08366883454846));
#35531=CARTESIAN_POINT('Ctrl Pts',(0.586218683837755,0.559024484619848,
-1.07308441884189));
#35532=CARTESIAN_POINT('Ctrl Pts',(0.248394595446193,0.771010927419258,
-1.06250000313532));
#35533=CARTESIAN_POINT('Ctrl Pts',(-0.149640798445549,0.796094342111122,
-1.05191558742875));
#35534=CARTESIAN_POINT('Ctrl Pts',(-0.511402698585469,0.628192542158725,
-1.04133117172218));
#35535=CARTESIAN_POINT('Ctrl Pts',(-0.749192454903402,0.308008147304108,
-1.0307467560156));
#35536=CARTESIAN_POINT('Ctrl Pts',(-0.805367637396107,-0.0868419751117861,
-1.02016234030904));
#35537=CARTESIAN_POINT('Ctrl Pts',(-0.666309959555272,-0.460640287244011,
-1.00957792460246));
#35538=CARTESIAN_POINT('Ctrl Pts',(-0.365729308830473,-0.722772831593449,
-0.998993508895892));
#35539=CARTESIAN_POINT('Ctrl Pts',(0.0235094193238739,-0.809694869478827,
-0.988409093189322));
#35540=CARTESIAN_POINT('Ctrl Pts',(0.407049099987941,-0.70033528174747,
-0.97782467748275));
#35541=CARTESIAN_POINT('Ctrl Pts',(0.691914261919856,-0.421204384778775,
-0.96724026177618));
#35542=CARTESIAN_POINT('Ctrl Pts',(0.809049488131863,-0.0399675137301197,
-0.956655846069608));
#35543=CARTESIAN_POINT('Ctrl Pts',(0.730059532600631,0.350958056416477,
-0.946071430363039));
#35544=CARTESIAN_POINT('Ctrl Pts',(0.474092686589819,0.656806365662141,
-0.935487014656468));
#35545=CARTESIAN_POINT('Ctrl Pts',(0.103198983021998,0.803435403596175,
-0.924902598949896));
#35546=CARTESIAN_POINT('Ctrl Pts',(-0.292711632809765,0.755300190510068,
-0.914318183243327));
#35547=CARTESIAN_POINT('Ctrl Pts',(-0.617664755579371,0.52406939182927,
-0.903733767536755));
#35548=CARTESIAN_POINT('Ctrl Pts',(-0.792887093817242,0.165796665355035,
-0.893149351830185));
#35549=CARTESIAN_POINT('Ctrl Pts',(-0.775902242528537,-0.23266754777807,
-0.882564936123613));
#35550=CARTESIAN_POINT('Ctrl Pts',(-0.570827573064835,-0.574729814432578,
-0.871980520417042));
#35551=CARTESIAN_POINT('Ctrl Pts',(-0.227376122902373,-0.777469341192823,
-0.861396104710471));
#35552=CARTESIAN_POINT('Ctrl Pts',(0.171194556553096,-0.791739162584277,
-0.850811689003902));
#35553=CARTESIAN_POINT('Ctrl Pts',(0.528265223182337,-0.614080069485486,
-0.840227273297329));
#35554=CARTESIAN_POINT('Ctrl Pts',(0.757276832434235,-0.287559170990757,
-0.82964285759076));
#35555=CARTESIAN_POINT('Ctrl Pts',(0.802713689691629,0.108670189770389,
-0.819058441884188));
#35556=CARTESIAN_POINT('Ctrl Pts',(0.653561249881321,0.478556339855944,
-0.808474026177618));
#35557=CARTESIAN_POINT('Ctrl Pts',(0.345976200987988,0.732433577952855,
-0.797889610471047));
#35558=CARTESIAN_POINT('Ctrl Pts',(-0.0454784350531523,0.808758424814214,
-0.787305194764475));
#35559=CARTESIAN_POINT('Ctrl Pts',(-0.425908446969387,0.689028644225321,
-0.776720779057906));
#35560=CARTESIAN_POINT('Ctrl Pts',(-0.703092150301373,0.402268450101991,
-0.766136363351333));
#35561=CARTESIAN_POINT('Ctrl Pts',(-0.809836244769646,0.0179926212724667,
-0.755551947644765));
#35562=CARTESIAN_POINT('Ctrl Pts',(-0.720264432790936,-0.3706448766936,
-0.744967531938193));
#35563=CARTESIAN_POINT('Ctrl Pts',(-0.456090204684126,-0.669432747147951,
-0.734383116231622));
#35564=CARTESIAN_POINT('Ctrl Pts',(-0.081353177576358,-0.805940530226077,
-0.723798700525052));
#35565=CARTESIAN_POINT('Ctrl Pts',(0.313105025141166,-0.74707678386777,
-0.71321428481848));
#35566=CARTESIAN_POINT('Ctrl Pts',(0.631662084608202,-0.507110923399685,
-0.70262986911191));
#35567=CARTESIAN_POINT('Ctrl Pts',(0.797095206354559,-0.144214110854122,
-0.692045453405339));
#35568=CARTESIAN_POINT('Ctrl Pts',(0.769301031878132,0.253642267995893,
-0.681461037698768));
#35569=CARTESIAN_POINT('Ctrl Pts',(0.555017267217064,0.590012127717527,
-0.670876621992197));
#35570=CARTESIAN_POINT('Ctrl Pts',(0.20618936649001,0.783354595894675,-0.660292206285626));
#35571=CARTESIAN_POINT('Ctrl Pts',(-0.19262179028868,0.786800688655548,
-0.649707790579056));
#35572=CARTESIAN_POINT('Ctrl Pts',(-0.544738665839292,0.599515023750439,
-0.639123374872485));
#35573=CARTESIAN_POINT('Ctrl Pts',(-0.764803085536454,0.266898329175701,
-0.628538959165914));
#35574=CARTESIAN_POINT('Ctrl Pts',(-0.799468281674222,-0.130418343647382,
-0.617954543459343));
#35575=CARTESIAN_POINT('Ctrl Pts',(-0.640330914137975,-0.496119741758063,
-0.607370127752772));
#35576=CARTESIAN_POINT('Ctrl Pts',(-0.325968160424072,-0.741554607667303,
-0.596785712046202));
#35577=CARTESIAN_POINT('Ctrl Pts',(0.0674139447942971,-0.80722601408164,
-0.58620129633963));
#35578=CARTESIAN_POINT('Ctrl Pts',(0.444453944105533,-0.6772142713587,-0.575616880633061));
#35579=CARTESIAN_POINT('Ctrl Pts',(0.713751940666771,-0.383036088322339,
-0.565032464926489));
#35580=CARTESIAN_POINT('Ctrl Pts',(0.810026242480743,0.00399552942575511,
-0.554448049219918));
#35581=CARTESIAN_POINT('Ctrl Pts',(0.709938579680874,0.390058573606021,
-0.543863633513348));
#35582=CARTESIAN_POINT('Ctrl Pts',(0.437751635462224,0.681565832046333,
-0.533279217806777));
#35583=CARTESIAN_POINT('Ctrl Pts',(0.059447424117716,0.807851769527449,
-0.522694802100205));
#35584=CARTESIAN_POINT('Ctrl Pts',(-0.333267694403375,0.738302865787421,
-0.512110386393635));
#35585=CARTESIAN_POINT('Ctrl Pts',(-0.645193949819297,0.489778771364619,
-0.501525970687064));
#35586=CARTESIAN_POINT('Ctrl Pts',(-0.800715949546566,0.122525286796663,
-0.490941554980493));
#35587=CARTESIAN_POINT('Ctrl Pts',(-0.762132933035007,-0.274430082436886,
-0.480357139273922));
#35588=CARTESIAN_POINT('Ctrl Pts',(-0.538797976179725,-0.604859668540974,
-0.469772723567352));
#35589=CARTESIAN_POINT('Ctrl Pts',(-0.184850671743447,-0.788662606517422,
-0.459188307860781));
#35590=CARTESIAN_POINT('Ctrl Pts',(0.213907083466054,-0.781282431266632,
-0.44860389215421));
#35591=CARTESIAN_POINT('Ctrl Pts',(0.560810697474509,-0.58450820298868,
-0.438019476447639));
#35592=CARTESIAN_POINT('Ctrl Pts',(0.771765764932892,-0.246040813362946,
-0.427435060741069));
#35593=CARTESIAN_POINT('Ctrl Pts',(0.79563375560773,0.152070393899081,-0.416850645034497));
#35594=CARTESIAN_POINT('Ctrl Pts',(0.626628726655168,0.513317559307143,
-0.406266229327927));
#35595=CARTESIAN_POINT('Ctrl Pts',(0.305719918052578,0.750129195185142,
-0.395681813621356));
#35596=CARTESIAN_POINT('Ctrl Pts',(-0.089299778054571,0.805098768724973,
-0.385097397914786));
#35597=CARTESIAN_POINT('Ctrl Pts',(-0.462671928758378,0.664900867874241,
-0.374512982208214));
#35598=CARTESIAN_POINT('Ctrl Pts',(-0.723885776272764,0.363521472101407,
-0.363928566501644));
#35599=CARTESIAN_POINT('Ctrl Pts',(-0.809619342106881,-0.0259807358690177,
-0.353344150795073));
#35600=CARTESIAN_POINT('Ctrl Pts',(-0.69908958184048,-0.409184841296576,
-0.342759735088502));
#35601=CARTESIAN_POINT('Ctrl Pts',(-0.419090492574486,-0.693196679717163,
-0.332175319381931));
#35602=CARTESIAN_POINT('Ctrl Pts',(-0.0374978646661203,-0.809167713093018,
-0.32159090367536));
#35603=CARTESIAN_POINT('Ctrl Pts',(0.353184783042777,-0.728984901678733,
-0.311006487968789));
#35604=CARTESIAN_POINT('Ctrl Pts',(0.658250379547182,-0.472085707555579,
-0.300422072262219));
#35605=CARTESIAN_POINT('Ctrl Pts',(0.803746655759618,-0.100746175410848,
-0.289837656555648));
#35606=CARTESIAN_POINT('Ctrl Pts',(0.754403227182257,0.29501567283314,-0.279253240849078));
#35607=CARTESIAN_POINT('Ctrl Pts',(0.52218165351834,0.619261495923831,-0.268668825142506));
#35608=CARTESIAN_POINT('Ctrl Pts',(0.163375759383167,0.793389461681509,
-0.258084409435936));
#35609=CARTESIAN_POINT('Ctrl Pts',(-0.23503474435684,0.775188456700946,
-0.247499993729365));
#35610=CARTESIAN_POINT('Ctrl Pts',(-0.576469488299965,0.569070665635125,
-0.236915578022794));
#35611=CARTESIAN_POINT('Ctrl Pts',(-0.778159713414792,0.225001992997841,
-0.226331162316223));
#35612=CARTESIAN_POINT('Ctrl Pts',(-0.791212989161812,-0.173610385023284,
-0.215746746609652));
#35613=CARTESIAN_POINT('Ctrl Pts',(-0.612464682138537,-0.530137120397013,
-0.205162330903081));
#35614=CARTESIAN_POINT('Ctrl Pts',(-0.285246595439292,-0.758151020532607,
-0.194577915196511));
#35615=CARTESIAN_POINT('Ctrl Pts',(0.111120202088729,-0.8023782591699,-0.18399349948994));
#35616=CARTESIAN_POINT('Ctrl Pts',(0.48054820104878,-0.652097501694006,
-0.173409083783369));
#35617=CARTESIAN_POINT('Ctrl Pts',(0.73348771265382,-0.343738992654054,
-0.162824668076798));
#35618=CARTESIAN_POINT('Ctrl Pts',(0.808612851326352,0.047946819377936,
-0.152240252370227));
#35619=CARTESIAN_POINT('Ctrl Pts',(0.687731314139997,0.428009542157163,
-0.141655836663656));
#35620=CARTESIAN_POINT('Ctrl Pts',(0.400108948943148,0.704316812114863,
-0.131071420957086));
#35621=CARTESIAN_POINT('Ctrl Pts',(0.0155437137054738,0.809887134152576,
-0.120487005250515));
#35622=CARTESIAN_POINT('Ctrl Pts',(-0.372890155274553,0.71913109295302,
-0.109902589543944));
#35623=CARTESIAN_POINT('Ctrl Pts',(-0.571421157135916,0.542397737891304,
-0.10284631240623));
#35624=CARTESIAN_POINT('Ctrl Pts',(-0.643664247046206,0.435663249423622,
-0.0993181738373734));
#35625=CARTESIAN_POINT('Ctrl Pts',(-0.459778808448986,-0.601851132366388,
-1.12625));
#35626=CARTESIAN_POINT('Ctrl Pts',(-0.35997790597287,-0.678093142316895,
-1.12272186143114));
#35627=CARTESIAN_POINT('Ctrl Pts',(-0.121819235374885,-0.779899516890621,
-1.11566558429343));
#35628=CARTESIAN_POINT('Ctrl Pts',(0.265169376314341,-0.743459799348471,
-1.10508116858686));
#35629=CARTESIAN_POINT('Ctrl Pts',(0.58778475434178,-0.526827671798993,
-1.09449675288029));
#35630=CARTESIAN_POINT('Ctrl Pts',(0.767958066793962,-0.18246928341655,
-1.08391233717372));
#35631=CARTESIAN_POINT('Ctrl Pts',(0.761944391177617,0.206114383395608,
-1.07332792146715));
#35632=CARTESIAN_POINT('Ctrl Pts',(0.571236150706839,0.544736978791855,
-1.06274350576057));
#35633=CARTESIAN_POINT('Ctrl Pts',(0.242046145015631,0.751305487993936,
-1.052159090054));
#35634=CARTESIAN_POINT('Ctrl Pts',(-0.145816290148117,0.775747822655396,
-1.04157467434743));
#35635=CARTESIAN_POINT('Ctrl Pts',(-0.498332306791342,0.612137244306613,
-1.03099025864086));
#35636=CARTESIAN_POINT('Ctrl Pts',(-0.730044650361353,0.300136098188639,
-1.02040584293429));
#35637=CARTESIAN_POINT('Ctrl Pts',(-0.784784111755367,-0.0846224744286134,
-1.00982142722772));
#35638=CARTESIAN_POINT('Ctrl Pts',(-0.649280459609721,-0.448867277349673,
-0.999237011521151));
#35639=CARTESIAN_POINT('Ctrl Pts',(-0.356382026600184,-0.704300257801392,
-0.988652595814578));
#35640=CARTESIAN_POINT('Ctrl Pts',(0.0229085673489721,-0.789000748765239,
-0.97806818010801));
#35641=CARTESIAN_POINT('Ctrl Pts',(0.396645769635941,-0.682436165170634,
-0.967483764401436));
#35642=CARTESIAN_POINT('Ctrl Pts',(0.674230369135852,-0.410439274720321,
-0.956899348694867));
#35643=CARTESIAN_POINT('Ctrl Pts',(0.788371862026309,-0.0389460270134185,
-0.946314932988296));
#35644=CARTESIAN_POINT('Ctrl Pts',(0.711400725851037,0.341988296746932,
-0.935730517281725));
#35645=CARTESIAN_POINT('Ctrl Pts',(0.461975861282485,0.640019757856149,
-0.925146101575155));
#35646=CARTESIAN_POINT('Ctrl Pts',(0.100561431158107,0.782901261841897,
-0.914561685868583));
#35647=CARTESIAN_POINT('Ctrl Pts',(-0.285230530863874,0.735996284919715,
-0.903977270162013));
#35648=CARTESIAN_POINT('Ctrl Pts',(-0.601878526106637,0.510675265639743,
-0.893392854455441));
#35649=CARTESIAN_POINT('Ctrl Pts',(-0.772622544972736,0.161559246623487,
-0.882808438748871));
#35650=CARTESIAN_POINT('Ctrl Pts',(-0.756071791238701,-0.226721048051633,
-0.8722240230423));
#35651=CARTESIAN_POINT('Ctrl Pts',(-0.556238404788084,-0.56004091296378,
-0.861639607335729));
#35652=CARTESIAN_POINT('Ctrl Pts',(-0.221564861015832,-0.757598838112923,
-0.851055191629159));
#35653=CARTESIAN_POINT('Ctrl Pts',(0.166819178923374,-0.77150395248008,
-0.840470775922587));
#35654=CARTESIAN_POINT('Ctrl Pts',(0.51476386024995,-0.598385457150939,
-0.829886360216018));
#35655=CARTESIAN_POINT('Ctrl Pts',(0.737922407977915,-0.280209755277387,
-0.819301944509446));
#35656=CARTESIAN_POINT('Ctrl Pts',(0.782197993447165,0.105892805214989,
-0.808717528802876));
#35657=CARTESIAN_POINT('Ctrl Pts',(0.636857580500936,0.466325432833394,
-0.798133113096304));
#35658=CARTESIAN_POINT('Ctrl Pts',(0.337133767205639,0.7137140955303,-0.787548697389735));
#35659=CARTESIAN_POINT('Ctrl Pts',(-0.0443161006228245,0.788088237683093,
-0.776964281683162));
#35660=CARTESIAN_POINT('Ctrl Pts',(-0.415023110842466,0.67141850184181,
-0.766379865976593));
#35661=CARTESIAN_POINT('Ctrl Pts',(-0.685122573884915,0.39198730324103,
-0.75579545027002));
#35662=CARTESIAN_POINT('Ctrl Pts',(-0.789138510796985,0.0175327672081737,
-0.745211034563451));
#35663=CARTESIAN_POINT('Ctrl Pts',(-0.701855968467241,-0.361171962748737,
-0.734626618856879));
#35664=CARTESIAN_POINT('Ctrl Pts',(-0.444433485458408,-0.652323435231444,
-0.724042203150309));
#35665=CARTESIAN_POINT('Ctrl Pts',(-0.0792739591687083,-0.78534236263338,
-0.713457787443737));
#35666=CARTESIAN_POINT('Ctrl Pts',(0.305102710404415,-0.727983051487286,
-0.702873371737167));
#35667=CARTESIAN_POINT('Ctrl Pts',(0.615518112450527,-0.494150220473696,
-0.692288956030596));
#35668=CARTESIAN_POINT('Ctrl Pts',(0.776723106885605,-0.140528297430925,
-0.681704540324026));
#35669=CARTESIAN_POINT('Ctrl Pts',(0.749639293834737,0.247159697944099,
-0.671120124617454));
#35670=CARTESIAN_POINT('Ctrl Pts',(0.540832177550744,0.574932642032597,
-0.660535708910884));
#35671=CARTESIAN_POINT('Ctrl Pts',(0.200919594133975,0.763333677916742,
-0.649951293204313));
#35672=CARTESIAN_POINT('Ctrl Pts',(-0.187698777027071,0.766691695697432,
-0.639366877497742));
#35673=CARTESIAN_POINT('Ctrl Pts',(-0.530816275895666,0.584192663761808,
-0.628782461791172));
#35674=CARTESIAN_POINT('Ctrl Pts',(-0.745256305668128,0.260076961707024,
-0.618198046084601));
#35675=CARTESIAN_POINT('Ctrl Pts',(-0.779035531324328,-0.127085121407204,
-0.607613630378029));
#35676=CARTESIAN_POINT('Ctrl Pts',(-0.623965384685697,-0.483439950627678,
-0.597029214671459));
#35677=CARTESIAN_POINT('Ctrl Pts',(-0.317637090641027,-0.72260201065176,
-0.586444798964888));
#35678=CARTESIAN_POINT('Ctrl Pts',(0.0656909842520752,-0.786594992189027,
-0.575860383258318));
#35679=CARTESIAN_POINT('Ctrl Pts',(0.433094623554483,-0.659906079830351,
-0.565275967551746));
#35680=CARTESIAN_POINT('Ctrl Pts',(0.695509922128081,-0.37324648072052,
-0.554691551845176));
#35681=CARTESIAN_POINT('Ctrl Pts',(0.789323652560836,0.00389341198452167,
-0.544107136138605));
#35682=CARTESIAN_POINT('Ctrl Pts',(0.691794022736101,0.380089485852299,
-0.533522720432034));
#35683=CARTESIAN_POINT('Ctrl Pts',(0.426563612012528,0.664146423656475,
-0.522938304725463));
#35684=CARTESIAN_POINT('Ctrl Pts',(0.0579280713131272,0.787204754624109,
-0.512353889018893));
#35685=CARTESIAN_POINT('Ctrl Pts',(-0.324750063678654,0.719433376546829,
-0.501769473312321));
#35686=CARTESIAN_POINT('Ctrl Pts',(-0.628704131266004,0.477261042279714,
-0.491185057605751));
#35687=CARTESIAN_POINT('Ctrl Pts',(-0.780251311394817,0.11939379471117,
-0.48060064189918));
#35688=CARTESIAN_POINT('Ctrl Pts',(-0.742654396723939,-0.267416218983553,
-0.470016226192609));
#35689=CARTESIAN_POINT('Ctrl Pts',(-0.525027417936622,-0.589400710521857,
-0.459431810486039));
#35690=CARTESIAN_POINT('Ctrl Pts',(-0.180126272146461,-0.768506026802313,
-0.448847394779467));
#35691=CARTESIAN_POINT('Ctrl Pts',(0.208440062278693,-0.761314473516765,
-0.438262979072897));
#35692=CARTESIAN_POINT('Ctrl Pts',(0.546477539752417,-0.569569386198947,
-0.427678563366326));
#35693=CARTESIAN_POINT('Ctrl Pts',(0.752041033427039,-0.239752520718236,
-0.417094147659755));
#35694=CARTESIAN_POINT('Ctrl Pts',(0.775299007787296,0.148183790183368,
-0.406509731953184));
#35695=CARTESIAN_POINT('Ctrl Pts',(0.610613396682346,0.500198227646385,
-0.395925316246614));
#35696=CARTESIAN_POINT('Ctrl Pts',(0.297906351328608,0.730957449505267,
-0.385340900540042));
#35697=CARTESIAN_POINT('Ctrl Pts',(-0.087017461028224,0.784522114809553,
-0.374756484833472));
#35698=CARTESIAN_POINT('Ctrl Pts',(-0.450846994322672,0.647907381388134,
-0.364172069126901));
#35699=CARTESIAN_POINT('Ctrl Pts',(-0.705384757924111,0.35423061759656,
-0.353587653420331));
#35700=CARTESIAN_POINT('Ctrl Pts',(-0.788927151716197,-0.0253167221713055,
-0.343003237713759));
#35701=CARTESIAN_POINT('Ctrl Pts',(-0.681222302768388,-0.398726925828479,
-0.332418822007189));
#35702=CARTESIAN_POINT('Ctrl Pts',(-0.40837940921436,-0.675480010995328,
-0.321834406300618));
#35703=CARTESIAN_POINT('Ctrl Pts',(-0.0365394970548715,-0.788487065402779,
-0.311249990594047));
#35704=CARTESIAN_POINT('Ctrl Pts',(0.344158112861213,-0.710353560265599,
-0.300665574887476));
#35705=CARTESIAN_POINT('Ctrl Pts',(0.641426865742676,-0.460020176467796,
-0.290081159180906));
#35706=CARTESIAN_POINT('Ctrl Pts',(0.783204559045904,-0.0981713122198202,
-0.279496743474334));
#35707=CARTESIAN_POINT('Ctrl Pts',(0.735122246113328,0.287475684405229,
-0.268912327767764));
#35708=CARTESIAN_POINT('Ctrl Pts',(0.508835774002905,0.603434457081194,
-0.258327912061193));
#35709=CARTESIAN_POINT('Ctrl Pts',(0.15920021398478,0.773112073356826,-0.247743496354623));
#35710=CARTESIAN_POINT('Ctrl Pts',(-0.22902774399788,0.755376248295729,
-0.237159080648051));
#35711=CARTESIAN_POINT('Ctrl Pts',(-0.561736124377012,0.554526400266621,
-0.226574664941481));
#35712=CARTESIAN_POINT('Ctrl Pts',(-0.75827156585345,0.219251408945243,
-0.215990249234909));
#35713=CARTESIAN_POINT('Ctrl Pts',(-0.770991226958462,-0.169173263830808,
-0.205405833528339));
#35714=CARTESIAN_POINT('Ctrl Pts',(-0.596811355752582,-0.516587915656082,
-0.194821417821768));
#35715=CARTESIAN_POINT('Ctrl Pts',(-0.277956284358327,-0.738774253642469,
-0.184237002115197));
#35716=CARTESIAN_POINT('Ctrl Pts',(0.108280200302349,-0.78187113583354,
-0.173652586408627));
#35717=CARTESIAN_POINT('Ctrl Pts',(0.468266386187336,-0.635431242679951,
-0.163068170702056));
#35718=CARTESIAN_POINT('Ctrl Pts',(0.71474128873568,-0.33495373727442,-0.152483754995485));
#35719=CARTESIAN_POINT('Ctrl Pts',(0.787946384751509,0.046721398166267,
-0.141899339288914));
#35720=CARTESIAN_POINT('Ctrl Pts',(0.670154328821455,0.417070506397101,
-0.131314923582343));
#35721=CARTESIAN_POINT('Ctrl Pts',(0.389882994450752,0.686315935883678,
-0.120730507875773));
#35722=CARTESIAN_POINT('Ctrl Pts',(0.0151464486370091,0.789188099552883,
-0.110146092169201));
#35723=CARTESIAN_POINT('Ctrl Pts',(-0.363359856668207,0.700751594443855,
-0.0995616764626311));
#35724=CARTESIAN_POINT('Ctrl Pts',(-0.55681681808202,0.528535177208507,
-0.0925053993249171));
#35725=CARTESIAN_POINT('Ctrl Pts',(-0.627213524521598,0.424528600787587,
-0.0889772607560602));
#35726=CARTESIAN_POINT('',(-0.676565692095423,0.457932546695692,-0.12));
#35727=CARTESIAN_POINT('Ctrl Pts',(0.351315334519666,0.671030718912565,
-0.12));
#35728=CARTESIAN_POINT('Ctrl Pts',(0.320499669985565,0.689321131271856,
-0.12));
#35729=CARTESIAN_POINT('Ctrl Pts',(0.288470314380151,0.705335580149119,
-0.12));
#35730=CARTESIAN_POINT('Ctrl Pts',(0.255512129576424,0.719045430115912,
-0.12));
#35731=CARTESIAN_POINT('Ctrl Pts',(0.22214779681421,0.732924228330563,-0.12));
#35732=CARTESIAN_POINT('Ctrl Pts',(0.187830516460429,0.744441808855943,
-0.12));
#35733=CARTESIAN_POINT('Ctrl Pts',(0.1528242686584,0.753525280825841,-0.12));
#35734=CARTESIAN_POINT('Ctrl Pts',(0.126989719984013,0.760228866998969,
-0.12));
#35735=CARTESIAN_POINT('Ctrl Pts',(0.100779187652097,0.765605880524251,
-0.12));
#35736=CARTESIAN_POINT('Ctrl Pts',(0.0742933277395626,0.76960959177323,
-0.12));
#35737=CARTESIAN_POINT('Ctrl Pts',(0.0666757152815714,0.770761101325464,
-0.12));
#35738=CARTESIAN_POINT('Ctrl Pts',(0.0590433060649341,0.771797653690197,
-0.12));
#35739=CARTESIAN_POINT('Ctrl Pts',(0.0514033585110513,0.772718183814392,
-0.12));
#35740=CARTESIAN_POINT('Ctrl Pts',(0.0392486607751243,0.774182691958918,
-0.12));
#35741=CARTESIAN_POINT('Ctrl Pts',(0.0270711318454161,0.775354140672433,
-0.12));
#35742=CARTESIAN_POINT('Ctrl Pts',(0.0148810082990363,0.776230637396706,
-0.12));
#35743=CARTESIAN_POINT('Ctrl Pts',(-0.0215690645837374,0.778851477895959,
-0.12));
#35744=CARTESIAN_POINT('Ctrl Pts',(-0.0581308241833953,0.778839173851118,
-0.12));
#35745=CARTESIAN_POINT('Ctrl Pts',(-0.0945366085257304,0.776289317214896,
-0.119999999999999));
#35746=CARTESIAN_POINT('Ctrl Pts',(-0.121214846927138,0.774420776694223,
-0.119999999999999));
#35747=CARTESIAN_POINT('Ctrl Pts',(-0.147809835066355,0.771188449071313,
-0.12));
#35748=CARTESIAN_POINT('Ctrl Pts',(-0.174217694473203,0.766612275855432,
-0.12));
#35749=CARTESIAN_POINT('Ctrl Pts',(-0.190197279886907,0.763843200572029,
-0.12));
#35750=CARTESIAN_POINT('Ctrl Pts',(-0.206108346383167,0.760581783987635,
-0.12));
#35751=CARTESIAN_POINT('Ctrl Pts',(-0.221927418745588,0.756829859540378,
-0.12));
#35752=CARTESIAN_POINT('Ctrl Pts',(-0.229467360158877,0.755041556795989,
-0.12));
#35753=CARTESIAN_POINT('Ctrl Pts',(-0.236985877671306,0.753141777075834,
-0.12));
#35754=CARTESIAN_POINT('Ctrl Pts',(-0.244467321374769,0.751134526250689,
-0.12));
#35755=CARTESIAN_POINT('Ctrl Pts',(-0.280535878868674,0.7414574312058,-0.12));
#35756=CARTESIAN_POINT('Ctrl Pts',(-0.315822129998283,0.729268499598691,
-0.12));
#35757=CARTESIAN_POINT('Ctrl Pts',(-0.350052129487708,0.714644278109736,
-0.12));
#35758=CARTESIAN_POINT('Ctrl Pts',(-0.355634194416505,0.712259429874209,
-0.12));
#35759=CARTESIAN_POINT('Ctrl Pts',(-0.361188160016036,0.709809706699139,
-0.12));
#35760=CARTESIAN_POINT('Ctrl Pts',(-0.366712818974203,0.707295310693253,
-0.12));
#35761=CARTESIAN_POINT('Ctrl Pts',(-0.397138122868593,0.693448073575234,
-0.12));
#35762=CARTESIAN_POINT('Ctrl Pts',(-0.426675742611669,0.677641907045338,
-0.12));
#35763=CARTESIAN_POINT('Ctrl Pts',(-0.455180005223245,0.66000787905436,
-0.12));
#35764=CARTESIAN_POINT('Ctrl Pts',(-0.461866014446751,0.65587161089679,
-0.12));
#35765=CARTESIAN_POINT('Ctrl Pts',(-0.468495101116925,0.651634643173702,
-0.12));
#35766=CARTESIAN_POINT('Ctrl Pts',(-0.475065246040253,0.647298434119057,
-0.12));
#35767=CARTESIAN_POINT('Ctrl Pts',(-0.481997163117426,0.642723460211044,
-0.12));
#35768=CARTESIAN_POINT('Ctrl Pts',(-0.488856348552518,0.638042668308952,
-0.12));
#35769=CARTESIAN_POINT('Ctrl Pts',(-0.495637685263811,0.633260662354593,
-0.12));
#35770=CARTESIAN_POINT('Ctrl Pts',(-0.526421712127851,0.611552641350735,
-0.12));
#35771=CARTESIAN_POINT('Ctrl Pts',(-0.555624158844379,0.587748863949367,
-0.12));
#35772=CARTESIAN_POINT('Ctrl Pts',(-0.583051806437047,0.562054023979174,
-0.12));
#35773=CARTESIAN_POINT('Ctrl Pts',(-0.610463295407308,0.536374321771544,
-0.12));
#35774=CARTESIAN_POINT('Ctrl Pts',(-0.636103059505849,0.50880506281788,
-0.12));
#35775=CARTESIAN_POINT('Ctrl Pts',(-0.659749387717314,0.479508356594237,
-0.12));
#35776=CARTESIAN_POINT('Ctrl Pts',(-0.665472951279087,0.472417126246673,
-0.12));
#35777=CARTESIAN_POINT('Ctrl Pts',(-0.671079552778587,0.465224522959082,
-0.12));
#35778=CARTESIAN_POINT('Ctrl Pts',(-0.676565692095422,0.457932546695692,
-0.12));
#35779=CARTESIAN_POINT('Ctrl Pts',(0.589349009255749,-0.565869316348656,
-1.12625));
#35780=CARTESIAN_POINT('Ctrl Pts',(0.595826955511021,-0.559130415243379,
-1.12600649737474));
#35781=CARTESIAN_POINT('Ctrl Pts',(0.694346705276116,-0.453008535243727,
-1.12223485618063));
#35782=CARTESIAN_POINT('Ctrl Pts',(0.828384689818385,-0.196826841568886,
-1.11493507641766));
#35783=CARTESIAN_POINT('Ctrl Pts',(0.821897829369206,0.222332451391628,
-1.10435066071109));
#35784=CARTESIAN_POINT('Ctrl Pts',(0.616183750099589,0.587599496275833,
-1.09376624500451));
#35785=CARTESIAN_POINT('Ctrl Pts',(0.261091496307317,0.810421806269904,
-1.08318182929794));
#35786=CARTESIAN_POINT('Ctrl Pts',(-0.157289815040412,0.836787381022574,
-1.07259741359137));
#35787=CARTESIAN_POINT('Ctrl Pts',(-0.537543482173721,0.660303137862947,
-1.0620129978848));
#35788=CARTESIAN_POINT('Ctrl Pts',(-0.7874880639875,0.323752245535046,-1.05142858217823));
#35789=CARTESIAN_POINT('Ctrl Pts',(-0.846534688677586,-0.0912809764781306,
-1.04084416647166));
#35790=CARTESIAN_POINT('Ctrl Pts',(-0.700368959446377,-0.484186307032688,
-1.03025975076509));
#35791=CARTESIAN_POINT('Ctrl Pts',(-0.38442387329105,-0.759717979177561,
-1.01967533505852));
#35792=CARTESIAN_POINT('Ctrl Pts',(0.0247111232736773,-0.851083110906004,
-1.00909091935195));
#35793=CARTESIAN_POINT('Ctrl Pts',(0.42785576069194,-0.736133514901142,
-0.998506503645377));
#35794=CARTESIAN_POINT('Ctrl Pts',(0.727282047487868,-0.442734604895683,
-0.987922087938807));
#35795=CARTESIAN_POINT('Ctrl Pts',(0.850404740342968,-0.0420104871635215,
-0.977337672232236));
#35796=CARTESIAN_POINT('Ctrl Pts',(0.767377146099821,0.368897575755567,
-0.966753256525664));
#35797=CARTESIAN_POINT('Ctrl Pts',(0.498326337204486,0.690379581274127,
-0.956168840819095));
#35798=CARTESIAN_POINT('Ctrl Pts',(0.108474086749781,0.844503687104731,
-0.945584425112522));
#35799=CARTESIAN_POINT('Ctrl Pts',(-0.307673836701548,0.793908001690772,
-0.935000009405953));
#35800=CARTESIAN_POINT('Ctrl Pts',(-0.649237214524841,0.550857644208324,
-0.924415593699381));
#35801=CARTESIAN_POINT('Ctrl Pts',(-0.833416191506255,0.174271502818131,
-0.913831177992811));
#35802=CARTESIAN_POINT('Ctrl Pts',(-0.815563145108209,-0.244560547230945,
-0.90324676228624));
#35803=CARTESIAN_POINT('Ctrl Pts',(-0.600005909618337,-0.604107617370174,
-0.892662346579669));
#35804=CARTESIAN_POINT('Ctrl Pts',(-0.238998646675454,-0.817210347352623,
-0.882077930873097));
#35805=CARTESIAN_POINT('Ctrl Pts',(0.17994531181254,-0.832209582792671,
-0.871493515166529));
#35806=CARTESIAN_POINT('Ctrl Pts',(0.555267949047113,-0.64546929415458,
-0.860909099459956));
#35807=CARTESIAN_POINT('Ctrl Pts',(0.795985681346874,-0.302258002417496,
-0.850324683753387));
#35808=CARTESIAN_POINT('Ctrl Pts',(0.843745082180559,0.114224958881187,
-0.839740268046815));
#35809=CARTESIAN_POINT('Ctrl Pts',(0.686968588642089,0.503018153901045,
-0.829155852340245));
#35810=CARTESIAN_POINT('Ctrl Pts',(0.363661068552687,0.769872542797965,
-0.818571436633673));
#35811=CARTESIAN_POINT('Ctrl Pts',(-0.047803103913807,0.850098799076459,
-0.807987020927103));
#35812=CARTESIAN_POINT('Ctrl Pts',(-0.447679119223231,0.724248928992339,
-0.797402605220532));
#35813=CARTESIAN_POINT('Ctrl Pts',(-0.739031303134287,0.422830743823914,
-0.786818189513961));
#35814=CARTESIAN_POINT('Ctrl Pts',(-0.85123171271497,0.0189123294010521,
-0.776233773807391));
#35815=CARTESIAN_POINT('Ctrl Pts',(-0.757081361438328,-0.389590704583327,
-0.765649358100819));
#35816=CARTESIAN_POINT('Ctrl Pts',(-0.479403643135562,-0.703651370980965,
-0.755064942394249));
#35817=CARTESIAN_POINT('Ctrl Pts',(-0.0855116143916565,-0.847136865411472,
-0.744480526687678));
#35818=CARTESIAN_POINT('Ctrl Pts',(0.329109654614668,-0.785264248628737,
-0.733896110981106));
#35819=CARTESIAN_POINT('Ctrl Pts',(0.663950028923553,-0.533032329251663,
-0.723311695274536));
#35820=CARTESIAN_POINT('Ctrl Pts',(0.837839405292465,-0.151585737700515,
-0.712727279567964));
#35821=CARTESIAN_POINT('Ctrl Pts',(0.808624507964925,0.266607408099481,
-0.702142863861395));
#35822=CARTESIAN_POINT('Ctrl Pts',(0.583387446549703,0.620171099087388,
-0.691558448154823));
#35823=CARTESIAN_POINT('Ctrl Pts',(0.216728911202081,0.82339643185054,-0.680974032448252));
#35824=CARTESIAN_POINT('Ctrl Pts',(-0.202467816811898,0.82701867457178,
-0.670389616741683));
#35825=CARTESIAN_POINT('Ctrl Pts',(-0.572583445726543,0.6301597437277,-0.659805201035111));
#35826=CARTESIAN_POINT('Ctrl Pts',(-0.803896645273107,0.280541064113054,
-0.64922078532854));
#35827=CARTESIAN_POINT('Ctrl Pts',(-0.840333782374013,-0.137084788127738,
-0.63863636962197));
#35828=CARTESIAN_POINT('Ctrl Pts',(-0.67306197304253,-0.521479324018831,
-0.628051953915399));
#35829=CARTESIAN_POINT('Ctrl Pts',(-0.342630299990165,-0.779459801698388,
-0.617467538208828));
#35830=CARTESIAN_POINT('Ctrl Pts',(0.0708598658787424,-0.848488057866867,
-0.606883122502257));
#35831=CARTESIAN_POINT('Ctrl Pts',(0.467172585207631,-0.7118306544154,-0.596298706795686));
#35832=CARTESIAN_POINT('Ctrl Pts',(0.750235977744155,-0.402615303525977,
-0.585714291089116));
#35833=CARTESIAN_POINT('Ctrl Pts',(0.851431422320551,0.00419976430822168,
-0.575129875382545));
#35834=CARTESIAN_POINT('Ctrl Pts',(0.746227693570422,0.409996749113464,
-0.564545459675974));
#35835=CARTESIAN_POINT('Ctrl Pts',(0.460127682361612,0.716404648826047,
-0.553961043969404));
#35836=CARTESIAN_POINT('Ctrl Pts',(0.0624861297268952,0.849145799334128,
-0.543376628262831));
#35837=CARTESIAN_POINT('Ctrl Pts',(-0.350302955852819,0.776041844268606,
-0.532792212556262));
#35838=CARTESIAN_POINT('Ctrl Pts',(-0.67817358692588,0.514814229534427,
-0.522207796849691));
#35839=CARTESIAN_POINT('Ctrl Pts',(-0.841645225850065,0.12878827096765,
-0.511623381143119));
#35840=CARTESIAN_POINT('Ctrl Pts',(-0.80109000565714,-0.288457809343551,
-0.501038965436549));
#35841=CARTESIAN_POINT('Ctrl Pts',(-0.566339092665934,-0.635777584579208,
-0.490454549729978));
#35842=CARTESIAN_POINT('Ctrl Pts',(-0.194299470937418,-0.82897576594764,
-0.479870134023407));
#35843=CARTESIAN_POINT('Ctrl Pts',(0.224841125840774,-0.821218346766367,
-0.469285718316837));
#35844=CARTESIAN_POINT('Ctrl Pts',(0.589477012918694,-0.614385836568145,
-0.458701302610266));
#35845=CARTESIAN_POINT('Ctrl Pts',(0.811215227944597,-0.258617398652365,
-0.448116886903695));
#35846=CARTESIAN_POINT('Ctrl Pts',(0.8363032512486,0.159843601330507,-0.437532471197124));
#35847=CARTESIAN_POINT('Ctrl Pts',(0.658659386600812,0.539556222628657,
-0.426948055490553));
#35848=CARTESIAN_POINT('Ctrl Pts',(0.321347051500517,0.788472686544893,
-0.416363639783983));
#35849=CARTESIAN_POINT('Ctrl Pts',(-0.0938644121072648,0.846252076555809,
-0.405779224077412));
#35850=CARTESIAN_POINT('Ctrl Pts',(-0.48632179762979,0.698887840846459,
-0.395194808370841));
#35851=CARTESIAN_POINT('Ctrl Pts',(-0.760887812970069,0.382103181111099,
-0.38461039266427));
#35852=CARTESIAN_POINT('Ctrl Pts',(-0.851003722888249,-0.0273087632644408,
-0.374025976957699));
#35853=CARTESIAN_POINT('Ctrl Pts',(-0.734824139984663,-0.43010067223277,
-0.363441561251128));
#35854=CARTESIAN_POINT('Ctrl Pts',(-0.440512659294738,-0.728630017160833,
-0.352857145544558));
#35855=CARTESIAN_POINT('Ctrl Pts',(-0.0394145998886176,-0.850529008473494,
-0.342272729837987));
#35856=CARTESIAN_POINT('Ctrl Pts',(0.371238123405903,-0.766247584505002,
-0.331688314131416));
#35857=CARTESIAN_POINT('Ctrl Pts',(0.691897407156195,-0.496216769731146,
-0.321103898424845));
#35858=CARTESIAN_POINT('Ctrl Pts',(0.844830849187047,-0.105895901792902,
-0.310519482718274));
#35859=CARTESIAN_POINT('Ctrl Pts',(0.792965189320117,0.310095649688961,
-0.299935067011704));
#35860=CARTESIAN_POINT('Ctrl Pts',(0.548873412549209,0.650915573609104,
-0.289350651305133));
#35861=CARTESIAN_POINT('Ctrl Pts',(0.171726850179941,0.833944238330876,
-0.278766235598562));
#35862=CARTESIAN_POINT('Ctrl Pts',(-0.247048745074761,0.814812873511381,
-0.268181819891991));
#35863=CARTESIAN_POINT('Ctrl Pts',(-0.605936216145871,0.598159196372131,
-0.257597404185421));
#35864=CARTESIAN_POINT('Ctrl Pts',(-0.817936008537478,0.236503161103038,
-0.247012988478849));
#35865=CARTESIAN_POINT('Ctrl Pts',(-0.831656513568513,-0.182484627408237,
-0.236428572772279));
#35866=CARTESIAN_POINT('Ctrl Pts',(-0.643771334910445,-0.557235529878874,
-0.225844157065708));
#35867=CARTESIAN_POINT('Ctrl Pts',(-0.29982721760122,-0.796904554312883,
-0.215259741359137));
#35868=CARTESIAN_POINT('Ctrl Pts',(0.116800205661488,-0.843392505842622,
-0.204675325652567));
#35869=CARTESIAN_POINT('Ctrl Pts',(0.50511183077167,-0.685430019722115,
-0.194090909945995));
#35870=CARTESIAN_POINT('Ctrl Pts',(0.770980560490097,-0.361309503413322,
-0.183506494239425));
#35871=CARTESIAN_POINT('Ctrl Pts',(0.849945784476039,0.0503976618012751,
-0.172922078532854));
#35872=CARTESIAN_POINT('Ctrl Pts',(0.722885284777081,0.449887613677287,
-0.162337662826283));
#35873=CARTESIAN_POINT('Ctrl Pts',(0.42056085792794,0.740318564577236,-0.151753247119712));
#35874=CARTESIAN_POINT('Ctrl Pts',(0.0163382438424028,0.85128520335196,
-0.141168831413141));
#35875=CARTESIAN_POINT('Ctrl Pts',(-0.391950752487246,0.755890089971351,
-0.130584415706571));
#35876=CARTESIAN_POINT('Ctrl Pts',(-0.600629835243707,0.5701228592569,-0.123528138568857));
#35877=CARTESIAN_POINT('Ctrl Pts',(-0.676565692095422,0.457932546695692,
-0.12));
#35878=CARTESIAN_POINT('Ctrl Pts',(0.589301091561372,-0.565833523687256,
-1.12625));
#35879=CARTESIAN_POINT('Ctrl Pts',(0.681795706363589,-0.469502756447982,
-1.12277201246584));
#35880=CARTESIAN_POINT('Ctrl Pts',(0.81857564756759,-0.230726286157592,
-1.11581603739752));
#35881=CARTESIAN_POINT('Ctrl Pts',(0.83073247791742,0.182054083126401,-1.10538207479504));
#35882=CARTESIAN_POINT('Ctrl Pts',(0.647100797261751,0.551826151980982,
-1.09494811219256));
#35883=CARTESIAN_POINT('Ctrl Pts',(0.310930583933833,0.79157490921723,-1.08451414959008));
#35884=CARTESIAN_POINT('Ctrl Pts',(-0.0985234799625354,0.844718114599206,
-1.0740801869876));
#35885=CARTESIAN_POINT('Ctrl Pts',(-0.48475737907202,0.698765466281198,
-1.06364622438511));
#35886=CARTESIAN_POINT('Ctrl Pts',(-0.756728010910768,0.388101050966165,
-1.05321226178264));
#35887=CARTESIAN_POINT('Ctrl Pts',(-0.850331447180054,-0.0140392876955771,
-1.04277829918015));
#35888=CARTESIAN_POINT('Ctrl Pts',(-0.743503406614721,-0.412872032986844,
-1.03234433657767));
#35889=CARTESIAN_POINT('Ctrl Pts',(-0.461424807647817,-0.714386145646102,
-1.02191037397519));
#35890=CARTESIAN_POINT('Ctrl Pts',(-0.0705839504414228,-0.847513141979658,
-1.01147641137271));
#35891=CARTESIAN_POINT('Ctrl Pts',(0.336894159842277,-0.780873113300908,
-1.00104244877023));
#35892=CARTESIAN_POINT('Ctrl Pts',(0.664963173900133,-0.530174058353571,
-0.990608486167752));
#35893=CARTESIAN_POINT('Ctrl Pts',(0.836294104630413,-0.154507939527313,
-0.980174523565271));
#35894=CARTESIAN_POINT('Ctrl Pts',(0.810502659647234,0.257577125376117,
-0.96974056096279));
#35895=CARTESIAN_POINT('Ctrl Pts',(0.59366811553693,0.608948854591686,-0.95930659836031));
#35896=CARTESIAN_POINT('Ctrl Pts',(0.236900417487042,0.816785607236096,
-0.94887263575783));
#35897=CARTESIAN_POINT('Ctrl Pts',(-0.175706936751581,0.832098317777405,
-0.938438673155349));
#35898=CARTESIAN_POINT('Ctrl Pts',(-0.546898513860029,0.651277630891634,
-0.928004710552868));
#35899=CARTESIAN_POINT('Ctrl Pts',(-0.789180970390855,0.316944685067354,
-0.917570747950387));
#35900=CARTESIAN_POINT('Ctrl Pts',(-0.845446053461757,-0.092095102919769,
-0.907136785347907));
#35901=CARTESIAN_POINT('Ctrl Pts',(-0.702431554241402,-0.479427209172021,
-0.896702822745427));
#35902=CARTESIAN_POINT('Ctrl Pts',(-0.39384733450868,-0.753753815530977,
-0.886268860142945));
#35903=CARTESIAN_POINT('Ctrl Pts',(0.00757040428266388,-0.850413561905815,
-0.875834897540466));
#35904=CARTESIAN_POINT('Ctrl Pts',(0.407203727626896,-0.746622837529435,
-0.865400934937985));
#35905=CARTESIAN_POINT('Ctrl Pts',(0.71085530448089,-0.466846091764925,
-0.854966972335503));
#35906=CARTESIAN_POINT('Ctrl Pts',(0.846951603734271,-0.0770293336317683,
-0.844533009733024));
#35907=CARTESIAN_POINT('Ctrl Pts',(0.783413448288196,0.330943962550494,
-0.834099047130542));
#35908=CARTESIAN_POINT('Ctrl Pts',(0.535217378667919,0.66091065574617,-0.823665084528063));
#35909=CARTESIAN_POINT('Ctrl Pts',(0.160865541628771,0.83509449454775,-0.813231121925581));
#35910=CARTESIAN_POINT('Ctrl Pts',(-0.251403815775338,0.812438710747312,
-0.802797159323101));
#35911=CARTESIAN_POINT('Ctrl Pts',(-0.604414930500539,0.598283485561275,
-0.79236319672062));
#35912=CARTESIAN_POINT('Ctrl Pts',(-0.814959764354287,0.243107218714002,
-0.78192923411814));
#35913=CARTESIAN_POINT('Ctrl Pts',(-0.833410920788056,-0.169371704893341,
-0.771495271515659));
#35914=CARTESIAN_POINT('Ctrl Pts',(-0.655419288781807,-0.541928125492692,
-0.76106130891318));
#35915=CARTESIAN_POINT('Ctrl Pts',(-0.322939169195012,-0.786746992562985,
-0.750627346310697));
#35916=CARTESIAN_POINT('Ctrl Pts',(0.0856607483339354,-0.846122197736321,
-0.740193383708219));
#35917=CARTESIAN_POINT('Ctrl Pts',(0.47406962223381,-0.706058447001635,
-0.729759421105735));
#35918=CARTESIAN_POINT('Ctrl Pts',(0.750735829721,-0.399570083064777,-0.719325458503257));
#35919=CARTESIAN_POINT('Ctrl Pts',(0.850446544913026,0.00110070557588867,
-0.708891495900775));
#35920=CARTESIAN_POINT('Ctrl Pts',(0.749699014916821,0.401512047565224,
-0.698457533298295));
#35921=CARTESIAN_POINT('Ctrl Pts',(0.472240379621288,0.707283225562725,
-0.688023570695814));
#35922=CARTESIAN_POINT('Ctrl Pts',(0.083470247592485,0.84634109853777,-0.677589608093334));
#35923=CARTESIAN_POINT('Ctrl Pts',(-0.32497460644901,0.785908418628138,
-0.667155645490853));
#35924=CARTESIAN_POINT('Ctrl Pts',(-0.656819890853628,0.540229736580928,
-0.656721682888372));
#35925=CARTESIAN_POINT('Ctrl Pts',(-0.83384655260312,0.167213827236748,
-0.646287720285892));
#35926=CARTESIAN_POINT('Ctrl Pts',(-0.81432774339868,-0.24521595306685,
-0.635853757683412));
#35927=CARTESIAN_POINT('Ctrl Pts',(-0.602864230054738,-0.59984602810036,
-0.62541979508093));
#35928=CARTESIAN_POINT('Ctrl Pts',(-0.249299950511683,-0.813086755507764,
-0.614985832478451));
#35929=CARTESIAN_POINT('Ctrl Pts',(0.163026670890489,-0.834675291287357,
-0.604551869875969));
#35930=CARTESIAN_POINT('Ctrl Pts',(0.536926373445071,-0.659523014614649,
-0.59411790727349));
#35931=CARTESIAN_POINT('Ctrl Pts',(0.784267482446793,-0.328914963605851,
-0.583683944671008));
#35932=CARTESIAN_POINT('Ctrl Pts',(0.846749373394363,0.0792214362626901,
-0.573249982068528));
#35933=CARTESIAN_POINT('Ctrl Pts',(0.709644477235602,0.468684598889571,
-0.562816019466046));
#35934=CARTESIAN_POINT('Ctrl Pts',(0.40526970683834,0.74767439572747,-0.552382056863567));
#35935=CARTESIAN_POINT('Ctrl Pts',(0.00536905683500232,0.850430309041236,
-0.541948094261085));
#35936=CARTESIAN_POINT('Ctrl Pts',(-0.395797130335717,0.752731804114374,
-0.531514131658606));
#35937=CARTESIAN_POINT('Ctrl Pts',(-0.703670213228203,0.47760733696484,
-0.521080169056124));
#35938=CARTESIAN_POINT('Ctrl Pts',(-0.845681612069302,0.0899063307845227,
-0.510646206453645));
#35939=CARTESIAN_POINT('Ctrl Pts',(-0.788357905185791,-0.318986442718713,
-0.500212243851163));
#35940=CARTESIAN_POINT('Ctrl Pts',(-0.54521082915687,-0.652691113067545,
-0.489778281248683));
#35941=CARTESIAN_POINT('Ctrl Pts',(-0.173552435486476,-0.832550352497661,
-0.479344318646202));
#35942=CARTESIAN_POINT('Ctrl Pts',(0.239013898693351,-0.816169647523525,
-0.468910356043722));
#35943=CARTESIAN_POINT('Ctrl Pts',(0.595242410120835,-0.607410084292985,
-0.458476393441241));
#35944=CARTESIAN_POINT('Ctrl Pts',(0.811166689955886,-0.255478254286475,
-0.448042430838761));
#35945=CARTESIAN_POINT('Ctrl Pts',(0.835891355663179,0.156672201857554,
-0.43760846823628));
#35946=CARTESIAN_POINT('Ctrl Pts',(0.663588571113166,0.531893547239614,
-0.4271745056338));
#35947=CARTESIAN_POINT('Ctrl Pts',(0.334871722342651,0.781742583516305,
-0.416740543031318));
#35948=CARTESIAN_POINT('Ctrl Pts',(-0.0727775393183068,0.847327544151471,
-0.406306580428838));
#35949=CARTESIAN_POINT('Ctrl Pts',(-0.463272450821894,0.713189437398579,
-0.395872617826357));
#35950=CARTESIAN_POINT('Ctrl Pts',(-0.744569690714111,0.410945875971156,
-0.385438655223877));
#35951=CARTESIAN_POINT('Ctrl Pts',(-0.850364855236199,0.0118385085176672,
-0.375004692621396));
#35952=CARTESIAN_POINT('Ctrl Pts',(-0.755721029601024,-0.390059306686192,
-0.364570730018916));
#35953=CARTESIAN_POINT('Ctrl Pts',(-0.482946653183774,-0.700016476572465,
-0.354136767416435));
#35954=CARTESIAN_POINT('Ctrl Pts',(-0.0963372107351888,-0.844973182506322,
-0.343702804813955));
#35955=CARTESIAN_POINT('Ctrl Pts',(0.312979817940913,-0.790761766178751,
-0.333268842211474));
#35956=CARTESIAN_POINT('Ctrl Pts',(0.648524561294595,-0.550160368159608,
-0.322834879608994));
#35957=CARTESIAN_POINT('Ctrl Pts',(0.831205969332431,-0.179880999456948,
-0.312400917006512));
#35958=CARTESIAN_POINT('Ctrl Pts',(0.817964316356762,0.232798011437263,
-0.301966954404033));
#35959=CARTESIAN_POINT('Ctrl Pts',(0.611920785515871,0.590604343299513,
-0.291532991801551));
#35960=CARTESIAN_POINT('Ctrl Pts',(0.261641771830851,0.809199678217179,
-0.281099029199071));
#35961=CARTESIAN_POINT('Ctrl Pts',(-0.150308664289153,0.837059044723434,
-0.27066506659659));
#35962=CARTESIAN_POINT('Ctrl Pts',(-0.526829940633294,0.667615720654169,
-0.26023110399411));
#35963=CARTESIAN_POINT('Ctrl Pts',(-0.779172437010209,0.340809105248279,
-0.249797141391629));
#35964=CARTESIAN_POINT('Ctrl Pts',(-0.847856686154441,-0.0663294394492015,
-0.239363178789149));
#35965=CARTESIAN_POINT('Ctrl Pts',(-0.716693103442292,-0.457833473536331,
-0.228929216186668));
#35966=CARTESIAN_POINT('Ctrl Pts',(-0.416598299086146,-0.741421929191928,
-0.218495253584187));
#35967=CARTESIAN_POINT('Ctrl Pts',(-0.0183072020772304,-0.850250118821527,
-0.208061290981707));
#35968=CARTESIAN_POINT('Ctrl Pts',(0.384298765226853,-0.758666652961298,
-0.197627328379226));
#35969=CARTESIAN_POINT('Ctrl Pts',(0.696322509060588,-0.488257754713524,
-0.187193365776746));
#35970=CARTESIAN_POINT('Ctrl Pts',(0.84421529649218,-0.102763035312453,
-0.176759403174265));
#35971=CARTESIAN_POINT('Ctrl Pts',(0.793120952222846,0.306956102035912,
-0.166325440571785));
#35972=CARTESIAN_POINT('Ctrl Pts',(0.555075924815366,0.644318467007061,
-0.155891477969304));
#35973=CARTESIAN_POINT('Ctrl Pts',(0.186203366191313,0.829817432539668,
-0.145457515366823));
#35974=CARTESIAN_POINT('Ctrl Pts',(-0.226576956355161,0.819703865231683,
-0.135023552764343));
#35975=CARTESIAN_POINT('Ctrl Pts',(-0.585915510641057,0.616411513065778,
-0.124589590161862));
#35976=CARTESIAN_POINT('Ctrl Pts',(-0.80722132928804,0.267758165995405,
-0.114155627559381));
#35977=CARTESIAN_POINT('Ctrl Pts',(-0.827788619517399,-0.00665018237018045,
-0.107199652491061));
#35978=CARTESIAN_POINT('Ctrl Pts',(-0.805186023504942,-0.138270823372324,
-0.103721664956901));
#35979=CARTESIAN_POINT('Ctrl Pts',(0.591130873629677,-0.567590438870538,
-1.12757052310292));
#35980=CARTESIAN_POINT('Ctrl Pts',(0.683912652131224,-0.470960598009098,
-1.12409253556876));
#35981=CARTESIAN_POINT('Ctrl Pts',(0.821117344248753,-0.23144266899012,
-1.11713656050044));
#35982=CARTESIAN_POINT('Ctrl Pts',(0.833311893543813,0.182619350617632,
-1.10670259789796));
#35983=CARTESIAN_POINT('Ctrl Pts',(0.64911004990092,0.553539577591926,-1.09626863529548));
#35984=CARTESIAN_POINT('Ctrl Pts',(0.31189602120762,0.794032746862491,-1.085834672693));
#35985=CARTESIAN_POINT('Ctrl Pts',(-0.0988293942380984,0.847340965934937,
-1.07540071009052));
#35986=CARTESIAN_POINT('Ctrl Pts',(-0.486262551456742,0.7009351325576,-1.06496674748804));
#35987=CARTESIAN_POINT('Ctrl Pts',(-0.759077651294708,0.389306105187746,
-1.05453278488556));
#35988=CARTESIAN_POINT('Ctrl Pts',(-0.85297172671121,-0.0140828798662705,
-1.04409882228308));
#35989=CARTESIAN_POINT('Ctrl Pts',(-0.745811984820572,-0.414154000672732,
-1.0336648596806));
#35990=CARTESIAN_POINT('Ctrl Pts',(-0.462857531842693,-0.716604314872263,
-1.02323089707812));
#35991=CARTESIAN_POINT('Ctrl Pts',(-0.0708031136070292,-0.850144670496582,
-1.01279693447564));
#35992=CARTESIAN_POINT('Ctrl Pts',(0.337940216291634,-0.783297724545797,
-1.00236297187316));
#35993=CARTESIAN_POINT('Ctrl Pts',(0.667027884744334,-0.531820248945421,
-0.991929009270677));
#35994=CARTESIAN_POINT('Ctrl Pts',(0.838890798054125,-0.154987686725405,
-0.981495046668197));
#35995=CARTESIAN_POINT('Ctrl Pts',(0.813019270631117,0.258376902423277,
-0.971061084065716));
#35996=CARTESIAN_POINT('Ctrl Pts',(0.595511455199308,0.61083964095294,-0.960627121463235));
#35997=CARTESIAN_POINT('Ctrl Pts',(0.237635993349256,0.819321726773046,
-0.950193158860755));
#35998=CARTESIAN_POINT('Ctrl Pts',(-0.176252506839004,0.834681983284209,
-0.939759196258274));
#35999=CARTESIAN_POINT('Ctrl Pts',(-0.548596633896848,0.653299848115922,
-0.929325233655793));
#36000=CARTESIAN_POINT('Ctrl Pts',(-0.791631377522398,0.31792879840216,
-0.918891271053313));
#36001=CARTESIAN_POINT('Ctrl Pts',(-0.848071163691739,-0.092381058239798,
-0.908457308450832));
#36002=CARTESIAN_POINT('Ctrl Pts',(-0.704612604411756,-0.480915830789212,
-0.898023345848352));
#36003=CARTESIAN_POINT('Ctrl Pts',(-0.395070230591335,-0.756094221336823,
-0.887589383245871));
#36004=CARTESIAN_POINT('Ctrl Pts',(0.00759391039005402,-0.853054096250918,
-0.87715542064339));
#36005=CARTESIAN_POINT('Ctrl Pts',(0.408468095313887,-0.748941101646617,
-0.86672145804091));
#36006=CARTESIAN_POINT('Ctrl Pts',(0.713062510398058,-0.468295649009072,
-0.856287495438429));
#36007=CARTESIAN_POINT('Ctrl Pts',(0.849581388698289,-0.077268509734015,
-0.845853532835948));
#36008=CARTESIAN_POINT('Ctrl Pts',(0.785845947261969,0.331971543645813,
-0.835419570233468));
#36009=CARTESIAN_POINT('Ctrl Pts',(0.536879228776822,0.662962783515193,
-0.824985607630987));
#36010=CARTESIAN_POINT('Ctrl Pts',(0.161365029180054,0.837687463184462,
-0.814551645028507));
#36011=CARTESIAN_POINT('Ctrl Pts',(-0.252184424692906,0.814961333169054,
-0.804117682426026));
#36012=CARTESIAN_POINT('Ctrl Pts',(-0.606291639027035,0.600141155949539,
-0.793683719823546));
#36013=CARTESIAN_POINT('Ctrl Pts',(-0.817490214648178,0.243862066695398,
-0.783249757221065));
#36014=CARTESIAN_POINT('Ctrl Pts',(-0.835998661927777,-0.169897604083914,
-0.772815794618584));
#36015=CARTESIAN_POINT('Ctrl Pts',(-0.657454365854886,-0.543610812472344,
-0.762381832016104));
#36016=CARTESIAN_POINT('Ctrl Pts',(-0.323941895404747,-0.789189842192653,
-0.751947869413623));
#36017=CARTESIAN_POINT('Ctrl Pts',(0.0859267249812216,-0.848749407394487,
-0.741513906811143));
#36018=CARTESIAN_POINT('Ctrl Pts',(0.475541608542061,-0.708250758675002,
-0.731079944208662));
#36019=CARTESIAN_POINT('Ctrl Pts',(0.753066864680076,-0.400810748283288,
-0.720645981606182));
#36020=CARTESIAN_POINT('Ctrl Pts',(0.853087181670373,0.00110412326700639,
-0.7102120190037));
#36021=CARTESIAN_POINT('Ctrl Pts',(0.752026830565643,0.402758742584047,
-0.69977805640122));
#36022=CARTESIAN_POINT('Ctrl Pts',(0.473706686130722,0.709479340173862,
-0.689344093798739));
#36023=CARTESIAN_POINT('Ctrl Pts',(0.0837294227343626,0.848968987882984,
-0.678910131196258));
#36024=CARTESIAN_POINT('Ctrl Pts',(-0.325983652691982,0.788348664485507,
-0.668476168593779));
#36025=CARTESIAN_POINT('Ctrl Pts',(-0.658859316796526,0.541907150062539,
-0.658042205991297));
#36026=CARTESIAN_POINT('Ctrl Pts',(-0.836435646379749,0.167733026216601,
-0.647608243388818));
#36027=CARTESIAN_POINT('Ctrl Pts',(-0.816856231267326,-0.245977348668995,
-0.637174280786336));
#36028=CARTESIAN_POINT('Ctrl Pts',(-0.604736123655922,-0.60170855018364,
-0.626740318183856));
#36029=CARTESIAN_POINT('Ctrl Pts',(-0.250074026927025,-0.815611390108666,
-0.616306355581375));
#36030=CARTESIAN_POINT('Ctrl Pts',(0.163532868748728,-0.83726695829783,
-0.605872392978895));
#36031=CARTESIAN_POINT('Ctrl Pts',(0.538593529983231,-0.661570833757573,
-0.595438430376414));
#36032=CARTESIAN_POINT('Ctrl Pts',(0.786702633196865,-0.329936244658886,
-0.585004467773934));
#36033=CARTESIAN_POINT('Ctrl Pts',(0.849378530433119,0.079467418844213,
-0.574570505171453));
#36034=CARTESIAN_POINT('Ctrl Pts',(0.711847923533838,0.470139864698849,
-0.564136542568972));
#36035=CARTESIAN_POINT('Ctrl Pts',(0.406528069390245,0.749995924933148,
-0.553702579966493));
#36036=CARTESIAN_POINT('Ctrl Pts',(0.00538572775796149,0.853070895386196,
-0.54326861736401));
#36037=CARTESIAN_POINT('Ctrl Pts',(-0.397026080534961,0.755069036574494,
-0.532834654761531));
#36038=CARTESIAN_POINT('Ctrl Pts',(-0.705855109435041,0.479090307878311,
-0.522400692159049));
#36039=CARTESIAN_POINT('Ctrl Pts',(-0.848307453708849,0.0901854899664934,
-0.51196672955657));
#36040=CARTESIAN_POINT('Ctrl Pts',(-0.7908057566996,-0.319976895711645,
-0.501532766954088));
#36041=CARTESIAN_POINT('Ctrl Pts',(-0.546903708932309,-0.654717719154274,
-0.491098804351608));
#36042=CARTESIAN_POINT('Ctrl Pts',(-0.174091315846699,-0.835135421572604,
-0.480664841749128));
#36043=CARTESIAN_POINT('Ctrl Pts',(0.23975603691495,-0.81870385450499,-0.470230879146647));
#36044=CARTESIAN_POINT('Ctrl Pts',(0.597090637969014,-0.609296092772836,
-0.459796916544167));
#36045=CARTESIAN_POINT('Ctrl Pts',(0.813685362752719,-0.256271514336748,
-0.449362953941686));
#36046=CARTESIAN_POINT('Ctrl Pts',(0.838486798553875,0.157158669087687,
-0.438928991339205));
#36047=CARTESIAN_POINT('Ctrl Pts',(0.665649013810144,0.533545076851013,
-0.428495028736725));
#36048=CARTESIAN_POINT('Ctrl Pts',(0.335911499133212,0.784169894454498,
-0.418061066134244));
#36049=CARTESIAN_POINT('Ctrl Pts',(-0.0730035135980338,0.849958496410589,
-0.407627103531763));
#36050=CARTESIAN_POINT('Ctrl Pts',(-0.464710911909924,0.715403890799101,
-0.397193140929283));
#36051=CARTESIAN_POINT('Ctrl Pts',(-0.746881579809863,0.412221863029791,
-0.386759178326802));
#36052=CARTESIAN_POINT('Ctrl Pts',(-0.853005238347077,0.0118752670898904,
-0.376325215724322));
#36053=CARTESIAN_POINT('Ctrl Pts',(-0.758067543607107,-0.391270440941414,
-0.36589125312184));
#36054=CARTESIAN_POINT('Ctrl Pts',(-0.484446202675582,-0.702190027925981,
-0.355457290519361));
#36055=CARTESIAN_POINT('Ctrl Pts',(-0.0966363378011864,-0.847596824471871,
-0.34502332791688));
#36056=CARTESIAN_POINT('Ctrl Pts',(0.313951620362249,-0.793217081681625,
-0.334589365314399));
#36057=CARTESIAN_POINT('Ctrl Pts',(0.650538230236913,-0.551868616254985,
-0.324155402711919));
#36058=CARTESIAN_POINT('Ctrl Pts',(0.833786864097282,-0.18043953001012,
-0.313721440109438));
#36059=CARTESIAN_POINT('Ctrl Pts',(0.820504095785434,0.233520849327348,
-0.303287477506957));
#36060=CARTESIAN_POINT('Ctrl Pts',(0.6138207997243,0.592438169948658,-0.292853514904477));
#36061=CARTESIAN_POINT('Ctrl Pts',(0.262454169604745,0.81171224344255,-0.282419552301996));
#36062=CARTESIAN_POINT('Ctrl Pts',(-0.150775372733257,0.839658113287939,
-0.271985589699516));
#36063=CARTESIAN_POINT('Ctrl Pts',(-0.528465747745009,0.669688667653643,
-0.261551627097035));
#36064=CARTESIAN_POINT('Ctrl Pts',(-0.781591767642338,0.341867317610364,
-0.251117664494554));
#36065=CARTESIAN_POINT('Ctrl Pts',(-0.850489281400512,-0.0665353923691048,
-0.240683701892074));
#36066=CARTESIAN_POINT('Ctrl Pts',(-0.718918435725105,-0.459255046614001,
-0.230249739289593));
#36067=CARTESIAN_POINT('Ctrl Pts',(-0.417891836923549,-0.743724044456582,
-0.219815776687113));
#36068=CARTESIAN_POINT('Ctrl Pts',(-0.0183640459380012,-0.852890145736156,
-0.209381814084632));
#36069=CARTESIAN_POINT('Ctrl Pts',(0.38549201298599,-0.761022313010097,
-0.198947851482151));
#36070=CARTESIAN_POINT('Ctrl Pts',(0.69848459067002,-0.489773795410256,
-0.188513888879671));
#36071=CARTESIAN_POINT('Ctrl Pts',(0.846836585170213,-0.103082114107123,
-0.17807992627719));
#36072=CARTESIAN_POINT('Ctrl Pts',(0.795583593099752,0.30790919991655,-0.16764596367471));
#36073=CARTESIAN_POINT('Ctrl Pts',(0.556799435517531,0.646319077797012,
-0.157212001072229));
#36074=CARTESIAN_POINT('Ctrl Pts',(0.186781528084318,0.832394012413366,
-0.146778038469748));
#36075=CARTESIAN_POINT('Ctrl Pts',(-0.227280478634909,0.822249052826763,
-0.136344075867268));
#36076=CARTESIAN_POINT('Ctrl Pts',(-0.58773477693239,0.61832545728428,-0.125910113264787));
#36077=CARTESIAN_POINT('Ctrl Pts',(-0.809727755002954,0.268589584372275,
-0.115476150662307));
#36078=CARTESIAN_POINT('Ctrl Pts',(-0.830358898319076,-0.00667087734730495,
-0.108520175593986));
#36079=CARTESIAN_POINT('Ctrl Pts',(-0.80768612908519,-0.138700154790167,
-0.105042188059826));
#36080=CARTESIAN_POINT('Ctrl Pts',(0.594875448103842,-0.571185894232435,
-1.13205842314276));
#36081=CARTESIAN_POINT('Ctrl Pts',(0.688244416305435,-0.47394451036991,
-1.1285804356086));
#36082=CARTESIAN_POINT('Ctrl Pts',(0.826319063393537,-0.232908375337079,
-1.12162446054028));
#36083=CARTESIAN_POINT('Ctrl Pts',(0.838590388344208,0.183775983334789,
-1.1111904979378));
#36084=CARTESIAN_POINT('Ctrl Pts',(0.653221937147487,0.557046083095301,
-1.10075653533532));
#36085=CARTESIAN_POINT('Ctrl Pts',(0.313871699922466,0.799062532067009,
-1.09032257273284));
#36086=CARTESIAN_POINT('Ctrl Pts',(-0.0994554132647963,0.852708501700446,
-1.07988861013036));
#36087=CARTESIAN_POINT('Ctrl Pts',(-0.489342809626885,0.705375220702387,
-1.06945464752788));
#36088=CARTESIAN_POINT('Ctrl Pts',(-0.763886051959438,0.391772185135781,
-1.0590206849254));
#36089=CARTESIAN_POINT('Ctrl Pts',(-0.858374910495864,-0.0141720913963306,
-1.04858672232292));
#36090=CARTESIAN_POINT('Ctrl Pts',(-0.750536357358176,-0.416777473112902,
-1.03815275972044));
#36091=CARTESIAN_POINT('Ctrl Pts',(-0.465789520808075,-0.721143672414928,
-1.02771879711796));
#36092=CARTESIAN_POINT('Ctrl Pts',(-0.0712516182342999,-0.855529943231549,
-1.01728483451548));
#36093=CARTESIAN_POINT('Ctrl Pts',(0.340080911027169,-0.788259553404189,
-1.006850871913));
#36094=CARTESIAN_POINT('Ctrl Pts',(0.67125319785122,-0.535189084049821,
-0.996416909310514));
#36095=CARTESIAN_POINT('Ctrl Pts',(0.844204783065118,-0.15596946206087,
-0.985982946708034));
#36096=CARTESIAN_POINT('Ctrl Pts',(0.81816937155348,0.260013600576988,-0.975548984105553));
#36097=CARTESIAN_POINT('Ctrl Pts',(0.599283744716542,0.614709027432676,
-0.965115021503073));
#36098=CARTESIAN_POINT('Ctrl Pts',(0.239141307420065,0.824511750823222,
-0.954681058900592));
#36099=CARTESIAN_POINT('Ctrl Pts',(-0.177368984921709,0.83996930744194,
-0.944247096298111));
#36100=CARTESIAN_POINT('Ctrl Pts',(-0.552071739738344,0.657438200377163,
-0.933813133695632));
#36101=CARTESIAN_POINT('Ctrl Pts',(-0.796645996016166,0.319942730235181,
-0.923379171093149));
#36102=CARTESIAN_POINT('Ctrl Pts',(-0.853443302115344,-0.092966249499067,
-0.91294520849067));
#36103=CARTESIAN_POINT('Ctrl Pts',(-0.709075999240419,-0.483962210060312,
-0.902511245888189));
#36104=CARTESIAN_POINT('Ctrl Pts',(-0.397572817705147,-0.760883728388119,
-0.892077283285709));
#36105=CARTESIAN_POINT('Ctrl Pts',(0.00764201429866176,-0.858457799247161,
-0.881643320683228));
#36106=CARTESIAN_POINT('Ctrl Pts',(0.411055551701723,-0.753685296994473,
-0.871209358080748));
#36107=CARTESIAN_POINT('Ctrl Pts',(0.717579431471206,-0.471262085267668,
-0.860775395478267));
#36108=CARTESIAN_POINT('Ctrl Pts',(0.854963093698934,-0.0777579699914457,
-0.850341432875786));
#36109=CARTESIAN_POINT('Ctrl Pts',(0.790823917731152,0.334074429773347,
-0.839907470273306));
#36110=CARTESIAN_POINT('Ctrl Pts',(0.540280110279977,0.667162345999428,
-0.829473507670825));
#36111=CARTESIAN_POINT('Ctrl Pts',(0.162387201977173,0.842993825670225,
-0.819039545068344));
#36112=CARTESIAN_POINT('Ctrl Pts',(-0.25378189633895,0.820123736136429,
-0.808605582465865));
#36113=CARTESIAN_POINT('Ctrl Pts',(-0.610132216032373,0.603942772490375,
-0.798171619863382));
#36114=CARTESIAN_POINT('Ctrl Pts',(-0.822668636909623,0.245406820054239,
-0.787737657260903));
#36115=CARTESIAN_POINT('Ctrl Pts',(-0.841294326638979,-0.170973826795073,
-0.777303694658422));
#36116=CARTESIAN_POINT('Ctrl Pts',(-0.661619035061958,-0.547054335443541,
-0.766869732055942));
#36117=CARTESIAN_POINT('Ctrl Pts',(-0.325993917425953,-0.794188994689024,
-0.75643576945346));
#36118=CARTESIAN_POINT('Ctrl Pts',(0.0864710310261411,-0.854125842178518,
-0.746001806850982));
#36119=CARTESIAN_POINT('Ctrl Pts',(0.478553944601616,-0.71273719952737,
-0.735567844248499));
#36120=CARTESIAN_POINT('Ctrl Pts',(0.757837194827813,-0.403349698920672,
-0.72513388164602));
#36121=CARTESIAN_POINT('Ctrl Pts',(0.858491094247378,0.00111111737703042,
-0.714699919043537));
#36122=CARTESIAN_POINT('Ctrl Pts',(0.756790572578483,0.405310032864,-0.704265956441059));
#36123=CARTESIAN_POINT('Ctrl Pts',(0.476707398805809,0.713973563521567,
-0.693831993838577));
#36124=CARTESIAN_POINT('Ctrl Pts',(0.0842598098862286,0.854346813607812,
-0.683398031236096));
#36125=CARTESIAN_POINT('Ctrl Pts',(-0.328048608300893,0.793342488510311,
-0.672964068633616));
#36126=CARTESIAN_POINT('Ctrl Pts',(-0.663032885717749,0.545339881120644,
-0.662530106031135));
#36127=CARTESIAN_POINT('Ctrl Pts',(-0.841734079185264,0.168795537328509,
-0.652096143428655));
#36128=CARTESIAN_POINT('Ctrl Pts',(-0.822030637537394,-0.24753550136041,
-0.641662180826173));
#36129=CARTESIAN_POINT('Ctrl Pts',(-0.608566847191112,-0.605520095441724,
-0.631228218223695));
#36130=CARTESIAN_POINT('Ctrl Pts',(-0.251658130179693,-0.820777910885976,
-0.620794255621212));
#36131=CARTESIAN_POINT('Ctrl Pts',(0.164568773806467,-0.842570657079702,
-0.610360293018733));
#36132=CARTESIAN_POINT('Ctrl Pts',(0.542005270791329,-0.66576157888414,
-0.599926330416251));
#36133=CARTESIAN_POINT('Ctrl Pts',(0.791686030375065,-0.332026238109064,
-0.589492367813771));
#36134=CARTESIAN_POINT('Ctrl Pts',(0.85475895042051,0.0799708081734412,
-0.57905840521129));
#36135=CARTESIAN_POINT('Ctrl Pts',(0.716357150761197,0.473117983210515,
-0.56862444260881));
#36136=CARTESIAN_POINT('Ctrl Pts',(0.409103236611468,0.754746802098496,
-0.558190480006329));
#36137=CARTESIAN_POINT('Ctrl Pts',(0.00541984385136099,0.858474704797125,
-0.547756517403849));
#36138=CARTESIAN_POINT('Ctrl Pts',(-0.399541057053306,0.759852049554789,
-0.537322554801367));
#36139=CARTESIAN_POINT('Ctrl Pts',(-0.710326374957927,0.482125123306196,
-0.526888592198888));
#36140=CARTESIAN_POINT('Ctrl Pts',(-0.853681088920773,0.0907567733170878,
-0.516454629596407));
#36141=CARTESIAN_POINT('Ctrl Pts',(-0.795815145266696,-0.32200380129438,
-0.506020666993927));
#36142=CARTESIAN_POINT('Ctrl Pts',(-0.550368090878974,-0.658865052970729,
-0.495586704391446));
#36143=CARTESIAN_POINT('Ctrl Pts',(-0.175194103781467,-0.840425618055572,
-0.485152741788965));
#36144=CARTESIAN_POINT('Ctrl Pts',(0.24127478047497,-0.823889964613384,
-0.474718779186485));
#36145=CARTESIAN_POINT('Ctrl Pts',(0.600872930889902,-0.613155701602509,
-0.464284816584004));
#36146=CARTESIAN_POINT('Ctrl Pts',(0.818839683037892,-0.257894875804611,
-0.453850853981523));
#36147=CARTESIAN_POINT('Ctrl Pts',(0.843798224459356,0.158154196539881,
-0.443416891379043));
#36148=CARTESIAN_POINT('Ctrl Pts',(0.669865592320392,0.536924838044412,
-0.432982928776562));
#36149=CARTESIAN_POINT('Ctrl Pts',(0.338039343055767,0.789137247904648,
-0.422548966174082));
#36150=CARTESIAN_POINT('Ctrl Pts',(-0.0734659570783422,0.855342590214103,
-0.412115003571601));
#36151=CARTESIAN_POINT('Ctrl Pts',(-0.467654640517619,0.719935643433753,
-0.40168104096912));
#36152=CARTESIAN_POINT('Ctrl Pts',(-0.751612729039847,0.414833097799243,
-0.39124707836664));
#36153=CARTESIAN_POINT('Ctrl Pts',(-0.85840863185104,0.0119504914122616,
-0.380813115764159));
#36154=CARTESIAN_POINT('Ctrl Pts',(-0.762869550742065,-0.393748958145996,
-0.370379153161678));
#36155=CARTESIAN_POINT('Ctrl Pts',(-0.487514945218855,-0.7066380768534,
-0.359945190559198));
#36156=CARTESIAN_POINT('Ctrl Pts',(-0.0972484842880587,-0.852965958176227,
-0.349511227956717));
#36157=CARTESIAN_POINT('Ctrl Pts',(0.315940358613543,-0.798241744877081,
-0.339077265354237));
#36158=CARTESIAN_POINT('Ctrl Pts',(0.654659088924836,-0.555364448591704,
-0.328643302751756));
#36159=CARTESIAN_POINT('Ctrl Pts',(0.839068518092747,-0.181582530945507,
-0.318209340149276));
#36160=CARTESIAN_POINT('Ctrl Pts',(0.825701609589118,0.235000095861305,
-0.307775377546795));
#36161=CARTESIAN_POINT('Ctrl Pts',(0.617709070479461,0.596190991632757,
-0.297341414944314));
#36162=CARTESIAN_POINT('Ctrl Pts',(0.26411669533205,0.816854064938793,-0.286907452341834));
#36163=CARTESIAN_POINT('Ctrl Pts',(-0.151730464954597,0.844976958912708,
-0.276473489739353));
#36164=CARTESIAN_POINT('Ctrl Pts',(-0.531813333742563,0.673930835536443,
-0.266039527136873));
#36165=CARTESIAN_POINT('Ctrl Pts',(-0.786542789844422,0.344032888819272,
-0.255605564534392));
#36166=CARTESIAN_POINT('Ctrl Pts',(-0.855876737496278,-0.0669568631605737,
-0.245171601931911));
#36167=CARTESIAN_POINT('Ctrl Pts',(-0.723472451346347,-0.462164215102107,
-0.234737639329431));
#36168=CARTESIAN_POINT('Ctrl Pts',(-0.420538988411856,-0.748435191644753,
-0.22430367672695));
#36169=CARTESIAN_POINT('Ctrl Pts',(-0.0184803735586201,-0.858292811196644,
-0.21386971412447));
#36170=CARTESIAN_POINT('Ctrl Pts',(0.387933926300145,-0.765843035246914,
-0.203435751521989));
#36171=CARTESIAN_POINT('Ctrl Pts',(0.702909167805226,-0.492876289710407,
-0.193001788919508));
#36172=CARTESIAN_POINT('Ctrl Pts',(0.852200902248733,-0.103735083894904,
-0.182567826317028));
#36173=CARTESIAN_POINT('Ctrl Pts',(0.80062324874381,0.309859647074902,-0.172133863714547));
#36174=CARTESIAN_POINT('Ctrl Pts',(0.560326498983091,0.650413239900023,
-0.161699901112067));
#36175=CARTESIAN_POINT('Ctrl Pts',(0.18796470919147,0.837666784744461,-0.151265938509586));
#36176=CARTESIAN_POINT('Ctrl Pts',(-0.228720208214088,0.827457735607709,
-0.140831975907105));
#36177=CARTESIAN_POINT('Ctrl Pts',(-0.591457779048169,0.622242032554347,
-0.130398013304625));
#36178=CARTESIAN_POINT('Ctrl Pts',(-0.814857060568082,0.270291466147333,
-0.119964050702144));
#36179=CARTESIAN_POINT('Ctrl Pts',(-0.83561875211749,-0.00671391055874626,
-0.113008075633824));
#36180=CARTESIAN_POINT('Ctrl Pts',(-0.812802493323686,-0.139578764049739,
-0.109530088099664));
#36181=CARTESIAN_POINT('Ctrl Pts',(0.596426278379634,-0.572674966240204,
-1.13871522674109));
#36182=CARTESIAN_POINT('Ctrl Pts',(0.690040836764293,-0.475177806505627,
-1.13523723920693));
#36183=CARTESIAN_POINT('Ctrl Pts',(0.828472169960178,-0.233517118585332,
-1.12828126413861));
#36184=CARTESIAN_POINT('Ctrl Pts',(0.840777371648047,0.184255830864911,
-1.11784730153613));
#36185=CARTESIAN_POINT('Ctrl Pts',(0.65492472312175,0.558498066470781,-1.10741333893365));
#36186=CARTESIAN_POINT('Ctrl Pts',(0.314690182553937,0.80114603583872,-1.09697937633117));
#36187=CARTESIAN_POINT('Ctrl Pts',(-0.099714792256329,0.854931601464745,
-1.08654541372869));
#36188=CARTESIAN_POINT('Ctrl Pts',(-0.490618589981855,0.70721432902319,
-1.07611145112621));
#36189=CARTESIAN_POINT('Ctrl Pts',(-0.765877684119506,0.392793594264123,
-1.06567748852373));
#36190=CARTESIAN_POINT('Ctrl Pts',(-0.860612864682261,-0.0142090290307453,
-1.05524352592124));
#36191=CARTESIAN_POINT('Ctrl Pts',(-0.752493169135755,-0.417864105986004,
-1.04480956331877));
#36192=CARTESIAN_POINT('Ctrl Pts',(-0.467003929674384,-0.723023842952487,
-1.03437560071628));
#36193=CARTESIAN_POINT('Ctrl Pts',(-0.0714373875773892,-0.857760491803007,
-1.02394163811381));
#36194=CARTESIAN_POINT('Ctrl Pts',(0.340967574370296,-0.790314711499318,
-1.01350767551132));
#36195=CARTESIAN_POINT('Ctrl Pts',(0.673003296155675,-0.536584435271303,
-1.00307371290884));
#36196=CARTESIAN_POINT('Ctrl Pts',(0.846405803153589,-0.156376107134283,
-0.992639750306363));
#36197=CARTESIAN_POINT('Ctrl Pts',(0.820302511565667,0.260691510764428,
-0.982205787703882));
#36198=CARTESIAN_POINT('Ctrl Pts',(0.600846203873041,0.616311703562287,
-0.971771825101402));
#36199=CARTESIAN_POINT('Ctrl Pts',(0.239764799219726,0.826661426818636,
-0.96133786249892));
#36200=CARTESIAN_POINT('Ctrl Pts',(-0.177831423260395,0.842159284588733,
-0.950903899896441));
#36201=CARTESIAN_POINT('Ctrl Pts',(-0.553511107201052,0.659152280411272,
-0.94046993729396));
#36202=CARTESIAN_POINT('Ctrl Pts',(-0.798723020136248,0.320776888411988,
-0.930035974691479));
#36203=CARTESIAN_POINT('Ctrl Pts',(-0.855668408795536,-0.0932086321197977,
-0.919602012088999));
#36204=CARTESIAN_POINT('Ctrl Pts',(-0.710924709912794,-0.485224001607969,
-0.909168049486518));
#36205=CARTESIAN_POINT('Ctrl Pts',(-0.398609373888867,-0.762867512737829,
-0.898734086884038));
#36206=CARTESIAN_POINT('Ctrl Pts',(0.0076619386418344,-0.860695979777121,
-0.888300124281556));
#36207=CARTESIAN_POINT('Ctrl Pts',(0.412127260215954,-0.75565031351505,
-0.877866161679076));
#36208=CARTESIAN_POINT('Ctrl Pts',(0.719450312385616,-0.472490764912421,
-0.867432199076595));
#36209=CARTESIAN_POINT('Ctrl Pts',(0.857192162794716,-0.0779607014182942,
-0.856998236474115));
#36210=CARTESIAN_POINT('Ctrl Pts',(0.792885762468364,0.334945432267619,
-0.846564273871634));
#36211=CARTESIAN_POINT('Ctrl Pts',(0.5416887344718,0.668901778939058,-0.836130311269154));
#36212=CARTESIAN_POINT('Ctrl Pts',(0.162810579659967,0.845191688359987,
-0.825696348666673));
#36213=CARTESIAN_POINT('Ctrl Pts',(-0.254443559264959,0.822261971679498,
-0.815262386064192));
#36214=CARTESIAN_POINT('Ctrl Pts',(-0.611722959395611,0.605517378668957,
-0.804828423461712));
#36215=CARTESIAN_POINT('Ctrl Pts',(-0.824813507545726,0.246046647390079,
-0.794394460859231));
#36216=CARTESIAN_POINT('Ctrl Pts',(-0.84348775837634,-0.171419591619671,
-0.783960498256751));
#36217=CARTESIAN_POINT('Ctrl Pts',(-0.663344015420905,-0.548480621469046,
-0.77352653565427));
#36218=CARTESIAN_POINT('Ctrl Pts',(-0.32684385232035,-0.796259612891541,
-0.76309257305179));
#36219=CARTESIAN_POINT('Ctrl Pts',(0.0866964792406478,-0.856352728383039,
-0.752658610449309));
#36220=CARTESIAN_POINT('Ctrl Pts',(0.479801635661559,-0.714595455721829,
-0.742224647846828));
#36221=CARTESIAN_POINT('Ctrl Pts',(0.759813036221548,-0.404401316651654,
-0.731790685244348));
#36222=CARTESIAN_POINT('Ctrl Pts',(0.860729361584667,0.00111401429436622,
-0.721356722641867));
#36223=CARTESIAN_POINT('Ctrl Pts',(0.758763685207283,0.406366761599003,
-0.710922760039386));
#36224=CARTESIAN_POINT('Ctrl Pts',(0.477950275531429,0.715835043177707,
-0.700488797436906));
#36225=CARTESIAN_POINT('Ctrl Pts',(0.0844794929808797,0.856574275931452,
-0.690054834834425));
#36226=CARTESIAN_POINT('Ctrl Pts',(-0.328903900207732,0.795410899692694,
-0.679620872231945));
#36227=CARTESIAN_POINT('Ctrl Pts',(-0.664761552283536,0.546761697202154,
-0.669186909629464));
#36228=CARTESIAN_POINT('Ctrl Pts',(-0.843928657450255,0.16923562289307,
-0.658752947026984));
#36229=CARTESIAN_POINT('Ctrl Pts',(-0.824173844774582,-0.248180878617352,
-0.648318984424503));
#36230=CARTESIAN_POINT('Ctrl Pts',(-0.610153509307647,-0.607098814033894,
-0.637885021822023));
#36231=CARTESIAN_POINT('Ctrl Pts',(-0.252314255999424,-0.822917852000584,
-0.627451059219541));
#36232=CARTESIAN_POINT('Ctrl Pts',(0.164997839307108,-0.844767416479698,
-0.617017096617062));
#36233=CARTESIAN_POINT('Ctrl Pts',(0.543418392840446,-0.667497359728489,
-0.606583134014579));
#36234=CARTESIAN_POINT('Ctrl Pts',(0.793750122821744,-0.33289190053569,
-0.596149171412101));
#36235=CARTESIAN_POINT('Ctrl Pts',(0.856987487271739,0.0801793089360827,
-0.585715208809619));
#36236=CARTESIAN_POINT('Ctrl Pts',(0.718224844931966,0.474351501572674,
-0.575281246207139));
#36237=CARTESIAN_POINT('Ctrl Pts',(0.410169855028622,0.756714586186626,
-0.564847283604658));
#36238=CARTESIAN_POINT('Ctrl Pts',(0.00543397452731906,0.860712929403663,
-0.554413321002177));
#36239=CARTESIAN_POINT('Ctrl Pts',(-0.400582744851701,0.761833144099726,
-0.543979358399697));
#36240=CARTESIAN_POINT('Ctrl Pts',(-0.712178345624295,0.483382125182179,
-0.533545395797217));
#36241=CARTESIAN_POINT('Ctrl Pts',(-0.855906815559753,0.090993395365603,
-0.523111433194736));
#36242=CARTESIAN_POINT('Ctrl Pts',(-0.797890003186722,-0.322843333114511,
-0.512677470592255));
#36243=CARTESIAN_POINT('Ctrl Pts',(-0.551803016563766,-0.660582853117555,
-0.502243507989775));
#36244=CARTESIAN_POINT('Ctrl Pts',(-0.175650871758219,-0.842616784886445,
-0.491809545387294));
#36245=CARTESIAN_POINT('Ctrl Pts',(0.241903834712186,-0.826038019508388,
-0.481375582784813));
#36246=CARTESIAN_POINT('Ctrl Pts',(0.602439533344005,-0.614754327830277,
-0.470941620182333));
#36247=CARTESIAN_POINT('Ctrl Pts',(0.82097457078373,-0.258567262135508,
-0.460507657579852));
#36248=CARTESIAN_POINT('Ctrl Pts',(0.845998184386402,0.158566537884764,
-0.450073694977372));
#36249=CARTESIAN_POINT('Ctrl Pts',(0.671612073193301,0.538324714333898,
-0.439639732374891));
#36250=CARTESIAN_POINT('Ctrl Pts',(0.338920682915143,0.791194695137898,
-0.429205769772411));
#36251=CARTESIAN_POINT('Ctrl Pts',(-0.0736574983223131,0.857572648737351,
-0.41877180716993));
#36252=CARTESIAN_POINT('Ctrl Pts',(-0.468873914793169,0.72181266748964,
-0.408337844567449));
#36253=CARTESIAN_POINT('Ctrl Pts',(-0.753572341938536,0.415914655172892,
-0.397903881964968));
#36254=CARTESIAN_POINT('Ctrl Pts',(-0.86064668419148,0.0119816488637972,
-0.387469919362488));
#36255=CARTESIAN_POINT('Ctrl Pts',(-0.764858512548967,-0.394775544721155,
-0.377035956760007));
#36256=CARTESIAN_POINT('Ctrl Pts',(-0.488785999497305,-0.708480431348438,
-0.366601994157526));
#36257=CARTESIAN_POINT('Ctrl Pts',(-0.0975020315960993,-0.855189820319156,
-0.356168031555046));
#36258=CARTESIAN_POINT('Ctrl Pts',(0.316764081759698,-0.800322929452839,
-0.345734068952565));
#36259=CARTESIAN_POINT('Ctrl Pts',(0.656365923236629,-0.556812400837173,
-0.335300106350085));
#36260=CARTESIAN_POINT('Ctrl Pts',(0.841256146677281,-0.182055954894479,
-0.324866143747604));
#36261=CARTESIAN_POINT('Ctrl Pts',(0.827854387825681,0.235612790663157,
-0.314432181145124));
#36262=CARTESIAN_POINT('Ctrl Pts',(0.619319568298158,0.597745387301993,
-0.303998218542643));
#36263=CARTESIAN_POINT('Ctrl Pts',(0.264805303262624,0.818983775723723,
-0.293564255940162));
#36264=CARTESIAN_POINT('Ctrl Pts',(-0.152126058284336,0.847179992119362,
-0.283130293337682));
#36265=CARTESIAN_POINT('Ctrl Pts',(-0.533199883246883,0.67568791521759,
-0.272696330735201));
#36266=CARTESIAN_POINT('Ctrl Pts',(-0.788593472808696,0.34492985538811,
-0.262262368132721));
#36267=CARTESIAN_POINT('Ctrl Pts',(-0.85810818859447,-0.0671314343578877,
-0.25182840553024));
#36268=CARTESIAN_POINT('Ctrl Pts',(-0.725358696723672,-0.463369173631078,
-0.241394442927759));
#36269=CARTESIAN_POINT('Ctrl Pts',(-0.42163542201511,-0.750386522096553,
-0.230960480325279));
#36270=CARTESIAN_POINT('Ctrl Pts',(-0.0185285562433286,-0.86053055751242,
-0.220526517722798));
#36271=CARTESIAN_POINT('Ctrl Pts',(0.388945352751919,-0.767839757527661,
-0.210092555120318));
#36272=CARTESIAN_POINT('Ctrl Pts',(0.704741798496438,-0.494161306472502,
-0.199658592517837));
#36273=CARTESIAN_POINT('Ctrl Pts',(0.854422773172538,-0.104005573943587,
-0.189224629915357));
#36274=CARTESIAN_POINT('Ctrl Pts',(0.802710635634209,0.310667577083977,
-0.178790667312876));
#36275=CARTESIAN_POINT('Ctrl Pts',(0.561787401646006,0.652108885332522,
-0.168356704710395));
#36276=CARTESIAN_POINT('Ctrl Pts',(0.188454746657786,0.839850992854134,
-0.157922742107915));
#36277=CARTESIAN_POINT('Ctrl Pts',(-0.229316478451291,0.829614630969344,
-0.147488779505434));
#36278=CARTESIAN_POINT('Ctrl Pts',(-0.592999937130289,0.623865269466565,
-0.137054816902953));
#36279=CARTESIAN_POINT('Ctrl Pts',(-0.816981345420958,0.270994210833155,
-0.126620854300473));
#36280=CARTESIAN_POINT('Ctrl Pts',(-0.837797728572329,-0.00672831308054614,
-0.119664879232153));
#36281=CARTESIAN_POINT('Ctrl Pts',(-0.81492145573658,-0.139942643537178,
-0.116186891697992));
#36282=CARTESIAN_POINT('Ctrl Pts',(0.596426278379634,-0.572674966240204,
-1.1425283350431));
#36283=CARTESIAN_POINT('Ctrl Pts',(0.690039237300988,-0.475179472305605,
-1.13905034750894));
#36284=CARTESIAN_POINT('Ctrl Pts',(0.82847297254682,-0.233515977058047,
-1.13209437244062));
#36285=CARTESIAN_POINT('Ctrl Pts',(0.840776790045668,0.184255282770994,
-1.12166040983814));
#36286=CARTESIAN_POINT('Ctrl Pts',(0.654924835154705,0.558498232654801,
-1.11122644723566));
#36287=CARTESIAN_POINT('Ctrl Pts',(0.314690017828941,0.801145770682765,
-1.10079248463318));
#36288=CARTESIAN_POINT('Ctrl Pts',(-0.0997147185513843,0.854931525810343,
-1.0903585220307));
#36289=CARTESIAN_POINT('Ctrl Pts',(-0.490618537208122,0.707214177068773,
-1.07992455942821));
#36290=CARTESIAN_POINT('Ctrl Pts',(-0.765877541643972,0.392793546079606,
-1.06949059682574));
#36291=CARTESIAN_POINT('Ctrl Pts',(-0.860612728693631,-0.0142090354680799,
-1.05905663422325));
#36292=CARTESIAN_POINT('Ctrl Pts',(-0.752493039839578,-0.417864031829528,
-1.04862267162077));
#36293=CARTESIAN_POINT('Ctrl Pts',(-0.467003853748614,-0.723023724671487,
-1.03818870901829));
#36294=CARTESIAN_POINT('Ctrl Pts',(-0.0714373746764496,-0.857760347616997,
-1.02775474641581));
#36295=CARTESIAN_POINT('Ctrl Pts',(0.340967517012713,-0.790314580308689,
-1.01732078381333));
#36296=CARTESIAN_POINT('Ctrl Pts',(0.673003184192239,-0.536584345498902,
-1.00688682121085));
#36297=CARTESIAN_POINT('Ctrl Pts',(0.846405661890073,-0.156376081212101,
-0.996452858608372));
#36298=CARTESIAN_POINT('Ctrl Pts',(0.820302374851196,0.260691467373266,
-0.986018896005888));
#36299=CARTESIAN_POINT('Ctrl Pts',(0.600846103651696,0.616311600756361,
-0.97558493340341));
#36300=CARTESIAN_POINT('Ctrl Pts',(0.239764759257472,0.826661288997698,
-0.965150970800928));
#36301=CARTESIAN_POINT('Ctrl Pts',(-0.17783139361675,0.842159144153302,
-0.954717008198448));
#36302=CARTESIAN_POINT('Ctrl Pts',(-0.553511014901828,0.659152170506626,
-0.944283045595968));
#36303=CARTESIAN_POINT('Ctrl Pts',(-0.798722886956041,0.320776834921644,
-0.933849082993486));
#36304=CARTESIAN_POINT('Ctrl Pts',(-0.855668266116611,-0.0932086165764496,
-0.923415120391006));
#36305=CARTESIAN_POINT('Ctrl Pts',(-0.710924591370777,-0.485223920700346,
-0.912981157788526));
#36306=CARTESIAN_POINT('Ctrl Pts',(-0.398609307422754,-0.762867385533718,
-0.902547195186045));
#36307=CARTESIAN_POINT('Ctrl Pts',(0.00766193736409961,-0.860695836261202,
-0.892113232583564));
#36308=CARTESIAN_POINT('Ctrl Pts',(0.412127191496183,-0.755650187514622,
-0.881679269981084));
#36309=CARTESIAN_POINT('Ctrl Pts',(0.719450192421382,-0.472490686127355,
-0.871245307378603));
#36310=CARTESIAN_POINT('Ctrl Pts',(0.857192019862882,-0.0779606884187723,
-0.860811344776123));
#36311=CARTESIAN_POINT('Ctrl Pts',(0.79288563025922,0.334945376417385,-0.850377382173642));
#36312=CARTESIAN_POINT('Ctrl Pts',(0.541688644148329,0.668901667403547,
-0.839943419571162));
#36313=CARTESIAN_POINT('Ctrl Pts',(0.162810552512238,0.845191547429138,
-0.829509456968681));
#36314=CARTESIAN_POINT('Ctrl Pts',(-0.25444351683796,0.822261834572052,
-0.8190754943662));
#36315=CARTESIAN_POINT('Ctrl Pts',(-0.611722857394332,0.605517277702421,
-0.80864153176372));
#36316=CARTESIAN_POINT('Ctrl Pts',(-0.824813370012825,0.246046606363219,
-0.798207569161239));
#36317=CARTESIAN_POINT('Ctrl Pts',(-0.843487617729615,-0.171419563036442,
-0.787773606558759));
#36318=CARTESIAN_POINT('Ctrl Pts',(-0.663343904812112,-0.548480530013062,
-0.777339643956278));
#36319=CARTESIAN_POINT('Ctrl Pts',(-0.32684379782102,-0.796259480119838,
-0.766905681353796));
#36320=CARTESIAN_POINT('Ctrl Pts',(0.0866964647845089,-0.856352585591155,
-0.756471718751317));
#36321=CARTESIAN_POINT('Ctrl Pts',(0.479801555657401,-0.714595336567153,
-0.746037756148836));
#36322=CARTESIAN_POINT('Ctrl Pts',(0.7598129095271,-0.404401249220064,-0.735603793546356));
#36323=CARTESIAN_POINT('Ctrl Pts',(0.860729218063005,0.00111401410861053,
-0.725169830943874));
#36324=CARTESIAN_POINT('Ctrl Pts',(0.758763558687808,0.406366693839686,
-0.714735868341394));
#36325=CARTESIAN_POINT('Ctrl Pts',(0.477950195835974,0.715834923816337,
-0.704301905738913));
#36326=CARTESIAN_POINT('Ctrl Pts',(0.0844794788944107,0.856574133102626,
-0.693867943136432));
#36327=CARTESIAN_POINT('Ctrl Pts',(-0.328903845364902,0.795410767062507,
-0.683433980533953));
#36328=CARTESIAN_POINT('Ctrl Pts',(-0.664761441438376,0.546761606032791,
-0.673000017931471));
#36329=CARTESIAN_POINT('Ctrl Pts',(-0.843928516730013,0.169235594674005,
-0.662566055328991));
#36330=CARTESIAN_POINT('Ctrl Pts',(-0.82417370734834,-0.24818083723462,
-0.652132092726511));
#36331=CARTESIAN_POINT('Ctrl Pts',(-0.610153407568064,-0.607098712803663,
-0.64169813012403));
#36332=CARTESIAN_POINT('Ctrl Pts',(-0.252314213927475,-0.822917714783773,
-0.63126416752155));
#36333=CARTESIAN_POINT('Ctrl Pts',(0.164997811794668,-0.844767275619597,
-0.620830204919068));
#36334=CARTESIAN_POINT('Ctrl Pts',(0.543418302228559,-0.66749724842715,
-0.610396242316588));
#36335=CARTESIAN_POINT('Ctrl Pts',(0.793749990468483,-0.332891845027883,
-0.599962279714107));
#36336=CARTESIAN_POINT('Ctrl Pts',(0.856987344374013,0.0801792955666445,
-0.589528317111627));
#36337=CARTESIAN_POINT('Ctrl Pts',(0.71822472517211,0.474351422477294,-0.579094354509146));
#36338=CARTESIAN_POINT('Ctrl Pts',(0.410169786635162,0.756714460008827,
-0.568660391906666));
#36339=CARTESIAN_POINT('Ctrl Pts',(0.00543397362123471,0.86071278588474,
-0.558226429304185));
#36340=CARTESIAN_POINT('Ctrl Pts',(-0.400582678056836,0.761833017068438,
-0.547792466701704));
#36341=CARTESIAN_POINT('Ctrl Pts',(-0.712178226872659,0.483382044580994,
-0.537358504099224));
#36342=CARTESIAN_POINT('Ctrl Pts',(-0.855906672842221,0.0909933801929788,
-0.526924541496743));
#36343=CARTESIAN_POINT('Ctrl Pts',(-0.797889870143161,-0.322843279282246,
-0.516490578894263));
#36344=CARTESIAN_POINT('Ctrl Pts',(-0.551802924553791,-0.660582742969169,
-0.506056616291782));
#36345=CARTESIAN_POINT('Ctrl Pts',(-0.175650842469449,-0.842616644384951,
-0.495622653689302));
#36346=CARTESIAN_POINT('Ctrl Pts',(0.241903794376115,-0.826037881771306,
-0.485188691086821));
#36347=CARTESIAN_POINT('Ctrl Pts',(0.602439432890683,-0.614754225323535,
-0.47475472848434));
#36348=CARTESIAN_POINT('Ctrl Pts',(0.82097443389095,-0.258567219020906,
-0.46432076588186));
#36349=CARTESIAN_POINT('Ctrl Pts',(0.845998043321078,0.158566511444706,
-0.453886803279379));
#36350=CARTESIAN_POINT('Ctrl Pts',(0.671611961205856,0.538324624571355,
-0.443452840676899));
#36351=CARTESIAN_POINT('Ctrl Pts',(0.338920626402072,0.791194563210736,
-0.433018878074418));
#36352=CARTESIAN_POINT('Ctrl Pts',(-0.0736574860403502,0.85757250574206,
-0.422584915471937));
#36353=CARTESIAN_POINT('Ctrl Pts',(-0.468873836611143,0.72181254713152,
-0.412150952869456));
#36354=CARTESIAN_POINT('Ctrl Pts',(-0.753572216284692,0.41591458582155,
-0.401716990266976));
#36355=CARTESIAN_POINT('Ctrl Pts',(-0.860646540683597,0.0119816468658661,
-0.391283027664495));
#36356=CARTESIAN_POINT('Ctrl Pts',(-0.764858385013229,-0.394775478894489,
-0.380849065062015));
#36357=CARTESIAN_POINT('Ctrl Pts',(-0.48878591799503,-0.708480313213638,
-0.370415102459534));
#36358=CARTESIAN_POINT('Ctrl Pts',(-0.0975020153382475,-0.855189677720724,
-0.359981139857053));
#36359=CARTESIAN_POINT('Ctrl Pts',(0.316764028941211,-0.800322796004496,
-0.349547177254573));
#36360=CARTESIAN_POINT('Ctrl Pts',(0.656365813791197,-0.556812307990154,
-0.339113214652092));
#36361=CARTESIAN_POINT('Ctrl Pts',(0.84125600640305,-0.182055924541153,
-0.328679252049612));
#36362=CARTESIAN_POINT('Ctrl Pts',(0.827854249784972,0.235612751382874,
-0.318245289447131));
#36363=CARTESIAN_POINT('Ctrl Pts',(0.61931946503168,0.597745287618039,-0.307811326844651));
#36364=CARTESIAN_POINT('Ctrl Pts',(0.264805259104931,0.818983639189147,
-0.29737736424217));
#36365=CARTESIAN_POINT('Ctrl Pts',(-0.152126032912425,0.847179850805378,
-0.286943401639689));
#36366=CARTESIAN_POINT('Ctrl Pts',(-0.533199794350212,0.675687802651956,
-0.276509439037209));
#36367=CARTESIAN_POINT('Ctrl Pts',(-0.78859334129299,0.344929797673649,
-0.266075476434728));
#36368=CARTESIAN_POINT('Ctrl Pts',(-0.858108045553686,-0.067131422772148,
-0.255641513832248));
#36369=CARTESIAN_POINT('Ctrl Pts',(-0.725358575688162,-0.463369097137429,
-0.245207551229767));
#36370=CARTESIAN_POINT('Ctrl Pts',(-0.421635351879133,-0.750386395459336,
-0.234773588627287));
#36371=CARTESIAN_POINT('Ctrl Pts',(-0.0185285528209972,-0.860530417001192,
-0.224339626024805));
#36372=CARTESIAN_POINT('Ctrl Pts',(0.388945287243321,-0.767839623642233,
-0.213905663422325));
#36373=CARTESIAN_POINT('Ctrl Pts',(0.704741682270793,-0.494161235578596,
-0.203471700819845));
#36374=CARTESIAN_POINT('Ctrl Pts',(0.854422628174535,-0.104005533986048,
-0.193037738217364));
#36375=CARTESIAN_POINT('Ctrl Pts',(0.802710506756154,0.310667480825686,
-0.182603775614883));
#36376=CARTESIAN_POINT('Ctrl Pts',(0.561787298202017,0.652108863993629,
-0.172169813012403));
#36377=CARTESIAN_POINT('Ctrl Pts',(0.188454734446523,0.839850680936053,
-0.161735850409922));
#36378=CARTESIAN_POINT('Ctrl Pts',(-0.229316478079899,0.829614831389836,
-0.151301887807442));
#36379=CARTESIAN_POINT('Ctrl Pts',(-0.592999762703061,0.623864489566949,
-0.140867925204961));
#36380=CARTESIAN_POINT('Ctrl Pts',(-0.816981370219958,0.270995606044562,
-0.13043396260248));
#36381=CARTESIAN_POINT('Ctrl Pts',(-0.837797337716894,-0.00673058913073388,
-0.12347798753416));
#36382=CARTESIAN_POINT('Ctrl Pts',(-0.81492145573658,-0.139942643537178,
-0.12));
#36383=CARTESIAN_POINT('Ctrl Pts',(-0.676565692095419,0.457932546695697,
-0.12));
#36384=CARTESIAN_POINT('Ctrl Pts',(-0.715290549838902,0.406460878340127,
-0.12));
#36385=CARTESIAN_POINT('Ctrl Pts',(-0.761722039381187,0.328281076047514,
-0.12));
#36386=CARTESIAN_POINT('Ctrl Pts',(-0.80978086870511,0.169044693082724,
-0.12));
#36387=CARTESIAN_POINT('Ctrl Pts',(-0.820456584566053,0.110526708837256,
-0.12));
#36388=CARTESIAN_POINT('Ctrl Pts',(-0.829018965506486,-0.012510540419889,
-0.12));
#36389=CARTESIAN_POINT('Ctrl Pts',(-0.825768317377141,-0.0767786210857152,
-0.12));
#36390=CARTESIAN_POINT('Ctrl Pts',(-0.81492145573658,-0.139942643537178,
-0.12));
#36391=CARTESIAN_POINT('Origin',(0.23094010767585,0.4,1.6));
#36392=CARTESIAN_POINT('',(0.23094010767585,0.4,1.6));
#36393=CARTESIAN_POINT('',(0.461880215351701,0.,1.6));
#36394=CARTESIAN_POINT('',(0.288675134594813,0.3,1.6));
#36395=CARTESIAN_POINT('',(0.23094010767585,0.4,1.1));
#36396=CARTESIAN_POINT('',(0.23094010767585,0.4,1.6));
#36397=CARTESIAN_POINT('',(0.461880215351701,0.,1.1));
#36398=CARTESIAN_POINT('',(0.461880215351701,0.,1.1));
#36399=CARTESIAN_POINT('',(0.461880215351701,0.,1.6));
#36400=CARTESIAN_POINT('Origin',(-0.23094010767585,0.4,1.6));
#36401=CARTESIAN_POINT('',(-0.23094010767585,0.4,1.6));
#36402=CARTESIAN_POINT('',(-0.115470053837925,0.4,1.6));
#36403=CARTESIAN_POINT('',(-0.23094010767585,0.4,1.1));
#36404=CARTESIAN_POINT('',(-0.23094010767585,0.4,1.6));
#36405=CARTESIAN_POINT('',(0.23094010767585,0.4,1.1));
#36406=CARTESIAN_POINT('Origin',(-0.461880215351701,5.55111512312578E-17,
1.6));
#36407=CARTESIAN_POINT('',(-0.461880215351701,5.6564012731995E-17,1.6));
#36408=CARTESIAN_POINT('',(-0.404145188432738,0.1,1.6));
#36409=CARTESIAN_POINT('',(-0.461880215351701,5.55111512312578E-17,1.1));
#36410=CARTESIAN_POINT('',(-0.461880215351701,5.6564012731995E-17,1.6));
#36411=CARTESIAN_POINT('',(-0.23094010767585,0.4,1.1));
#36412=CARTESIAN_POINT('Origin',(-0.230940107675851,-0.4,1.6));
#36413=CARTESIAN_POINT('',(-0.230940107675851,-0.4,1.6));
#36414=CARTESIAN_POINT('',(-0.288675134594813,-0.3,1.6));
#36415=CARTESIAN_POINT('',(-0.230940107675851,-0.4,1.1));
#36416=CARTESIAN_POINT('',(-0.230940107675851,-0.4,1.6));
#36417=CARTESIAN_POINT('',(-0.461880215351701,5.6564012731995E-17,1.1));
#36418=CARTESIAN_POINT('Origin',(0.23094010767585,-0.4,1.6));
#36419=CARTESIAN_POINT('',(0.23094010767585,-0.4,1.6));
#36420=CARTESIAN_POINT('',(0.115470053837925,-0.4,1.6));
#36421=CARTESIAN_POINT('',(0.23094010767585,-0.4,1.1));
#36422=CARTESIAN_POINT('',(0.23094010767585,-0.4,1.6));
#36423=CARTESIAN_POINT('',(-0.230940107675851,-0.4,1.1));
#36424=CARTESIAN_POINT('Origin',(0.461880215351701,0.,1.6));
#36425=CARTESIAN_POINT('',(0.404145188432738,-0.1,1.6));
#36426=CARTESIAN_POINT('',(0.23094010767585,-0.4,1.1));
#36427=CARTESIAN_POINT('Origin',(0.,0.,1.1));
#36428=CARTESIAN_POINT('Origin',(0.833031364477342,-0.43549827301267,1.54));
#36429=CARTESIAN_POINT('',(0.810450538189109,-0.391369295102443,0.94));
#36430=CARTESIAN_POINT('',(0.810450538189109,-0.391369295102443,1.54));
#36431=CARTESIAN_POINT('',(0.810450538189109,-0.391369295102443,0.795));
#36432=CARTESIAN_POINT('',(0.79021682086085,-0.351827196260567,0.94));
#36433=CARTESIAN_POINT('',(0.833031364477342,-0.43549827301267,0.94));
#36434=CARTESIAN_POINT('',(0.79021682086085,-0.351827196260567,1.54));
#36435=CARTESIAN_POINT('',(0.79021682086085,-0.351827196260567,1.54));
#36436=CARTESIAN_POINT('',(0.833031364477342,-0.43549827301267,1.54));
#36437=CARTESIAN_POINT('Origin',(0.835630945491614,-0.381577998747588,1.54));
#36438=CARTESIAN_POINT('',(0.833141326548458,-0.340404950018469,1.54));
#36439=CARTESIAN_POINT('Origin',(0.,0.,1.54));
#36440=CARTESIAN_POINT('',(0.79021682086085,-0.351827196260567,1.54));
#36441=CARTESIAN_POINT('Origin',(0.79021682086085,-0.351827196260567,1.54));
#36442=CARTESIAN_POINT('',(0.833141326548458,-0.340404950018469,0.94));
#36443=CARTESIAN_POINT('',(0.833141326548458,-0.340404950018469,0.795));
#36444=CARTESIAN_POINT('',(0.79021682086085,-0.351827196260567,0.94));
#36445=CARTESIAN_POINT('Origin',(0.835630945491614,-0.381577998747588,0.94));
#36446=CARTESIAN_POINT('Origin',(0.,0.,0.94));
#36447=CARTESIAN_POINT('Origin',(0.583878913461612,-0.736671849886289,1.54));
#36448=CARTESIAN_POINT('',(0.581199174513752,-0.687173573083638,0.94));
#36449=CARTESIAN_POINT('',(0.581199174513752,-0.687173573083638,1.54));
#36450=CARTESIAN_POINT('',(0.581199174513752,-0.687173573083638,0.795));
#36451=CARTESIAN_POINT('',(0.578797974500412,-0.642820274037946,0.94));
#36452=CARTESIAN_POINT('',(0.583878913461612,-0.736671849886289,0.94));
#36453=CARTESIAN_POINT('',(0.578797974500412,-0.642820274037946,1.54));
#36454=CARTESIAN_POINT('',(0.578797974500412,-0.642820274037946,1.54));
#36455=CARTESIAN_POINT('',(0.583878913461612,-0.736671849886289,1.54));
#36456=CARTESIAN_POINT('Origin',(0.625201146677623,-0.689746061962118,1.54));
#36457=CARTESIAN_POINT('',(0.622657307785777,-0.649844502216468,1.54));
#36458=CARTESIAN_POINT('Origin',(0.,0.,1.54));
#36459=CARTESIAN_POINT('',(0.578797974500412,-0.642820274037946,1.54));
#36460=CARTESIAN_POINT('Origin',(0.578797974500412,-0.642820274037946,1.54));
#36461=CARTESIAN_POINT('',(0.622657307785777,-0.649844502216468,0.94));
#36462=CARTESIAN_POINT('',(0.622657307785776,-0.649844502216468,0.795));
#36463=CARTESIAN_POINT('',(0.578797974500412,-0.642820274037946,0.94));
#36464=CARTESIAN_POINT('Origin',(0.625201146677623,-0.689746061962118,0.94));
#36465=CARTESIAN_POINT('Origin',(0.,0.,0.94));
#36466=CARTESIAN_POINT('Origin',(0.233768493934963,-0.910468171460913,1.54));
#36467=CARTESIAN_POINT('',(0.251453193536225,-0.864159297502743,0.94));
#36468=CARTESIAN_POINT('',(0.251453193536225,-0.864159297502743,1.54));
#36469=CARTESIAN_POINT('',(0.251453193536225,-0.864159297502743,0.795));
#36470=CARTESIAN_POINT('',(0.267299700134329,-0.822663886595308,0.94));
#36471=CARTESIAN_POINT('',(0.233768493934963,-0.910468171460913,0.94));
#36472=CARTESIAN_POINT('',(0.267299700134329,-0.822663886595308,1.54));
#36473=CARTESIAN_POINT('',(0.267299700134329,-0.822663886595308,1.54));
#36474=CARTESIAN_POINT('',(0.233768493934963,-0.910468171460913,1.54));
#36475=CARTESIAN_POINT('Origin',(0.28990278672928,-0.866566029028111,1.54));
#36476=CARTESIAN_POINT('',(0.304510183842877,-0.846920036329273,1.54));
#36477=CARTESIAN_POINT('Origin',(0.,0.,1.54));
#36478=CARTESIAN_POINT('',(0.267299700134329,-0.822663886595308,1.54));
#36479=CARTESIAN_POINT('Origin',(0.267299700134329,-0.822663886595308,1.54));
#36480=CARTESIAN_POINT('',(0.304510183842877,-0.846920036329273,0.94));
#36481=CARTESIAN_POINT('',(0.304510183842877,-0.846920036329273,0.795));
#36482=CARTESIAN_POINT('',(0.267299700134329,-0.822663886595308,0.94));
#36483=CARTESIAN_POINT('Origin',(0.28990278672928,-0.866566029028111,0.94));
#36484=CARTESIAN_POINT('Origin',(0.,0.,0.94));
#36485=CARTESIAN_POINT('Origin',(-0.156762621913137,-0.926836274846275,
1.54));
#36486=CARTESIAN_POINT('',(-0.121771328984263,-0.891724028742865,0.94));
#36487=CARTESIAN_POINT('',(-0.121771328984263,-0.891724028742865,1.54));
#36488=CARTESIAN_POINT('',(-0.121771328984263,-0.891724028742865,0.795));
#36489=CARTESIAN_POINT('',(-0.0904171207265202,-0.860261439493557,0.94));
#36490=CARTESIAN_POINT('',(-0.156762621913137,-0.926836274846275,0.94));
#36491=CARTESIAN_POINT('',(-0.0904171207265202,-0.860261439493557,1.54));
#36492=CARTESIAN_POINT('',(-0.0904171207265202,-0.860261439493557,1.54));
#36493=CARTESIAN_POINT('',(-0.156762621913137,-0.926836274846275,1.54));
#36494=CARTESIAN_POINT('Origin',(-0.0980628682092918,-0.899718449893242,
1.54));
#36495=CARTESIAN_POINT('',(-0.0662895172746297,-0.897555402133761,1.54));
#36496=CARTESIAN_POINT('Origin',(0.,0.,1.54));
#36497=CARTESIAN_POINT('',(-0.0904171207265202,-0.860261439493557,1.54));
#36498=CARTESIAN_POINT('Origin',(-0.0904171207265202,-0.860261439493557,
1.54));
#36499=CARTESIAN_POINT('',(-0.0662895172746297,-0.897555402133761,0.94));
#36500=CARTESIAN_POINT('',(-0.0662895172746297,-0.897555402133761,0.795));
#36501=CARTESIAN_POINT('',(-0.0904171207265202,-0.860261439493557,0.94));
#36502=CARTESIAN_POINT('Origin',(-0.0980628682092918,-0.899718449893242,
0.94));
#36503=CARTESIAN_POINT('Origin',(0.,0.,0.94));
#36504=CARTESIAN_POINT('Origin',(-0.520188056288743,-0.782945966267494,
1.54));
#36505=CARTESIAN_POINT('',(-0.473940482465577,-0.765101574354867,0.94));
#36506=CARTESIAN_POINT('',(-0.473940482465577,-0.765101574354867,1.54));
#36507=CARTESIAN_POINT('',(-0.473940482465577,-0.765101574354867,0.795));
#36508=CARTESIAN_POINT('',(-0.4325,-0.749111974273539,0.94));
#36509=CARTESIAN_POINT('',(-0.520188056288743,-0.782945966267494,0.94));
#36510=CARTESIAN_POINT('',(-0.4325,-0.749111974273539,1.54));
#36511=CARTESIAN_POINT('',(-0.4325,-0.749111974273539,1.54));
#36512=CARTESIAN_POINT('',(-0.520188056288743,-0.782945966267494,1.54));
#36513=CARTESIAN_POINT('Origin',(-0.469072562361288,-0.795540514449294,
1.54));
#36514=CARTESIAN_POINT('',(-0.425627158633995,-0.792995284874477,1.54));
#36515=CARTESIAN_POINT('Origin',(0.,0.,1.54));
#36516=CARTESIAN_POINT('',(-0.4325,-0.749111974273539,1.54));
#36517=CARTESIAN_POINT('Origin',(-0.4325,-0.749111974273539,1.54));
#36518=CARTESIAN_POINT('',(-0.425627158633995,-0.792995284874477,0.94));
#36519=CARTESIAN_POINT('',(-0.425627158633995,-0.792995284874477,0.795));
#36520=CARTESIAN_POINT('',(-0.4325,-0.749111974273539,0.94));
#36521=CARTESIAN_POINT('Origin',(-0.469072562361288,-0.795540514449294,
0.94));
#36522=CARTESIAN_POINT('Origin',(0.,0.,0.94));
#36523=CARTESIAN_POINT('Origin',(-0.793668249971894,-0.503677187280257,
1.54));
#36524=CARTESIAN_POINT('',(-0.744161020914479,-0.506186107031317,0.94));
#36525=CARTESIAN_POINT('',(-0.744161020914479,-0.506186107031317,1.54));
#36526=CARTESIAN_POINT('',(-0.744161020914479,-0.506186107031317,0.795));
#36527=CARTESIAN_POINT('',(-0.69979970013433,-0.508434243232989,0.94));
#36528=CARTESIAN_POINT('',(-0.793668249971894,-0.503677187280257,0.94));
#36529=CARTESIAN_POINT('',(-0.69979970013433,-0.508434243232989,1.54));
#36530=CARTESIAN_POINT('',(-0.69979970013433,-0.508434243232989,1.54));
#36531=CARTESIAN_POINT('',(-0.793668249971894,-0.503677187280257,1.54));
#36532=CARTESIAN_POINT('Origin',(-0.746733975053112,-0.551427868822013,
1.54));
#36533=CARTESIAN_POINT('',(-0.711369997564195,-0.551319078724396,1.54));
#36534=CARTESIAN_POINT('Origin',(0.,0.,1.54));
#36535=CARTESIAN_POINT('',(-0.69979970013433,-0.508434243232989,1.54));
#36536=CARTESIAN_POINT('Origin',(-0.69979970013433,-0.508434243232989,1.54));
#36537=CARTESIAN_POINT('',(-0.711369997564195,-0.551319078724396,0.94));
#36538=CARTESIAN_POINT('',(-0.711369997564195,-0.551319078724396,0.795));
#36539=CARTESIAN_POINT('',(-0.69979970013433,-0.508434243232989,0.94));
#36540=CARTESIAN_POINT('Origin',(-0.746733975053112,-0.551427868822013,
0.94));
#36541=CARTESIAN_POINT('Origin',(0.,0.,0.94));
#36542=CARTESIAN_POINT('Origin',(-0.929915992985209,-0.137318046848667,
1.54));
#36543=CARTESIAN_POINT('',(-0.885709358356629,-0.159746463245636,0.94));
#36544=CARTESIAN_POINT('',(-0.885709358356629,-0.159746463245636,1.54));
#36545=CARTESIAN_POINT('',(-0.885709358356629,-0.159746463245636,0.795));
#36546=CARTESIAN_POINT('',(-0.846097674634742,-0.179843612557362,0.94));
#36547=CARTESIAN_POINT('',(-0.929915992985209,-0.137318046848667,0.94));
#36548=CARTESIAN_POINT('',(-0.846097674634742,-0.179843612557362,1.54));
#36549=CARTESIAN_POINT('',(-0.846097674634742,-0.179843612557362,1.54));
#36550=CARTESIAN_POINT('',(-0.929915992985209,-0.137318046848667,1.54));
#36551=CARTESIAN_POINT('Origin',(-0.888006833809975,-0.195051339113508,
1.54));
#36552=CARTESIAN_POINT('',(-0.874110501322002,-0.214314795286275,1.54));
#36553=CARTESIAN_POINT('Origin',(0.,0.,1.54));
#36554=CARTESIAN_POINT('',(-0.846097674634742,-0.179843612557362,1.54));
#36555=CARTESIAN_POINT('Origin',(-0.846097674634742,-0.179843612557362,
1.54));
#36556=CARTESIAN_POINT('',(-0.874110501322002,-0.214314795286275,0.94));
#36557=CARTESIAN_POINT('',(-0.874110501322002,-0.214314795286275,0.795));
#36558=CARTESIAN_POINT('',(-0.846097674634742,-0.179843612557362,0.94));
#36559=CARTESIAN_POINT('Origin',(-0.888006833809975,-0.195051339113508,
0.94));
#36560=CARTESIAN_POINT('Origin',(0.,0.,0.94));
#36561=CARTESIAN_POINT('Origin',(0.901572562361288,0.,1.54));
#36562=CARTESIAN_POINT('',(0.899567641099572,-0.0278937105196098,1.54));
#36563=CARTESIAN_POINT('',(0.899567641099572,0.0278937105196097,1.54));
#36564=CARTESIAN_POINT('Origin',(0.,0.,1.54));
#36565=CARTESIAN_POINT('',(0.865,0.,1.54));
#36566=CARTESIAN_POINT('',(0.938145124722575,-0.0590230883575546,1.54));
#36567=CARTESIAN_POINT('',(0.865,0.,1.54));
#36568=CARTESIAN_POINT('Origin',(0.938145124722575,-0.0590230883575546,
1.54));
#36569=CARTESIAN_POINT('',(0.899567641099572,-0.0278937105196098,0.94));
#36570=CARTESIAN_POINT('',(0.899567641099572,-0.0278937105196099,0.795));
#36571=CARTESIAN_POINT('',(0.865,0.,0.94));
#36572=CARTESIAN_POINT('',(0.938145124722575,-0.0590230883575546,0.94));
#36573=CARTESIAN_POINT('',(0.865,0.,1.54));
#36574=CARTESIAN_POINT('Origin',(0.865,0.,1.54));
#36575=CARTESIAN_POINT('',(0.899567641099572,0.0278937105196097,0.94));
#36576=CARTESIAN_POINT('',(0.899567641099572,0.0278937105196099,0.795));
#36577=CARTESIAN_POINT('',(0.865,0.,0.94));
#36578=CARTESIAN_POINT('Origin',(0.901572562361288,0.,0.94));
#36579=CARTESIAN_POINT('Origin',(0.,0.,0.94));
#36580=CARTESIAN_POINT('Origin',(-0.833031364477342,0.43549827301267,1.54));
#36581=CARTESIAN_POINT('',(-0.810450538189109,0.391369295102443,0.94));
#36582=CARTESIAN_POINT('',(-0.810450538189109,0.391369295102443,1.54));
#36583=CARTESIAN_POINT('',(-0.810450538189109,0.391369295102443,0.795));
#36584=CARTESIAN_POINT('',(-0.79021682086085,0.351827196260567,0.94));
#36585=CARTESIAN_POINT('',(-0.833031364477342,0.43549827301267,0.94));
#36586=CARTESIAN_POINT('',(-0.79021682086085,0.351827196260567,1.54));
#36587=CARTESIAN_POINT('',(-0.79021682086085,0.351827196260567,1.54));
#36588=CARTESIAN_POINT('',(-0.833031364477342,0.43549827301267,1.54));
#36589=CARTESIAN_POINT('Origin',(-0.835630945491614,0.381577998747588,1.54));
#36590=CARTESIAN_POINT('',(-0.833141326548458,0.340404950018469,1.54));
#36591=CARTESIAN_POINT('Origin',(0.,0.,1.54));
#36592=CARTESIAN_POINT('',(-0.79021682086085,0.351827196260567,1.54));
#36593=CARTESIAN_POINT('Origin',(-0.79021682086085,0.351827196260567,1.54));
#36594=CARTESIAN_POINT('',(-0.833141326548458,0.340404950018469,0.94));
#36595=CARTESIAN_POINT('',(-0.833141326548458,0.340404950018469,0.795));
#36596=CARTESIAN_POINT('',(-0.79021682086085,0.351827196260567,0.94));
#36597=CARTESIAN_POINT('Origin',(-0.835630945491614,0.381577998747588,0.94));
#36598=CARTESIAN_POINT('Origin',(0.,0.,0.94));
#36599=CARTESIAN_POINT('Origin',(-0.583878913461612,0.736671849886289,1.54));
#36600=CARTESIAN_POINT('',(-0.581199174513752,0.687173573083638,0.94));
#36601=CARTESIAN_POINT('',(-0.581199174513752,0.687173573083638,1.54));
#36602=CARTESIAN_POINT('',(-0.581199174513752,0.687173573083638,0.795));
#36603=CARTESIAN_POINT('',(-0.578797974500412,0.642820274037946,0.94));
#36604=CARTESIAN_POINT('',(-0.583878913461612,0.736671849886289,0.94));
#36605=CARTESIAN_POINT('',(-0.578797974500412,0.642820274037946,1.54));
#36606=CARTESIAN_POINT('',(-0.578797974500412,0.642820274037946,1.54));
#36607=CARTESIAN_POINT('',(-0.583878913461612,0.736671849886289,1.54));
#36608=CARTESIAN_POINT('Origin',(-0.625201146677624,0.689746061962118,1.54));
#36609=CARTESIAN_POINT('',(-0.622657307785776,0.649844502216468,1.54));
#36610=CARTESIAN_POINT('Origin',(0.,0.,1.54));
#36611=CARTESIAN_POINT('',(-0.578797974500412,0.642820274037946,1.54));
#36612=CARTESIAN_POINT('Origin',(-0.578797974500412,0.642820274037946,1.54));
#36613=CARTESIAN_POINT('',(-0.622657307785776,0.649844502216468,0.94));
#36614=CARTESIAN_POINT('',(-0.622657307785776,0.649844502216468,0.795));
#36615=CARTESIAN_POINT('',(-0.578797974500412,0.642820274037946,0.94));
#36616=CARTESIAN_POINT('Origin',(-0.625201146677624,0.689746061962118,0.94));
#36617=CARTESIAN_POINT('Origin',(0.,0.,0.94));
#36618=CARTESIAN_POINT('Origin',(-0.233768493934964,0.910468171460913,1.54));
#36619=CARTESIAN_POINT('',(-0.251453193536226,0.864159297502743,0.94));
#36620=CARTESIAN_POINT('',(-0.251453193536226,0.864159297502743,1.54));
#36621=CARTESIAN_POINT('',(-0.251453193536226,0.864159297502743,0.795));
#36622=CARTESIAN_POINT('',(-0.267299700134329,0.822663886595308,0.94));
#36623=CARTESIAN_POINT('',(-0.233768493934964,0.910468171460913,0.94));
#36624=CARTESIAN_POINT('',(-0.267299700134329,0.822663886595308,1.54));
#36625=CARTESIAN_POINT('',(-0.267299700134329,0.822663886595308,1.54));
#36626=CARTESIAN_POINT('',(-0.233768493934964,0.910468171460913,1.54));
#36627=CARTESIAN_POINT('Origin',(-0.28990278672928,0.866566029028111,1.54));
#36628=CARTESIAN_POINT('',(-0.304510183842877,0.846920036329273,1.54));
#36629=CARTESIAN_POINT('Origin',(0.,0.,1.54));
#36630=CARTESIAN_POINT('',(-0.267299700134329,0.822663886595308,1.54));
#36631=CARTESIAN_POINT('Origin',(-0.267299700134329,0.822663886595308,1.54));
#36632=CARTESIAN_POINT('',(-0.304510183842877,0.846920036329273,0.94));
#36633=CARTESIAN_POINT('',(-0.304510183842877,0.846920036329273,0.795));
#36634=CARTESIAN_POINT('',(-0.267299700134329,0.822663886595308,0.94));
#36635=CARTESIAN_POINT('Origin',(-0.28990278672928,0.866566029028111,0.94));
#36636=CARTESIAN_POINT('Origin',(0.,0.,0.94));
#36637=CARTESIAN_POINT('Origin',(0.156762621913136,0.926836274846275,1.54));
#36638=CARTESIAN_POINT('',(0.121771328984262,0.891724028742865,0.94));
#36639=CARTESIAN_POINT('',(0.121771328984262,0.891724028742865,1.54));
#36640=CARTESIAN_POINT('',(0.121771328984263,0.891724028742865,0.795));
#36641=CARTESIAN_POINT('',(0.0904171207265202,0.860261439493556,0.94));
#36642=CARTESIAN_POINT('',(0.156762621913136,0.926836274846275,0.94));
#36643=CARTESIAN_POINT('',(0.0904171207265202,0.860261439493556,1.54));
#36644=CARTESIAN_POINT('',(0.0904171207265202,0.860261439493556,1.54));
#36645=CARTESIAN_POINT('',(0.156762621913136,0.926836274846275,1.54));
#36646=CARTESIAN_POINT('Origin',(0.0980628682092919,0.899718449893242,1.54));
#36647=CARTESIAN_POINT('',(0.0662895172746301,0.897555402133761,1.54));
#36648=CARTESIAN_POINT('Origin',(0.,0.,1.54));
#36649=CARTESIAN_POINT('',(0.0904171207265202,0.860261439493556,1.54));
#36650=CARTESIAN_POINT('Origin',(0.0904171207265202,0.860261439493556,1.54));
#36651=CARTESIAN_POINT('',(0.0662895172746301,0.897555402133761,0.94));
#36652=CARTESIAN_POINT('',(0.0662895172746301,0.897555402133761,0.795));
#36653=CARTESIAN_POINT('',(0.0904171207265202,0.860261439493556,0.94));
#36654=CARTESIAN_POINT('Origin',(0.0980628682092919,0.899718449893242,0.94));
#36655=CARTESIAN_POINT('Origin',(0.,0.,0.94));
#36656=CARTESIAN_POINT('Origin',(0.520188056288743,0.782945966267494,1.54));
#36657=CARTESIAN_POINT('',(0.473940482465577,0.765101574354867,0.94));
#36658=CARTESIAN_POINT('',(0.473940482465577,0.765101574354867,1.54));
#36659=CARTESIAN_POINT('',(0.473940482465577,0.765101574354867,0.795));
#36660=CARTESIAN_POINT('',(0.4325,0.749111974273539,0.94));
#36661=CARTESIAN_POINT('',(0.520188056288743,0.782945966267494,0.94));
#36662=CARTESIAN_POINT('',(0.4325,0.749111974273539,1.54));
#36663=CARTESIAN_POINT('',(0.4325,0.749111974273539,1.54));
#36664=CARTESIAN_POINT('',(0.520188056288743,0.782945966267494,1.54));
#36665=CARTESIAN_POINT('Origin',(0.469072562361288,0.795540514449294,1.54));
#36666=CARTESIAN_POINT('',(0.425627158633995,0.792995284874477,1.54));
#36667=CARTESIAN_POINT('Origin',(0.,0.,1.54));
#36668=CARTESIAN_POINT('',(0.4325,0.749111974273539,1.54));
#36669=CARTESIAN_POINT('Origin',(0.4325,0.749111974273539,1.54));
#36670=CARTESIAN_POINT('',(0.425627158633995,0.792995284874477,0.94));
#36671=CARTESIAN_POINT('',(0.425627158633995,0.792995284874477,0.795));
#36672=CARTESIAN_POINT('',(0.4325,0.749111974273539,0.94));
#36673=CARTESIAN_POINT('Origin',(0.469072562361288,0.795540514449294,0.94));
#36674=CARTESIAN_POINT('Origin',(0.,0.,0.94));
#36675=CARTESIAN_POINT('Origin',(0.793668249971894,0.503677187280257,1.54));
#36676=CARTESIAN_POINT('',(0.744161020914479,0.506186107031317,0.94));
#36677=CARTESIAN_POINT('',(0.744161020914479,0.506186107031317,1.54));
#36678=CARTESIAN_POINT('',(0.744161020914479,0.506186107031317,0.795));
#36679=CARTESIAN_POINT('',(0.69979970013433,0.508434243232989,0.94));
#36680=CARTESIAN_POINT('',(0.793668249971894,0.503677187280257,0.94));
#36681=CARTESIAN_POINT('',(0.69979970013433,0.508434243232989,1.54));
#36682=CARTESIAN_POINT('',(0.69979970013433,0.508434243232989,1.54));
#36683=CARTESIAN_POINT('',(0.793668249971894,0.503677187280257,1.54));
#36684=CARTESIAN_POINT('Origin',(0.746733975053112,0.551427868822013,1.54));
#36685=CARTESIAN_POINT('',(0.711369997564195,0.551319078724396,1.54));
#36686=CARTESIAN_POINT('Origin',(0.,0.,1.54));
#36687=CARTESIAN_POINT('',(0.69979970013433,0.508434243232989,1.54));
#36688=CARTESIAN_POINT('Origin',(0.69979970013433,0.508434243232989,1.54));
#36689=CARTESIAN_POINT('',(0.711369997564195,0.551319078724396,0.94));
#36690=CARTESIAN_POINT('',(0.711369997564195,0.551319078724396,0.795));
#36691=CARTESIAN_POINT('',(0.69979970013433,0.508434243232989,0.94));
#36692=CARTESIAN_POINT('Origin',(0.746733975053112,0.551427868822013,0.94));
#36693=CARTESIAN_POINT('Origin',(0.,0.,0.94));
#36694=CARTESIAN_POINT('Origin',(0.929915992985209,0.137318046848667,1.54));
#36695=CARTESIAN_POINT('',(0.885709358356629,0.159746463245636,0.94));
#36696=CARTESIAN_POINT('',(0.885709358356629,0.159746463245636,1.54));
#36697=CARTESIAN_POINT('',(0.885709358356629,0.159746463245636,0.795));
#36698=CARTESIAN_POINT('',(0.846097674634742,0.179843612557362,0.94));
#36699=CARTESIAN_POINT('',(0.929915992985209,0.137318046848667,0.94));
#36700=CARTESIAN_POINT('',(0.846097674634742,0.179843612557362,1.54));
#36701=CARTESIAN_POINT('',(0.846097674634742,0.179843612557362,1.54));
#36702=CARTESIAN_POINT('',(0.929915992985209,0.137318046848667,1.54));
#36703=CARTESIAN_POINT('Origin',(0.888006833809975,0.195051339113508,1.54));
#36704=CARTESIAN_POINT('',(0.874110501322002,0.214314795286275,1.54));
#36705=CARTESIAN_POINT('Origin',(0.,0.,1.54));
#36706=CARTESIAN_POINT('',(0.846097674634742,0.179843612557362,1.54));
#36707=CARTESIAN_POINT('Origin',(0.846097674634742,0.179843612557362,1.54));
#36708=CARTESIAN_POINT('',(0.874110501322002,0.214314795286275,0.94));
#36709=CARTESIAN_POINT('',(0.874110501322002,0.214314795286275,0.795));
#36710=CARTESIAN_POINT('',(0.846097674634742,0.179843612557362,0.94));
#36711=CARTESIAN_POINT('Origin',(0.888006833809975,0.195051339113508,0.94));
#36712=CARTESIAN_POINT('Origin',(0.,0.,0.94));
#36713=CARTESIAN_POINT('Origin',(0.881045070122378,0.327657724482506,1.54));
#36714=CARTESIAN_POINT('',(0.833141326548458,0.340404950018469,0.94));
#36715=CARTESIAN_POINT('',(0.833141326548458,0.340404950018469,1.54));
#36716=CARTESIAN_POINT('',(0.833141326548458,0.340404950018469,0.795));
#36717=CARTESIAN_POINT('',(0.79021682086085,0.351827196260567,0.94));
#36718=CARTESIAN_POINT('',(0.881045070122378,0.327657724482506,0.94));
#36719=CARTESIAN_POINT('',(0.79021682086085,0.351827196260567,1.54));
#36720=CARTESIAN_POINT('',(0.79021682086085,0.351827196260567,1.54));
#36721=CARTESIAN_POINT('',(0.881045070122378,0.327657724482506,1.54));
#36722=CARTESIAN_POINT('Origin',(0.835630945491614,0.381577998747588,1.54));
#36723=CARTESIAN_POINT('',(0.810450538189109,0.391369295102443,1.54));
#36724=CARTESIAN_POINT('Origin',(0.,0.,1.54));
#36725=CARTESIAN_POINT('',(0.79021682086085,0.351827196260567,1.54));
#36726=CARTESIAN_POINT('Origin',(0.79021682086085,0.351827196260567,1.54));
#36727=CARTESIAN_POINT('',(0.810450538189109,0.391369295102443,0.94));
#36728=CARTESIAN_POINT('',(0.810450538189109,0.391369295102443,0.795));
#36729=CARTESIAN_POINT('',(0.79021682086085,0.351827196260567,0.94));
#36730=CARTESIAN_POINT('Origin',(0.835630945491614,0.381577998747588,0.94));
#36731=CARTESIAN_POINT('Origin',(0.,0.,0.94));
#36732=CARTESIAN_POINT('Origin',(0.671604318854835,0.657683540082563,1.54));
#36733=CARTESIAN_POINT('',(0.622657307785777,0.649844502216468,0.94));
#36734=CARTESIAN_POINT('',(0.622657307785777,0.649844502216468,1.54));
#36735=CARTESIAN_POINT('',(0.622657307785777,0.649844502216468,0.795));
#36736=CARTESIAN_POINT('',(0.578797974500412,0.642820274037946,0.94));
#36737=CARTESIAN_POINT('',(0.671604318854835,0.657683540082563,0.94));
#36738=CARTESIAN_POINT('',(0.578797974500412,0.642820274037946,1.54));
#36739=CARTESIAN_POINT('',(0.578797974500412,0.642820274037946,1.54));
#36740=CARTESIAN_POINT('',(0.671604318854835,0.657683540082563,1.54));
#36741=CARTESIAN_POINT('Origin',(0.625201146677624,0.689746061962118,1.54));
#36742=CARTESIAN_POINT('',(0.581199174513752,0.687173573083638,1.54));
#36743=CARTESIAN_POINT('Origin',(0.,0.,1.54));
#36744=CARTESIAN_POINT('',(0.578797974500412,0.642820274037946,1.54));
#36745=CARTESIAN_POINT('Origin',(0.578797974500412,0.642820274037946,1.54));
#36746=CARTESIAN_POINT('',(0.581199174513752,0.687173573083638,0.94));
#36747=CARTESIAN_POINT('',(0.581199174513752,0.687173573083638,0.795));
#36748=CARTESIAN_POINT('',(0.578797974500412,0.642820274037946,0.94));
#36749=CARTESIAN_POINT('Origin',(0.625201146677624,0.689746061962118,0.94));
#36750=CARTESIAN_POINT('Origin',(0.,0.,0.94));
#36751=CARTESIAN_POINT('Origin',(0.346037079523597,0.873989896734956,1.54));
#36752=CARTESIAN_POINT('',(0.304510183842877,0.846920036329273,0.94));
#36753=CARTESIAN_POINT('',(0.304510183842877,0.846920036329273,1.54));
#36754=CARTESIAN_POINT('',(0.304510183842877,0.846920036329273,0.795));
#36755=CARTESIAN_POINT('',(0.26729970013433,0.822663886595308,0.94));
#36756=CARTESIAN_POINT('',(0.346037079523597,0.873989896734956,0.94));
#36757=CARTESIAN_POINT('',(0.26729970013433,0.822663886595308,1.54));
#36758=CARTESIAN_POINT('',(0.26729970013433,0.822663886595308,1.54));
#36759=CARTESIAN_POINT('',(0.346037079523597,0.873989896734956,1.54));
#36760=CARTESIAN_POINT('Origin',(0.28990278672928,0.866566029028111,1.54));
#36761=CARTESIAN_POINT('',(0.251453193536226,0.864159297502743,1.54));
#36762=CARTESIAN_POINT('Origin',(0.,0.,1.54));
#36763=CARTESIAN_POINT('',(0.26729970013433,0.822663886595308,1.54));
#36764=CARTESIAN_POINT('Origin',(0.26729970013433,0.822663886595308,1.54));
#36765=CARTESIAN_POINT('',(0.251453193536226,0.864159297502743,0.94));
#36766=CARTESIAN_POINT('',(0.251453193536226,0.864159297502743,0.795));
#36767=CARTESIAN_POINT('',(0.26729970013433,0.822663886595308,0.94));
#36768=CARTESIAN_POINT('Origin',(0.28990278672928,0.866566029028111,0.94));
#36769=CARTESIAN_POINT('Origin',(0.,0.,0.94));
#36770=CARTESIAN_POINT('Origin',(-0.0393631145054476,0.939175460292927,
1.54));
#36771=CARTESIAN_POINT('',(-0.0662895172746301,0.89755540213376,0.94));
#36772=CARTESIAN_POINT('',(-0.0662895172746301,0.89755540213376,1.54));
#36773=CARTESIAN_POINT('',(-0.0662895172746301,0.897555402133761,0.795));
#36774=CARTESIAN_POINT('',(-0.0904171207265203,0.860261439493556,0.94));
#36775=CARTESIAN_POINT('',(-0.0393631145054476,0.939175460292927,0.94));
#36776=CARTESIAN_POINT('',(-0.0904171207265203,0.860261439493556,1.54));
#36777=CARTESIAN_POINT('',(-0.0904171207265203,0.860261439493556,1.54));
#36778=CARTESIAN_POINT('',(-0.0393631145054476,0.939175460292927,1.54));
#36779=CARTESIAN_POINT('Origin',(-0.0980628682092919,0.899718449893242,
1.54));
#36780=CARTESIAN_POINT('',(-0.121771328984263,0.891724028742865,1.54));
#36781=CARTESIAN_POINT('Origin',(0.,0.,1.54));
#36782=CARTESIAN_POINT('',(-0.0904171207265203,0.860261439493556,1.54));
#36783=CARTESIAN_POINT('Origin',(-0.0904171207265203,0.860261439493556,
1.54));
#36784=CARTESIAN_POINT('',(-0.121771328984263,0.891724028742865,0.94));
#36785=CARTESIAN_POINT('',(-0.121771328984263,0.891724028742865,0.795));
#36786=CARTESIAN_POINT('',(-0.0904171207265203,0.860261439493556,0.94));
#36787=CARTESIAN_POINT('Origin',(-0.0980628682092919,0.899718449893242,
0.94));
#36788=CARTESIAN_POINT('Origin',(0.,0.,0.94));
#36789=CARTESIAN_POINT('Origin',(-0.417957068433832,0.841969054625048,1.54));
#36790=CARTESIAN_POINT('',(-0.425627158633995,0.792995284874477,0.94));
#36791=CARTESIAN_POINT('',(-0.425627158633995,0.792995284874477,1.54));
#36792=CARTESIAN_POINT('',(-0.425627158633995,0.792995284874477,0.795));
#36793=CARTESIAN_POINT('',(-0.4325,0.749111974273539,0.94));
#36794=CARTESIAN_POINT('',(-0.417957068433832,0.841969054625048,0.94));
#36795=CARTESIAN_POINT('',(-0.4325,0.749111974273539,1.54));
#36796=CARTESIAN_POINT('',(-0.4325,0.749111974273539,1.54));
#36797=CARTESIAN_POINT('',(-0.417957068433832,0.841969054625048,1.54));
#36798=CARTESIAN_POINT('Origin',(-0.469072562361288,0.795540514449294,1.54));
#36799=CARTESIAN_POINT('',(-0.473940482465577,0.765101574354867,1.54));
#36800=CARTESIAN_POINT('Origin',(0.,0.,1.54));
#36801=CARTESIAN_POINT('',(-0.4325,0.749111974273539,1.54));
#36802=CARTESIAN_POINT('Origin',(-0.4325,0.749111974273539,1.54));
#36803=CARTESIAN_POINT('',(-0.473940482465577,0.765101574354867,0.94));
#36804=CARTESIAN_POINT('',(-0.473940482465577,0.765101574354867,0.795));
#36805=CARTESIAN_POINT('',(-0.4325,0.749111974273539,0.94));
#36806=CARTESIAN_POINT('Origin',(-0.469072562361288,0.795540514449294,0.94));
#36807=CARTESIAN_POINT('Origin',(0.,0.,0.94));
#36808=CARTESIAN_POINT('Origin',(-0.724282448209242,0.599178550363768,1.54));
#36809=CARTESIAN_POINT('',(-0.711369997564195,0.551319078724396,0.94));
#36810=CARTESIAN_POINT('',(-0.711369997564195,0.551319078724396,1.54));
#36811=CARTESIAN_POINT('',(-0.711369997564195,0.551319078724396,0.795));
#36812=CARTESIAN_POINT('',(-0.699799700134329,0.508434243232989,0.94));
#36813=CARTESIAN_POINT('',(-0.724282448209242,0.599178550363768,0.94));
#36814=CARTESIAN_POINT('',(-0.699799700134329,0.508434243232989,1.54));
#36815=CARTESIAN_POINT('',(-0.699799700134329,0.508434243232989,1.54));
#36816=CARTESIAN_POINT('',(-0.724282448209242,0.599178550363768,1.54));
#36817=CARTESIAN_POINT('Origin',(-0.746733975053112,0.551427868822013,1.54));
#36818=CARTESIAN_POINT('',(-0.744161020914479,0.506186107031317,1.54));
#36819=CARTESIAN_POINT('Origin',(0.,0.,1.54));
#36820=CARTESIAN_POINT('',(-0.699799700134329,0.508434243232989,1.54));
#36821=CARTESIAN_POINT('Origin',(-0.699799700134329,0.508434243232989,1.54));
#36822=CARTESIAN_POINT('',(-0.744161020914479,0.506186107031317,0.94));
#36823=CARTESIAN_POINT('',(-0.744161020914479,0.506186107031317,0.795));
#36824=CARTESIAN_POINT('',(-0.699799700134329,0.508434243232989,0.94));
#36825=CARTESIAN_POINT('Origin',(-0.746733975053112,0.551427868822013,0.94));
#36826=CARTESIAN_POINT('Origin',(0.,0.,0.94));
#36827=CARTESIAN_POINT('Origin',(-0.905372812789799,0.25278463137835,1.54));
#36828=CARTESIAN_POINT('',(-0.874110501322002,0.214314795286275,0.94));
#36829=CARTESIAN_POINT('',(-0.874110501322002,0.214314795286275,1.54));
#36830=CARTESIAN_POINT('',(-0.874110501322002,0.214314795286275,0.795));
#36831=CARTESIAN_POINT('',(-0.846097674634742,0.179843612557362,0.94));
#36832=CARTESIAN_POINT('',(-0.905372812789799,0.25278463137835,0.94));
#36833=CARTESIAN_POINT('',(-0.846097674634742,0.179843612557362,1.54));
#36834=CARTESIAN_POINT('',(-0.846097674634742,0.179843612557362,1.54));
#36835=CARTESIAN_POINT('',(-0.905372812789799,0.25278463137835,1.54));
#36836=CARTESIAN_POINT('Origin',(-0.888006833809975,0.195051339113509,1.54));
#36837=CARTESIAN_POINT('',(-0.885709358356629,0.159746463245636,1.54));
#36838=CARTESIAN_POINT('Origin',(0.,0.,1.54));
#36839=CARTESIAN_POINT('',(-0.846097674634742,0.179843612557362,1.54));
#36840=CARTESIAN_POINT('Origin',(-0.846097674634742,0.179843612557362,1.54));
#36841=CARTESIAN_POINT('',(-0.885709358356629,0.159746463245636,0.94));
#36842=CARTESIAN_POINT('',(-0.885709358356629,0.159746463245636,0.795));
#36843=CARTESIAN_POINT('',(-0.846097674634742,0.179843612557362,0.94));
#36844=CARTESIAN_POINT('Origin',(-0.888006833809975,0.195051339113509,0.94));
#36845=CARTESIAN_POINT('Origin',(0.,0.,0.94));
#36846=CARTESIAN_POINT('Origin',(-0.938145124722575,0.0590230883575544,
1.54));
#36847=CARTESIAN_POINT('',(-0.899567641099572,0.0278937105196099,0.94));
#36848=CARTESIAN_POINT('',(-0.899567641099572,0.0278937105196099,1.54));
#36849=CARTESIAN_POINT('',(-0.899567641099572,0.0278937105196097,0.795));
#36850=CARTESIAN_POINT('',(-0.865,1.05931948126246E-16,0.94));
#36851=CARTESIAN_POINT('',(-0.938145124722575,0.0590230883575544,0.94));
#36852=CARTESIAN_POINT('',(-0.865,1.05931948126246E-16,1.54));
#36853=CARTESIAN_POINT('',(-0.865,1.05931948126246E-16,1.54));
#36854=CARTESIAN_POINT('',(-0.938145124722575,0.0590230883575544,1.54));
#36855=CARTESIAN_POINT('Origin',(-0.901572562361288,-9.71445146547012E-17,
1.54));
#36856=CARTESIAN_POINT('',(-0.9,-1.10218211923262E-16,1.54));
#36857=CARTESIAN_POINT('Origin',(0.,0.,1.54));
#36858=CARTESIAN_POINT('',(-0.899567641099572,-0.0278937105196098,1.54));
#36859=CARTESIAN_POINT('',(-0.865,1.05931948126246E-16,1.54));
#36860=CARTESIAN_POINT('Origin',(0.,0.,1.54));
#36861=CARTESIAN_POINT('Origin',(-0.865,1.05931948126246E-16,1.54));
#36862=CARTESIAN_POINT('',(-0.899567641099572,-0.0278937105196098,0.94));
#36863=CARTESIAN_POINT('',(-0.899567641099572,-0.0278937105196098,0.795));
#36864=CARTESIAN_POINT('',(-0.865,1.05931948126246E-16,0.94));
#36865=CARTESIAN_POINT('Origin',(-0.901572562361288,-9.71445146547012E-17,
0.94));
#36866=CARTESIAN_POINT('',(-0.9,-1.10218211923262E-16,0.94));
#36867=CARTESIAN_POINT('Origin',(0.,0.,0.94));
#36868=CARTESIAN_POINT('Origin',(0.,0.,0.94));
#36869=CARTESIAN_POINT('Origin',(-0.881045070122378,-0.327657724482506,
1.54));
#36870=CARTESIAN_POINT('',(-0.833141326548458,-0.340404950018469,0.94));
#36871=CARTESIAN_POINT('',(-0.833141326548458,-0.340404950018469,1.54));
#36872=CARTESIAN_POINT('',(-0.833141326548458,-0.340404950018469,0.795));
#36873=CARTESIAN_POINT('',(-0.79021682086085,-0.351827196260567,0.94));
#36874=CARTESIAN_POINT('',(-0.881045070122378,-0.327657724482506,0.94));
#36875=CARTESIAN_POINT('',(-0.79021682086085,-0.351827196260567,1.54));
#36876=CARTESIAN_POINT('',(-0.79021682086085,-0.351827196260567,1.54));
#36877=CARTESIAN_POINT('',(-0.881045070122378,-0.327657724482506,1.54));
#36878=CARTESIAN_POINT('Origin',(-0.835630945491614,-0.381577998747588,
1.54));
#36879=CARTESIAN_POINT('',(-0.810450538189109,-0.391369295102443,1.54));
#36880=CARTESIAN_POINT('Origin',(0.,0.,1.54));
#36881=CARTESIAN_POINT('',(-0.79021682086085,-0.351827196260567,1.54));
#36882=CARTESIAN_POINT('Origin',(-0.79021682086085,-0.351827196260567,1.54));
#36883=CARTESIAN_POINT('',(-0.810450538189109,-0.391369295102443,0.94));
#36884=CARTESIAN_POINT('',(-0.810450538189109,-0.391369295102443,0.795));
#36885=CARTESIAN_POINT('',(-0.79021682086085,-0.351827196260567,0.94));
#36886=CARTESIAN_POINT('Origin',(-0.835630945491614,-0.381577998747588,
0.94));
#36887=CARTESIAN_POINT('Origin',(0.,0.,0.94));
#36888=CARTESIAN_POINT('Origin',(-0.671604318854835,-0.657683540082563,
1.54));
#36889=CARTESIAN_POINT('',(-0.622657307785777,-0.649844502216468,0.94));
#36890=CARTESIAN_POINT('',(-0.622657307785777,-0.649844502216468,1.54));
#36891=CARTESIAN_POINT('',(-0.622657307785777,-0.649844502216468,0.795));
#36892=CARTESIAN_POINT('',(-0.578797974500412,-0.642820274037946,0.94));
#36893=CARTESIAN_POINT('',(-0.671604318854835,-0.657683540082563,0.94));
#36894=CARTESIAN_POINT('',(-0.578797974500412,-0.642820274037946,1.54));
#36895=CARTESIAN_POINT('',(-0.578797974500412,-0.642820274037946,1.54));
#36896=CARTESIAN_POINT('',(-0.671604318854835,-0.657683540082563,1.54));
#36897=CARTESIAN_POINT('Origin',(-0.625201146677624,-0.689746061962118,
1.54));
#36898=CARTESIAN_POINT('',(-0.581199174513752,-0.687173573083637,1.54));
#36899=CARTESIAN_POINT('Origin',(0.,0.,1.54));
#36900=CARTESIAN_POINT('',(-0.578797974500412,-0.642820274037946,1.54));
#36901=CARTESIAN_POINT('Origin',(-0.578797974500412,-0.642820274037946,
1.54));
#36902=CARTESIAN_POINT('',(-0.581199174513752,-0.687173573083637,0.94));
#36903=CARTESIAN_POINT('',(-0.581199174513752,-0.687173573083637,0.795));
#36904=CARTESIAN_POINT('',(-0.578797974500412,-0.642820274037946,0.94));
#36905=CARTESIAN_POINT('Origin',(-0.625201146677624,-0.689746061962118,
0.94));
#36906=CARTESIAN_POINT('Origin',(0.,0.,0.94));
#36907=CARTESIAN_POINT('Origin',(-0.346037079523597,-0.873989896734956,
1.54));
#36908=CARTESIAN_POINT('',(-0.304510183842877,-0.846920036329273,0.94));
#36909=CARTESIAN_POINT('',(-0.304510183842877,-0.846920036329273,1.54));
#36910=CARTESIAN_POINT('',(-0.304510183842877,-0.846920036329273,0.795));
#36911=CARTESIAN_POINT('',(-0.26729970013433,-0.822663886595308,0.94));
#36912=CARTESIAN_POINT('',(-0.346037079523597,-0.873989896734956,0.94));
#36913=CARTESIAN_POINT('',(-0.26729970013433,-0.822663886595308,1.54));
#36914=CARTESIAN_POINT('',(-0.26729970013433,-0.822663886595308,1.54));
#36915=CARTESIAN_POINT('',(-0.346037079523597,-0.873989896734956,1.54));
#36916=CARTESIAN_POINT('Origin',(-0.289902786729281,-0.866566029028111,
1.54));
#36917=CARTESIAN_POINT('',(-0.251453193536226,-0.864159297502742,1.54));
#36918=CARTESIAN_POINT('Origin',(0.,0.,1.54));
#36919=CARTESIAN_POINT('',(-0.26729970013433,-0.822663886595308,1.54));
#36920=CARTESIAN_POINT('Origin',(-0.26729970013433,-0.822663886595308,1.54));
#36921=CARTESIAN_POINT('',(-0.251453193536226,-0.864159297502742,0.94));
#36922=CARTESIAN_POINT('',(-0.251453193536226,-0.864159297502743,0.795));
#36923=CARTESIAN_POINT('',(-0.26729970013433,-0.822663886595308,0.94));
#36924=CARTESIAN_POINT('Origin',(-0.289902786729281,-0.866566029028111,
0.94));
#36925=CARTESIAN_POINT('Origin',(0.,0.,0.94));
#36926=CARTESIAN_POINT('Origin',(0.0393631145054475,-0.939175460292927,
1.54));
#36927=CARTESIAN_POINT('',(0.0662895172746297,-0.897555402133761,0.94));
#36928=CARTESIAN_POINT('',(0.0662895172746297,-0.897555402133761,1.54));
#36929=CARTESIAN_POINT('',(0.0662895172746297,-0.897555402133761,0.795));
#36930=CARTESIAN_POINT('',(0.0904171207265198,-0.860261439493557,0.94));
#36931=CARTESIAN_POINT('',(0.0393631145054475,-0.939175460292927,0.94));
#36932=CARTESIAN_POINT('',(0.0904171207265198,-0.860261439493557,1.54));
#36933=CARTESIAN_POINT('',(0.0904171207265198,-0.860261439493557,1.54));
#36934=CARTESIAN_POINT('',(0.0393631145054475,-0.939175460292927,1.54));
#36935=CARTESIAN_POINT('Origin',(0.0980628682092919,-0.899718449893242,
1.54));
#36936=CARTESIAN_POINT('',(0.121771328984262,-0.891724028742865,1.54));
#36937=CARTESIAN_POINT('Origin',(0.,0.,1.54));
#36938=CARTESIAN_POINT('',(0.0904171207265198,-0.860261439493557,1.54));
#36939=CARTESIAN_POINT('Origin',(0.0904171207265198,-0.860261439493557,
1.54));
#36940=CARTESIAN_POINT('',(0.121771328984262,-0.891724028742865,0.94));
#36941=CARTESIAN_POINT('',(0.121771328984262,-0.891724028742865,0.795));
#36942=CARTESIAN_POINT('',(0.0904171207265198,-0.860261439493557,0.94));
#36943=CARTESIAN_POINT('Origin',(0.0980628682092919,-0.899718449893242,
0.94));
#36944=CARTESIAN_POINT('Origin',(0.,0.,0.94));
#36945=CARTESIAN_POINT('Origin',(0.417957068433832,-0.841969054625048,1.54));
#36946=CARTESIAN_POINT('',(0.425627158633994,-0.792995284874477,0.94));
#36947=CARTESIAN_POINT('',(0.425627158633994,-0.792995284874477,1.54));
#36948=CARTESIAN_POINT('',(0.425627158633994,-0.792995284874477,0.795));
#36949=CARTESIAN_POINT('',(0.4325,-0.749111974273539,0.94));
#36950=CARTESIAN_POINT('',(0.417957068433832,-0.841969054625048,0.94));
#36951=CARTESIAN_POINT('',(0.4325,-0.749111974273539,1.54));
#36952=CARTESIAN_POINT('',(0.4325,-0.749111974273539,1.54));
#36953=CARTESIAN_POINT('',(0.417957068433832,-0.841969054625048,1.54));
#36954=CARTESIAN_POINT('Origin',(0.469072562361288,-0.795540514449294,1.54));
#36955=CARTESIAN_POINT('',(0.473940482465578,-0.765101574354867,1.54));
#36956=CARTESIAN_POINT('Origin',(0.,0.,1.54));
#36957=CARTESIAN_POINT('',(0.4325,-0.749111974273539,1.54));
#36958=CARTESIAN_POINT('Origin',(0.4325,-0.749111974273539,1.54));
#36959=CARTESIAN_POINT('',(0.473940482465578,-0.765101574354867,0.94));
#36960=CARTESIAN_POINT('',(0.473940482465578,-0.765101574354867,0.795));
#36961=CARTESIAN_POINT('',(0.4325,-0.749111974273539,0.94));
#36962=CARTESIAN_POINT('Origin',(0.469072562361288,-0.795540514449294,0.94));
#36963=CARTESIAN_POINT('Origin',(0.,0.,0.94));
#36964=CARTESIAN_POINT('Origin',(0.724282448209242,-0.599178550363769,1.54));
#36965=CARTESIAN_POINT('',(0.711369997564195,-0.551319078724397,0.94));
#36966=CARTESIAN_POINT('',(0.711369997564195,-0.551319078724397,1.54));
#36967=CARTESIAN_POINT('',(0.711369997564195,-0.551319078724397,0.795));
#36968=CARTESIAN_POINT('',(0.699799700134329,-0.508434243232989,0.94));
#36969=CARTESIAN_POINT('',(0.724282448209242,-0.599178550363769,0.94));
#36970=CARTESIAN_POINT('',(0.699799700134329,-0.508434243232989,1.54));
#36971=CARTESIAN_POINT('',(0.699799700134329,-0.508434243232989,1.54));
#36972=CARTESIAN_POINT('',(0.724282448209242,-0.599178550363769,1.54));
#36973=CARTESIAN_POINT('Origin',(0.746733975053112,-0.551427868822013,1.54));
#36974=CARTESIAN_POINT('',(0.744161020914479,-0.506186107031317,1.54));
#36975=CARTESIAN_POINT('Origin',(0.,0.,1.54));
#36976=CARTESIAN_POINT('',(0.699799700134329,-0.508434243232989,1.54));
#36977=CARTESIAN_POINT('Origin',(0.699799700134329,-0.508434243232989,1.54));
#36978=CARTESIAN_POINT('',(0.744161020914479,-0.506186107031317,0.94));
#36979=CARTESIAN_POINT('',(0.744161020914479,-0.506186107031317,0.795));
#36980=CARTESIAN_POINT('',(0.699799700134329,-0.508434243232989,0.94));
#36981=CARTESIAN_POINT('Origin',(0.746733975053112,-0.551427868822013,0.94));
#36982=CARTESIAN_POINT('Origin',(0.,0.,0.94));
#36983=CARTESIAN_POINT('Origin',(0.905372812789799,-0.25278463137835,1.54));
#36984=CARTESIAN_POINT('',(0.874110501322002,-0.214314795286275,0.94));
#36985=CARTESIAN_POINT('',(0.874110501322002,-0.214314795286275,1.54));
#36986=CARTESIAN_POINT('',(0.874110501322002,-0.214314795286275,0.795));
#36987=CARTESIAN_POINT('',(0.846097674634742,-0.179843612557362,0.94));
#36988=CARTESIAN_POINT('',(0.905372812789799,-0.25278463137835,0.94));
#36989=CARTESIAN_POINT('',(0.846097674634742,-0.179843612557362,1.54));
#36990=CARTESIAN_POINT('',(0.846097674634742,-0.179843612557362,1.54));
#36991=CARTESIAN_POINT('',(0.905372812789799,-0.25278463137835,1.54));
#36992=CARTESIAN_POINT('Origin',(0.888006833809975,-0.195051339113508,1.54));
#36993=CARTESIAN_POINT('',(0.885709358356629,-0.159746463245636,1.54));
#36994=CARTESIAN_POINT('Origin',(0.,0.,1.54));
#36995=CARTESIAN_POINT('',(0.846097674634742,-0.179843612557362,1.54));
#36996=CARTESIAN_POINT('Origin',(0.846097674634742,-0.179843612557362,1.54));
#36997=CARTESIAN_POINT('',(0.885709358356629,-0.159746463245636,0.94));
#36998=CARTESIAN_POINT('',(0.885709358356629,-0.159746463245636,0.795));
#36999=CARTESIAN_POINT('',(0.846097674634742,-0.179843612557362,0.94));
#37000=CARTESIAN_POINT('Origin',(0.888006833809975,-0.195051339113508,0.94));
#37001=CARTESIAN_POINT('Origin',(0.,0.,0.94));
#37002=CARTESIAN_POINT('Origin',(0.,0.,0.0794349077448279));
#37003=CARTESIAN_POINT('',(-1.045,-1.27975590510898E-16,-6.93889390390723E-17));
#37004=CARTESIAN_POINT('Origin',(0.,0.,0.));
#37005=CARTESIAN_POINT('',(-1.1,-9.25861368525747E-17,0.0317542648054295));
#37006=CARTESIAN_POINT('',(-1.18258529610859,-1.44824929759811E-16,0.0794349077448279));
#37007=CARTESIAN_POINT('',(-1.1,0.635085296108588,0.130002302030174));
#37008=CARTESIAN_POINT('Ctrl Pts',(-1.1,0.635085296108588,0.130002302030174));
#37009=CARTESIAN_POINT('Ctrl Pts',(-1.1,0.294744111674235,0.0317542648054296));
#37010=CARTESIAN_POINT('Ctrl Pts',(-1.1,-5.04611257989404E-17,0.0317542648054295));
#37011=CARTESIAN_POINT('',(7.77755175064932E-17,1.27017059221718,0.130002302030174));
#37012=CARTESIAN_POINT('Ctrl Pts',(7.77755175064932E-17,1.27017059221718,
0.130002302030174));
#37013=CARTESIAN_POINT('Ctrl Pts',(-0.55,0.952627944162882,-0.0533310313031589));
#37014=CARTESIAN_POINT('Ctrl Pts',(-1.1,0.635085296108588,0.130002302030174));
#37015=CARTESIAN_POINT('',(1.1,0.635085296108588,0.130002302030174));
#37016=CARTESIAN_POINT('Ctrl Pts',(1.1,0.635085296108588,0.130002302030174));
#37017=CARTESIAN_POINT('Ctrl Pts',(0.55,0.952627944162882,-0.0533310313031591));
#37018=CARTESIAN_POINT('Ctrl Pts',(7.77755175064932E-17,1.27017059221718,
0.130002302030174));
#37019=CARTESIAN_POINT('',(1.1,-0.635085296108589,0.130002302030174));
#37020=CARTESIAN_POINT('Ctrl Pts',(1.1,-0.635085296108589,0.130002302030174));
#37021=CARTESIAN_POINT('Ctrl Pts',(1.1,-3.33066907387547E-16,-0.0533310313031591));
#37022=CARTESIAN_POINT('Ctrl Pts',(1.1,0.635085296108588,0.130002302030174));
#37023=CARTESIAN_POINT('',(-2.3332655251948E-16,-1.27017059221718,0.130002302030174));
#37024=CARTESIAN_POINT('Ctrl Pts',(-2.3332655251948E-16,-1.27017059221718,
0.130002302030174));
#37025=CARTESIAN_POINT('Ctrl Pts',(0.55,-0.952627944162883,-0.0533310313031587));
#37026=CARTESIAN_POINT('Ctrl Pts',(1.1,-0.635085296108589,0.130002302030174));
#37027=CARTESIAN_POINT('',(-1.1,-0.635085296108588,0.130002302030174));
#37028=CARTESIAN_POINT('Ctrl Pts',(-1.1,-0.635085296108588,0.130002302030174));
#37029=CARTESIAN_POINT('Ctrl Pts',(-0.55,-0.952627944162882,-0.0533310313031589));
#37030=CARTESIAN_POINT('Ctrl Pts',(-2.3332655251948E-16,-1.27017059221718,
0.130002302030174));
#37031=CARTESIAN_POINT('Ctrl Pts',(-1.1,-5.04611257989404E-17,0.0317542648054295));
#37032=CARTESIAN_POINT('Ctrl Pts',(-1.1,-0.294744111674235,0.0317542648054295));
#37033=CARTESIAN_POINT('Ctrl Pts',(-1.1,-0.635085296108588,0.130002302030174));
#37034=CARTESIAN_POINT('Origin',(-2.3332655251948E-16,-1.27017059221718,
0.));
#37035=CARTESIAN_POINT('',(1.1,-0.635085296108589,0.669997697969826));
#37036=CARTESIAN_POINT('',(1.1,-0.635085296108589,0.));
#37037=CARTESIAN_POINT('',(-2.3332655251948E-16,-1.27017059221718,0.669997697969826));
#37038=CARTESIAN_POINT('Ctrl Pts',(1.1,-0.635085296108589,0.669997697969826));
#37039=CARTESIAN_POINT('Ctrl Pts',(0.55,-0.952627944162883,0.853331031303159));
#37040=CARTESIAN_POINT('Ctrl Pts',(-2.3332655251948E-16,-1.27017059221718,
0.669997697969826));
#37041=CARTESIAN_POINT('',(-2.3332655251948E-16,-1.27017059221718,0.));
#37042=CARTESIAN_POINT('Origin',(1.1,-0.635085296108589,0.));
#37043=CARTESIAN_POINT('',(1.1,0.635085296108588,0.669997697969826));
#37044=CARTESIAN_POINT('',(1.1,0.635085296108588,0.));
#37045=CARTESIAN_POINT('Ctrl Pts',(1.1,0.635085296108588,0.669997697969826));
#37046=CARTESIAN_POINT('Ctrl Pts',(1.1,-3.33066907387547E-16,0.853331031303159));
#37047=CARTESIAN_POINT('Ctrl Pts',(1.1,-0.635085296108589,0.669997697969826));
#37048=CARTESIAN_POINT('Origin',(1.1,0.635085296108588,0.));
#37049=CARTESIAN_POINT('',(7.77755175064932E-17,1.27017059221718,0.669997697969826));
#37050=CARTESIAN_POINT('',(7.77755175064932E-17,1.27017059221718,0.));
#37051=CARTESIAN_POINT('Ctrl Pts',(7.77755175064932E-17,1.27017059221718,
0.669997697969826));
#37052=CARTESIAN_POINT('Ctrl Pts',(0.55,0.952627944162882,0.853331031303159));
#37053=CARTESIAN_POINT('Ctrl Pts',(1.1,0.635085296108588,0.669997697969826));
#37054=CARTESIAN_POINT('Origin',(0.,0.,0.720565092255172));
#37055=CARTESIAN_POINT('',(-1.1,0.635085296108588,0.669997697969826));
#37056=CARTESIAN_POINT('Ctrl Pts',(-1.1,0.635085296108588,0.669997697969826));
#37057=CARTESIAN_POINT('Ctrl Pts',(-0.55,0.952627944162882,0.853331031303159));
#37058=CARTESIAN_POINT('Ctrl Pts',(7.77755175064932E-17,1.27017059221718,
0.669997697969826));
#37059=CARTESIAN_POINT('',(-1.1,-1.43047262651515E-16,0.768245735194571));
#37060=CARTESIAN_POINT('Ctrl Pts',(-1.1,-1.51383377396821E-16,0.768245735194571));
#37061=CARTESIAN_POINT('Ctrl Pts',(-1.1,0.294744111674235,0.768245735194571));
#37062=CARTESIAN_POINT('Ctrl Pts',(-1.1,0.635085296108588,0.669997697969826));
#37063=CARTESIAN_POINT('',(-1.045,-1.27975590510898E-16,0.8));
#37064=CARTESIAN_POINT('',(-1.18258529610859,-1.44824929759811E-16,0.720565092255172));
#37065=CARTESIAN_POINT('Origin',(0.,0.,0.8));
#37066=CARTESIAN_POINT('',(-1.1,-0.635085296108588,0.669997697969826));
#37067=CARTESIAN_POINT('Ctrl Pts',(-1.1,-0.635085296108588,0.669997697969826));
#37068=CARTESIAN_POINT('Ctrl Pts',(-1.1,-0.294744111674235,0.76824573519457));
#37069=CARTESIAN_POINT('Ctrl Pts',(-1.1,-1.51383377396821E-16,0.768245735194571));
#37070=CARTESIAN_POINT('Ctrl Pts',(-2.3332655251948E-16,-1.27017059221718,
0.669997697969826));
#37071=CARTESIAN_POINT('Ctrl Pts',(-0.55,-0.952627944162883,0.853331031303159));
#37072=CARTESIAN_POINT('Ctrl Pts',(-1.1,-0.635085296108588,0.669997697969826));
#37073=CARTESIAN_POINT('Origin',(7.77755175064932E-17,1.27017059221718,
0.));
#37074=CARTESIAN_POINT('',(-1.1,0.635085296108588,0.));
#37075=CARTESIAN_POINT('Origin',(0.,0.,0.8));
#37076=CARTESIAN_POINT('',(-0.9,-1.10218211923262E-16,0.8));
#37077=CARTESIAN_POINT('Origin',(0.,0.,0.8));
#37078=CARTESIAN_POINT('Origin',(0.,0.,0.));
#37079=CARTESIAN_POINT('',(-0.7431,9.10035036446398E-17,0.));
#37080=CARTESIAN_POINT('Origin',(0.,0.,0.));
#37081=CARTESIAN_POINT('Origin',(-1.1,-0.635085296108589,0.));
#37082=CARTESIAN_POINT('',(-1.1,-0.635085296108589,0.));
#37083=CARTESIAN_POINT('Origin',(-1.1,0.635085296108588,0.));
#37084=CARTESIAN_POINT('Origin',(0.,0.,-0.925));
#37085=CARTESIAN_POINT('',(-0.3,-3.67394039744206E-17,-1.2));
#37086=CARTESIAN_POINT('Origin',(0.,0.,-1.2));
#37087=CARTESIAN_POINT('',(-0.3,-3.67394039744206E-17,-0.6));
#37088=CARTESIAN_POINT('',(-0.3,-3.67394039744206E-17,-0.925));
#37089=CARTESIAN_POINT('Origin',(0.,0.,-0.6));
#37090=CARTESIAN_POINT('Origin',(0.,0.,-0.6));
#37091=CARTESIAN_POINT('',(0.,0.,-0.4));
#37092=CARTESIAN_POINT('',(-0.3,-3.67394039744206E-17,-0.6));
#37093=CARTESIAN_POINT('Origin',(0.7531,0.,-1.2));
#37094=CARTESIAN_POINT('',(-0.7531,-9.22281504437872E-17,-1.2));
#37095=CARTESIAN_POINT('Origin',(0.,0.,-1.2));
#37096=CARTESIAN_POINT('Origin',(0.,0.,-1.16));
#37097=CARTESIAN_POINT('',(-0.7931,-9.71267376403766E-17,-1.16));
#37098=CARTESIAN_POINT('Origin',(0.7431,0.,-0.12));
#37099=CARTESIAN_POINT('',(-0.7431,-9.10035036446398E-17,-0.12));
#37100=CARTESIAN_POINT('Origin',(0.,0.,-0.12));
#37101=CARTESIAN_POINT('Origin',(0.,0.,-0.0349999999999999));
#37102=CARTESIAN_POINT('',(-0.7431,-9.10035036446398E-17,-0.0349999999999999));
#37103=CARTESIAN_POINT('Origin',(0.,0.,0.795));
#37104=CARTESIAN_POINT('Origin',(0.,0.,1.54));
#37105=CARTESIAN_POINT('Origin',(0.,0.,1.54));
#37106=CARTESIAN_POINT('Origin',(0.,0.,1.54));
#37107=CARTESIAN_POINT('Origin',(0.,0.,1.54));
#37108=CARTESIAN_POINT('Origin',(0.,0.,1.54));
#37109=CARTESIAN_POINT('Origin',(0.,0.,1.54));
#37110=CARTESIAN_POINT('Origin',(0.,0.,1.54));
#37111=CARTESIAN_POINT('Origin',(0.,0.,1.54));
#37112=CARTESIAN_POINT('Origin',(0.,0.,1.54));
#37113=CARTESIAN_POINT('Origin',(0.,0.,1.54));
#37114=CARTESIAN_POINT('Origin',(0.,0.,1.54));
#37115=CARTESIAN_POINT('Origin',(0.,0.,1.54));
#37116=CARTESIAN_POINT('Origin',(0.,0.,1.54));
#37117=CARTESIAN_POINT('',(-0.9,-1.10218211923262E-16,0.795));
#37118=CARTESIAN_POINT('Origin',(0.,0.,1.54));
#37119=CARTESIAN_POINT('Origin',(0.,0.,1.54));
#37120=CARTESIAN_POINT('Origin',(0.,0.,1.54));
#37121=CARTESIAN_POINT('Origin',(0.,0.,1.54));
#37122=CARTESIAN_POINT('Origin',(0.,0.,1.54));
#37123=CARTESIAN_POINT('Origin',(0.,0.,1.54));
#37124=CARTESIAN_POINT('Origin',(0.,0.,1.54));
#37125=CARTESIAN_POINT('Origin',(0.,0.,1.54));
#37126=CARTESIAN_POINT('Origin',(0.,0.,1.54));
#37127=CARTESIAN_POINT('Origin',(0.,0.,1.54));
#37128=CARTESIAN_POINT('Origin',(0.,0.,1.54));
#37129=CARTESIAN_POINT('Origin',(0.,0.,1.54));
#37130=CARTESIAN_POINT('Origin',(0.,0.,1.54));
#37131=CARTESIAN_POINT('Origin',(0.,0.,1.54));
#37132=CARTESIAN_POINT('Origin',(0.,0.,1.54));
#37133=CARTESIAN_POINT('Origin',(0.,0.,1.54));
#37134=CARTESIAN_POINT('Origin',(0.,0.,1.54));
#37135=CARTESIAN_POINT('Origin',(0.,0.,1.57));
#37136=CARTESIAN_POINT('',(-0.84,-1.02870331128378E-16,1.6));
#37137=CARTESIAN_POINT('Origin',(0.,0.,1.6));
#37138=CARTESIAN_POINT('',(-0.87,-1.0654427152582E-16,1.57));
#37139=CARTESIAN_POINT('Origin',(0.,0.,1.6));
#59168=UNCERTAINTY_MEASURE_WITH_UNIT(LENGTH_MEASURE(0.001),#59205,
'DISTANCE_ACCURACY_VALUE',
'Maximum model space distance between geometric entities at asserted c
onnectivities');
#59182=UNCERTAINTY_MEASURE_WITH_UNIT(LENGTH_MEASURE(0.001),#59205,
'DISTANCE_ACCURACY_VALUE',
'Maximum model space distance between geometric entities at asserted c
onnectivities');
#59190=(
GEOMETRIC_REPRESENTATION_CONTEXT(3)
GLOBAL_UNCERTAINTY_ASSIGNED_CONTEXT((#59168))
GLOBAL_UNIT_ASSIGNED_CONTEXT((#59205,#59207,#59208))
REPRESENTATION_CONTEXT('','3D')
);
#59204=(
GEOMETRIC_REPRESENTATION_CONTEXT(3)
GLOBAL_UNCERTAINTY_ASSIGNED_CONTEXT((#59182))
GLOBAL_UNIT_ASSIGNED_CONTEXT((#59205,#59207,#59208))
REPRESENTATION_CONTEXT('','3D')
);
#59205=(
LENGTH_UNIT()
NAMED_UNIT(*)
SI_UNIT(.CENTI.,.METRE.)
);
#59207=(
NAMED_UNIT(*)
PLANE_ANGLE_UNIT()
SI_UNIT($,.RADIAN.)
);
#59208=(
NAMED_UNIT(*)
SI_UNIT($,.STERADIAN.)
SOLID_ANGLE_UNIT()
);
#59216=SHAPE_DEFINITION_REPRESENTATION(#59237,#59303);
#59237=PRODUCT_DEFINITION_SHAPE('',$,#59325);
#59303=SHAPE_REPRESENTATION('',(#23228),#59190);
#59317=PRODUCT_DEFINITION_CONTEXT('part definition',#59382,'design');
#59325=PRODUCT_DEFINITION('2026-10-23-00-47-37-044',
'18_Pressure_Relief_Valve_Plug_G3-8_AF22',#59346,#59317);
#59346=PRODUCT_DEFINITION_FORMATION('',$,#59391);
#59382=APPLICATION_CONTEXT(
'Core Data for Automotive Mechanical Design Process');
#59383=PRODUCT_CONTEXT('part definition',#59382,'mechanical');
#59391=PRODUCT('2026-10-23-00-47-37-044',
'18_Pressure_Relief_Valve_Plug_G3-8_AF22',$,(#59383));
#59566=COLOUR_RGB('Light Blue',0.38,0.62,0.78);
#59567=FILL_AREA_STYLE_COLOUR('',#59566);
#59568=FILL_AREA_STYLE('',(#59567));
#59569=SURFACE_STYLE_FILL_AREA(#59568);
#59570=SURFACE_SIDE_STYLE('',(#59569));
#59571=SURFACE_STYLE_USAGE(.BOTH.,#59570);
#59572=PRESENTATION_STYLE_ASSIGNMENT((#59571));
ENDSEC;
END-ISO-10303-21;
